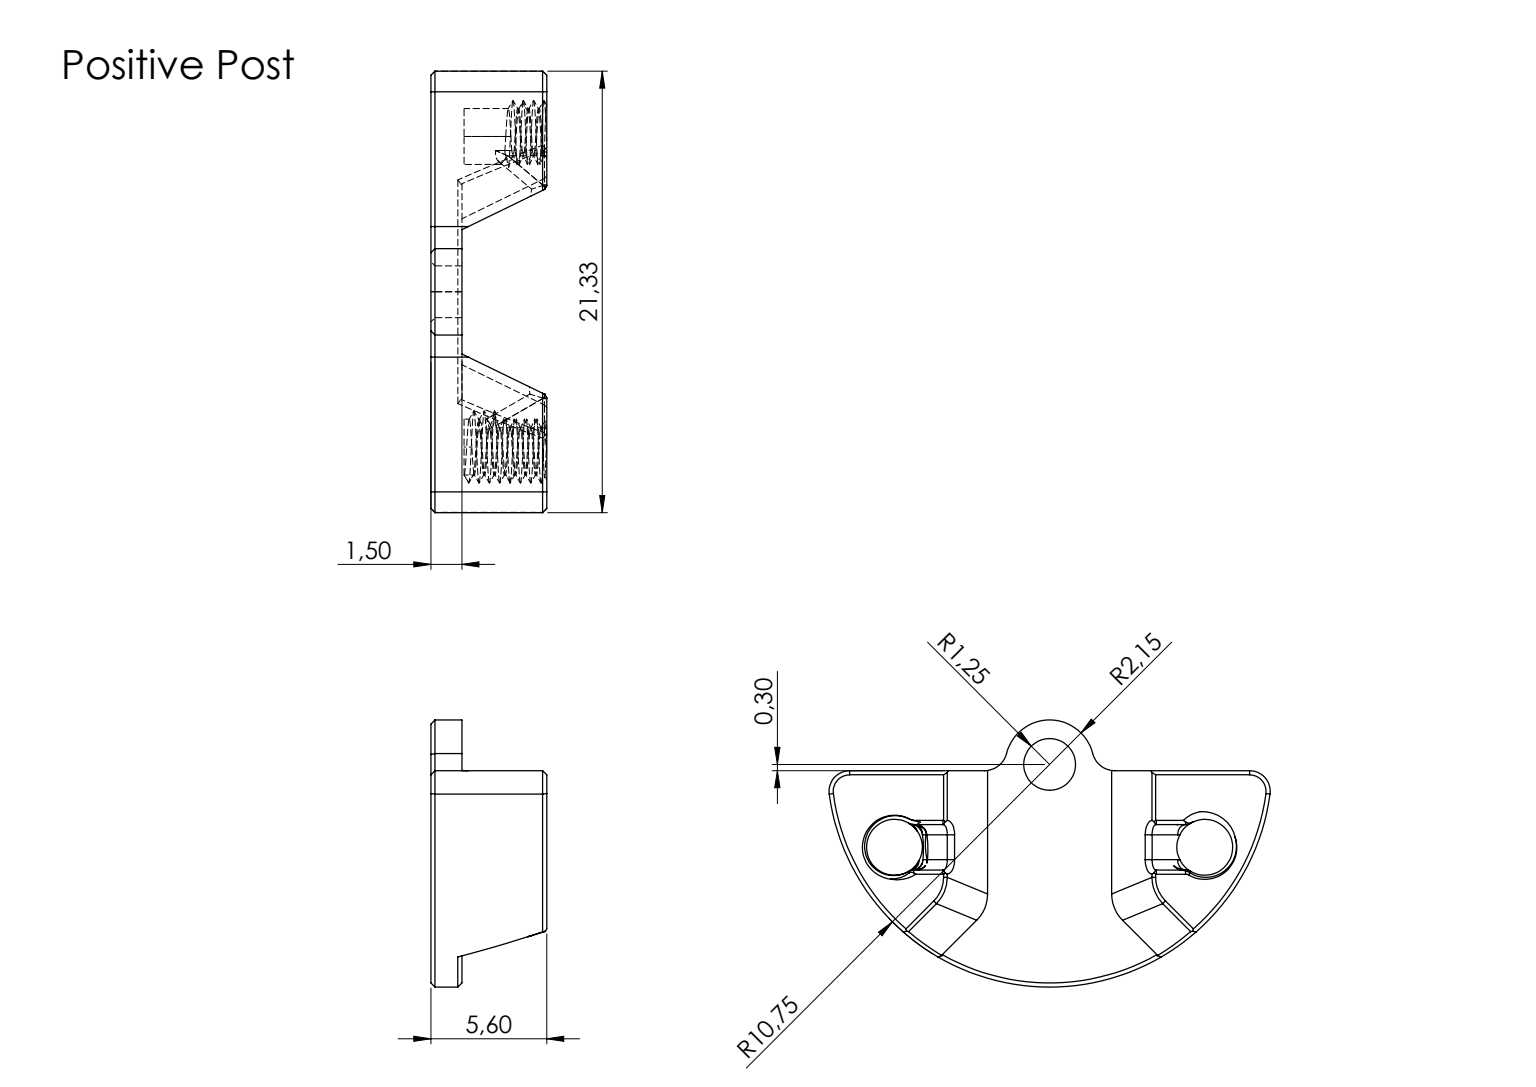
ISO-10303-21;
HEADER;
FILE_DESCRIPTION (('STEP AP214'),
    '1' );
FILE_NAME ('Positive Post.step',
    '2026-10-05T22:38:29',
    ( '' ),
    ( '' ),
    'SwSTEP 2.0',
    'SolidWorks 2020',
    '' );
FILE_SCHEMA (( 'AUTOMOTIVE_DESIGN' ));
ENDSEC;

DATA;
#3=DIRECTION ( 'NONE',  ( 1.000000000000000000, 0.000000000000000000, 0.000000000000000000 ) ) ;
#10=CARTESIAN_POINT ( 'NONE',  ( 9.778462793022999477, -5.743713977826000239, 7.748300060190000060 ) ) ;
#24=B_SPLINE_CURVE_WITH_KNOTS ( 'NONE', 3,
 ( #18393, #12452, #50546, #13155, #61715, #44967, #55102, #35164, #34485, #56132, #66271, #55449, #55796, #8240, #40068, #29927 ),
 .UNSPECIFIED., .F., .F.,
 ( 4, 2, 2, 1, 1, 2, 2, 2, 4 ),
 ( 0.000000000000000000, 0.2499999999999854561, 0.3749999999999792943, 0.4374999999999752420, 0.4687499999999756861, 0.4843749999999741873, 0.4999999999999726885, 0.7499999999999863443, 1.000000000000000000 ),
 .UNSPECIFIED. ) ;
#26=CARTESIAN_POINT ( 'NONE',  ( 9.239023565813489824, -2.669687318136871212, 7.269906695626100479 ) ) ;
#28=ORIENTED_EDGE ( 'NONE', *, *, #52791, .T. ) ;
#57=CARTESIAN_POINT ( 'NONE',  ( 8.674830025576039105, -2.649890579813208191, 7.499988935010342139 ) ) ;
#61=CARTESIAN_POINT ( 'NONE',  ( 9.794101180193951706, -2.685368189354502721, -7.853409369710684373 ) ) ;
#62=CYLINDRICAL_SURFACE ( 'NONE', #7615, 1.350000000000000089 ) ;
#73=EDGE_CURVE ( 'NONE', #54965, #29508, #17176, .T. ) ;
#82=ORIENTED_EDGE ( 'NONE', *, *, #59738, .T. ) ;
#88=CARTESIAN_POINT ( 'NONE',  ( 10.01835931248959888, -5.126777126172243015, -6.752018918849381102 ) ) ;
#100=EDGE_CURVE ( 'NONE', #6210, #57286, #54708, .T. ) ;
#109=CARTESIAN_POINT ( 'NONE',  ( 8.383148997457999130, -5.167567567567999731, 6.822293592207000934 ) ) ;
#113=CARTESIAN_POINT ( 'NONE',  ( 10.36950884864999978, -2.719121019997000399, -7.031782724641000293 ) ) ;
#114=ORIENTED_EDGE ( 'NONE', *, *, #34124, .T. ) ;
#117=CARTESIAN_POINT ( 'NONE',  ( 10.17905590578999941, -2.899999999999999911, 6.571291218949999902 ) ) ;
#118=LINE ( 'NONE', #6737, #27722 ) ;
#119=CARTESIAN_POINT ( 'NONE',  ( 8.635274708161395196, -3.045105040003566632, -6.545565613752198253 ) ) ;
#132=CARTESIAN_POINT ( 'NONE',  ( 7.905017292225999803, -2.916160783733999562, 6.437838678341997856 ) ) ;
#137=CARTESIAN_POINT ( 'NONE',  ( 9.215289122285998502, -4.861979632688999686, 8.938813901364000003 ) ) ;
#150=DIRECTION ( 'NONE',  ( -1.000000000000000000, 0.000000000000000000, 0.000000000000000000 ) ) ;
#157=DIRECTION ( 'NONE',  ( 0.000000000000000000, -0.1333333333333049930, -0.9910712498212376209 ) ) ;
#163=CARTESIAN_POINT ( 'NONE',  ( 10.00122642709000154, -2.274091010763000131, 7.851325450887000734 ) ) ;
#167=CARTESIAN_POINT ( 'NONE',  ( 9.085769353209000698, -2.821866379289000193, 6.127148604720000336 ) ) ;
#168=CARTESIAN_POINT ( 'NONE',  ( 10.32322128467999889, -3.399999874579999748, -4.621083553505000552 ) ) ;
#171=CIRCLE ( 'NONE', #66048, 0.5000000000000000000 ) ;
#176=CARTESIAN_POINT ( 'NONE',  ( 10.84168850528999961, -2.681008214828000114, 6.554752254946000889 ) ) ;
#181=CARTESIAN_POINT ( 'NONE',  ( 10.65229194037999960, -4.944342461481999962, -8.478476072358999360 ) ) ;
#183=CARTESIAN_POINT ( 'NONE',  ( 10.90000000536000080, -2.899999999941999640, -5.157071284930999866 ) ) ;
#191=CARTESIAN_POINT ( 'NONE',  ( 10.98768521492000083, -5.299565686336999981, -4.945211137252000455 ) ) ;
#200=CARTESIAN_POINT ( 'NONE',  ( 8.767881343006999728, -4.605543323398999966, -6.293427432547999523 ) ) ;
#202=CARTESIAN_POINT ( 'NONE',  ( 9.492702081557240490, -3.384517283567192170, -9.168413593352800817 ) ) ;
#208=CARTESIAN_POINT ( 'NONE',  ( 8.464254440379999522, -2.029110377978999846, 7.726994002375999315 ) ) ;
#212=VECTOR ( 'NONE', #46961, 1000.000000000000000 ) ;
#220=CARTESIAN_POINT ( 'NONE',  ( 11.09999999999999964, -6.593648099371000271, -5.598803483715999896 ) ) ;
#222=CARTESIAN_POINT ( 'NONE',  ( 8.764831853209999579, -5.808258301303999893, 7.446016267012000256 ) ) ;
#223=CARTESIAN_POINT ( 'NONE',  ( 8.898558059623999483, -5.146736128384000075, 6.597417125647000447 ) ) ;
#224=EDGE_CURVE ( 'NONE', #15130, #33857, #51488, .T. ) ;
#243=CARTESIAN_POINT ( 'NONE',  ( 8.449835681852293945, -2.260412657429408334, 7.498936987450196767 ) ) ;
#254=CARTESIAN_POINT ( 'NONE',  ( 9.865041550948088656, -2.650034642413194419, -7.500002425457253707 ) ) ;
#276=ORIENTED_EDGE ( 'NONE', *, *, #50855, .T. ) ;
#282=CARTESIAN_POINT ( 'NONE',  ( 10.98768521492000083, -5.299565686336999981, -4.945211137252000455 ) ) ;
#288=LINE ( 'NONE', #16362, #21275 ) ;
#296=ADVANCED_FACE ( 'NONE', ( #16756 ), #38788, .T. ) ;
#299=ORIENTED_EDGE ( 'NONE', *, *, #35075, .F. ) ;
#302=ADVANCED_FACE ( 'NONE', ( #33547 ), #22385, .T. ) ;
#309=AXIS2_PLACEMENT_3D ( 'NONE', #43572, #37285, #64184 ) ;
#320=CARTESIAN_POINT ( 'NONE',  ( 10.64872180584000105, -2.614778238704999591, 6.717279975758000177 ) ) ;
#321=CARTESIAN_POINT ( 'NONE',  ( 7.127706853208000126, -4.698358408974000255, 8.789434435623999065 ) ) ;
#326=CARTESIAN_POINT ( 'NONE',  ( 10.41025564679000048, -4.690690303276999984, -6.142863315966000215 ) ) ;
#327=CARTESIAN_POINT ( 'NONE',  ( 7.869532996850215234, -3.050177706499410668, 8.968124616582409558 ) ) ;
#329=CARTESIAN_POINT ( 'NONE',  ( 10.09196524370999981, -3.841385669346000231, 5.536421174581999338 ) ) ;
#350=CARTESIAN_POINT ( 'NONE',  ( 10.92717634842000152, -5.023656093247000243, 8.718039182945998888 ) ) ;
#357=ORIENTED_EDGE ( 'NONE', *, *, #14220, .T. ) ;
#374=CARTESIAN_POINT ( 'NONE',  ( 10.06844525594999951, -4.148609764890999863, 8.941457795715999524 ) ) ;
#414=CARTESIAN_POINT ( 'NONE',  ( 10.10735564678999943, -4.293585439421999439, -8.994200998147999115 ) ) ;
#436=CARTESIAN_POINT ( 'NONE',  ( 10.52663358771999924, -4.933730002636999679, -6.506004698255999585 ) ) ;
#438=VERTEX_POINT ( 'NONE', #64909 ) ;
#440=ORIENTED_EDGE ( 'NONE', *, *, #23269, .T. ) ;
#448=CARTESIAN_POINT ( 'NONE',  ( 10.29378083128999855, -3.483628580733000302, 6.176326635498999629 ) ) ;
#458=CARTESIAN_POINT ( 'NONE',  ( 10.36629943602999937, -5.852732332139999549, -7.568014220767000033 ) ) ;
#460=ORIENTED_EDGE ( 'NONE', *, *, #48777, .T. ) ;
#473=FACE_OUTER_BOUND ( 'NONE', #7500, .T. ) ;
#478=CARTESIAN_POINT ( 'NONE',  ( 9.318721994369999706, -2.755032632138999737, 8.795122807847999269 ) ) ;
#482=CARTESIAN_POINT ( 'NONE',  ( 9.504901164121001500, -3.934733502342999678, 5.704835336325999151 ) ) ;
#484=CARTESIAN_POINT ( 'NONE',  ( 9.780103651350286142, -2.899999999999999911, -6.453331515098025051 ) ) ;
#485=EDGE_CURVE ( 'NONE', #31101, #42061, #40421, .T. ) ;
#497=DIRECTION ( 'NONE',  ( 0.000000000000000000, -1.000000000000000000, 0.000000000000000000 ) ) ;
#505=ORIENTED_EDGE ( 'NONE', *, *, #36321, .F. ) ;
#507=CARTESIAN_POINT ( 'NONE',  ( 10.18909467608999897, -5.907859813488999912, 7.801539220053999912 ) ) ;
#518=VERTEX_POINT ( 'NONE', #61745 ) ;
#519=CARTESIAN_POINT ( 'NONE',  ( 9.104016254283999743, -5.045864843302999780, 8.527867871227000407 ) ) ;
#525=DIRECTION ( 'NONE',  ( 0.8987684456439055669, 0.000000000000000000, -0.4384236320214022764 ) ) ;
#532=VECTOR ( 'NONE', #65504, 1000.000000000000114 ) ;
#550=CARTESIAN_POINT ( 'NONE',  ( 10.90000000016000037, -2.832432432627000285, -6.822293591557000880 ) ) ;
#553=ORIENTED_EDGE ( 'NONE', *, *, #2355, .F. ) ;
#560=CARTESIAN_POINT ( 'NONE',  ( 7.705394353206999725, -3.245532552444000185, 8.949627348471000943 ) ) ;
#562=CARTESIAN_POINT ( 'NONE',  ( 7.851684996376999237, -4.710033951126000318, 6.351751497389999557 ) ) ;
#564=EDGE_CURVE ( 'NONE', #28902, #67173, #57226, .T. ) ;
#569=CARTESIAN_POINT ( 'NONE',  ( 11.09999999999999787, -5.533462193136272411, 7.009885406647008210 ) ) ;
#572=CARTESIAN_POINT ( 'NONE',  ( 9.406706853206999952, -3.705847642455000202, 9.096432253453999195 ) ) ;
#577=EDGE_CURVE ( 'NONE', #1541, #49491, #24675, .T. ) ;
#578=AXIS2_PLACEMENT_3D ( 'NONE', #48457, #16634, #59282 ) ;
#583=CARTESIAN_POINT ( 'NONE',  ( 9.470944094206000585, -5.100000000000000533, 6.571291218949999902 ) ) ;
#590=CARTESIAN_POINT ( 'NONE',  ( 8.432199894032919474, -2.299073235464944798, 7.876362923782135539 ) ) ;
#597=CARTESIAN_POINT ( 'NONE',  ( 7.732053840042254045, -3.067861470021875814, 6.507875357840980257 ) ) ;
#600=CARTESIAN_POINT ( 'NONE',  ( 10.28566371494471632, -5.375939593780930892, -6.377587382198379728 ) ) ;
#603=CARTESIAN_POINT ( 'NONE',  ( 9.004094043040858253, -2.621318921512024946, 6.376249635427098994 ) ) ;
#606=VERTEX_POINT ( 'NONE', #23655 ) ;
#611=CARTESIAN_POINT ( 'NONE',  ( 9.056630296855326279, -5.100000000000000533, 6.328714934328742103 ) ) ;
#612=ORIENTED_EDGE ( 'NONE', *, *, #21132, .T. ) ;
#616=LINE ( 'NONE', #53412, #60037 ) ;
#633=CARTESIAN_POINT ( 'NONE',  ( 10.25166529434999951, -3.418639857622999934, -8.733652610425998830 ) ) ;
#634=AXIS2_PLACEMENT_3D ( 'NONE', #59823, #28367, #23107 ) ;
#639=CARTESIAN_POINT ( 'NONE',  ( 10.85646369190719973, -5.100000000000000533, 6.665341197380437066 ) ) ;
#649=ORIENTED_EDGE ( 'NONE', *, *, #42532, .T. ) ;
#650=DIRECTION ( 'NONE',  ( 1.000000000000000000, 0.000000000000000000, -1.736057635220000058E-14 ) ) ;
#659=EDGE_CURVE ( 'NONE', #35912, #16031, #57879, .T. ) ;
#660=VECTOR ( 'NONE', #36324, 1000.000000000000000 ) ;
#664=VERTEX_POINT ( 'NONE', #9284 ) ;
#668=CARTESIAN_POINT ( 'NONE',  ( 10.98286725694000054, -3.998514182530999772, 9.091066422484001208 ) ) ;
#669=CARTESIAN_POINT ( 'NONE',  ( 7.833769353207999941, -2.583664704444999849, 6.684748541034000624 ) ) ;
#671=CARTESIAN_POINT ( 'NONE',  ( 8.205992358809998777, -3.399999999999999911, 6.138278517058000538 ) ) ;
#673=CARTESIAN_POINT ( 'NONE',  ( 10.29666814679000097, -2.755511079787000384, -6.622434938646999392 ) ) ;
#674=CARTESIAN_POINT ( 'NONE',  ( 7.771548168530000744, -5.066493862386956870, 8.873801325387214334 ) ) ;
#675=CARTESIAN_POINT ( 'NONE',  ( 10.58844302970999962, -3.754658547780000521, 5.545362468768000319 ) ) ;
#683=VERTEX_POINT ( 'NONE', #46710 ) ;
#691=CARTESIAN_POINT ( 'NONE',  ( 8.946004440379999423, -5.458705123429999695, 7.456451825584000659 ) ) ;
#701=EDGE_CURVE ( 'NONE', #59694, #61758, #40523, .T. ) ;
#705=ADVANCED_FACE ( 'NONE', ( #26415 ), #52981, .T. ) ;
#706=EDGE_CURVE ( 'NONE', #1057, #51230, #41392, .T. ) ;
#723=CARTESIAN_POINT ( 'NONE',  ( 10.31668414895000119, -3.819528725844000494, 6.062183754159999438 ) ) ;
#744=EDGE_CURVE ( 'NONE', #12348, #53120, #12170, .T. ) ;
#751=VECTOR ( 'NONE', #15220, 1000.000000000000000 ) ;
#760=CARTESIAN_POINT ( 'NONE',  ( 10.09249435321000021, -2.841617206345000035, -8.724656239052000828 ) ) ;
#765=DIRECTION ( 'NONE',  ( -0.7660444431190119863, -5.852582307674940185E-12, -0.6427876096864989508 ) ) ;
#766=ORIENTED_EDGE ( 'NONE', *, *, #53572, .F. ) ;
#782=CARTESIAN_POINT ( 'NONE',  ( 10.43283788151999936, -3.279327064383000145, -9.029275888523999427 ) ) ;
#795=CARTESIAN_POINT ( 'NONE',  ( 9.423521818475000700, -4.993993578306000103, 8.578110568283999982 ) ) ;
#808=CARTESIAN_POINT ( 'NONE',  ( 10.19715077290999972, -4.982624057277000418, -6.124316828241999744 ) ) ;
#825=CARTESIAN_POINT ( 'NONE',  ( 10.02990552045999983, -2.506467134554999809, 6.215414506835998942 ) ) ;
#829=CARTESIAN_POINT ( 'NONE',  ( 9.442841440870999747, -2.691258483914000355, 6.269525829285999663 ) ) ;
#844=CARTESIAN_POINT ( 'NONE',  ( 7.610826510211253115, -3.823093646280199653, 8.848653938445639966 ) ) ;
#847=CARTESIAN_POINT ( 'NONE',  ( 5.699999999836000697, -1.433333331105999919, -10.65401593570999950 ) ) ;
#849=CARTESIAN_POINT ( 'NONE',  ( 10.84920446231350155, -2.899999999999999911, -6.662590550579920112 ) ) ;
#852=VERTEX_POINT ( 'NONE', #14552 ) ;
#859=EDGE_LOOP ( 'NONE', ( #2403, #13429, #58338, #59065 ) ) ;
#864=CARTESIAN_POINT ( 'NONE',  ( 9.911640687501567015, -2.873222873816665413, -6.752018918868491149 ) ) ;
#867=CARTESIAN_POINT ( 'NONE',  ( 10.68904248846000016, -2.568964727443000307, 7.728094434513999467 ) ) ;
#870=EDGE_CURVE ( 'NONE', #57810, #22321, #17292, .T. ) ;
#873=VERTEX_POINT ( 'NONE', #6798 ) ;
#886=CARTESIAN_POINT ( 'NONE',  ( 9.327383005933997495, -3.946161398296482048, 9.238824392371451921 ) ) ;
#895=CARTESIAN_POINT ( 'NONE',  ( 9.305875415870998424, -4.945293979885000191, 9.077881967919999795 ) ) ;
#897=CARTESIAN_POINT ( 'NONE',  ( 7.717206996518667594, -2.839603352907888123, 6.809939372030577864 ) ) ;
#899=EDGE_LOOP ( 'NONE', ( #66916, #36286, #32294, #9509 ) ) ;
#900=ORIENTED_EDGE ( 'NONE', *, *, #41275, .F. ) ;
#904=CARTESIAN_POINT ( 'NONE',  ( 9.199609130449999839, -2.551382302226000487, 7.536606162076999738 ) ) ;
#906=CARTESIAN_POINT ( 'NONE',  ( 8.347269353210000631, -2.741638482234999952, 6.457327039244000311 ) ) ;
#915=CARTESIAN_POINT ( 'NONE',  ( 11.07925595036916633, -5.279255950369167394, 6.503434303641999925 ) ) ;
#920=CARTESIAN_POINT ( 'NONE',  ( 8.834370559623998531, -4.141908960411000429, 6.047561724438000219 ) ) ;
#938=CARTESIAN_POINT ( 'NONE',  ( 8.447423826815846581, -2.260942181570626541, 7.552185937853629127 ) ) ;
#948=CARTESIAN_POINT ( 'NONE',  ( 10.77164068750950143, -2.873222873834234914, 6.752018918838221140 ) ) ;
#949=CARTESIAN_POINT ( 'NONE',  ( 11.04783424078000031, -2.764605797469000148, 5.041477660832000218 ) ) ;
#953=EDGE_LOOP ( 'NONE', ( #20511, #17436, #26609 ) ) ;
#956=EDGE_CURVE ( 'NONE', #9091, #38701, #48076, .T. ) ;
#980=CARTESIAN_POINT ( 'NONE',  ( 10.77434462036999818, -4.612888200890999713, -8.898797372219998891 ) ) ;
#985=ORIENTED_EDGE ( 'NONE', *, *, #39002, .F. ) ;
#996=DIRECTION ( 'NONE',  ( -0.7071067811865474617, -0.7071067811865474617, 1.013775886743067205E-08 ) ) ;
#998=FACE_OUTER_BOUND ( 'NONE', #6504, .T. ) ;
#1004=CARTESIAN_POINT ( 'NONE',  ( 10.63789391302397647, -4.829717262113836895, -8.579596796881972409 ) ) ;
#1017=CARTESIAN_POINT ( 'NONE',  ( 10.18239901426000138, -2.607725299334000102, 7.783410967795999724 ) ) ;
#1018=CARTESIAN_POINT ( 'NONE',  ( 8.770183059623999355, -3.049610585291000042, 6.392533570808999421 ) ) ;
#1022=CARTESIAN_POINT ( 'NONE',  ( 11.01605564679000082, -5.482859940357000639, -7.846409404949000077 ) ) ;
#1023=CARTESIAN_POINT ( 'NONE',  ( 7.767789809242127141, -5.129599579532937881, 8.822844411293367273 ) ) ;
#1026=ORIENTED_EDGE ( 'NONE', *, *, #43279, .F. ) ;
#1040=DIRECTION ( 'NONE',  ( -0.7660444431190069903, 0.000000000000000000, -0.6427876096865049460 ) ) ;
#1043=CARTESIAN_POINT ( 'NONE',  ( 9.395316940379000670, -5.146736128384000075, 6.597417125647000447 ) ) ;
#1046=CARTESIAN_POINT ( 'NONE',  ( 10.00068357938802954, -3.239576832587917732, -9.078134629932138822 ) ) ;
#1057=VERTEX_POINT ( 'NONE', #21414 ) ;
#1064=LINE ( 'NONE', #22718, #65137 ) ;
#1072=CARTESIAN_POINT ( 'NONE',  ( 10.13050497920000126, -3.092053006542000215, 8.629388195475000245 ) ) ;
#1083=PLANE ( 'NONE',  #43091 ) ;
#1110=CARTESIAN_POINT ( 'NONE',  ( 10.16821935321000048, -2.330398934821000356, -7.267462182607999921 ) ) ;
#1111=CARTESIAN_POINT ( 'NONE',  ( 11.00000000000000000, -0.4000000000000000222, -7.331472342878999626 ) ) ;
#1114=DIRECTION ( 'NONE',  ( 0.4384236320214023319, 0.000000000000000000, -0.8987684456439056779 ) ) ;
#1117=ORIENTED_EDGE ( 'NONE', *, *, #15075, .T. ) ;
#1128=CARTESIAN_POINT ( 'NONE',  ( 10.98277446826000059, -2.518728855032000169, -8.314788219120000434 ) ) ;
#1132=B_SPLINE_CURVE_WITH_KNOTS ( 'NONE', 3,
 ( #7572, #7229, #2671, #65944 ),
 .UNSPECIFIED., .F., .F.,
 ( 4, 4 ),
 ( 0.000000000000000000, 1.000000000000000000 ),
 .UNSPECIFIED. ) ;
#1133=ORIENTED_EDGE ( 'NONE', *, *, #68920, .T. ) ;
#1136=ORIENTED_EDGE ( 'NONE', *, *, #47046, .F. ) ;
#1138=CARTESIAN_POINT ( 'NONE',  ( 10.85067755245999876, -5.068636324353000155, 5.153848641568999689 ) ) ;
#1150=DIRECTION ( 'NONE',  ( 1.000000000000000000, 0.000000000000000000, 0.000000000000000000 ) ) ;
#1155=CARTESIAN_POINT ( 'NONE',  ( 9.973487588364999823, -4.344961837988999598, -9.321582626371998970 ) ) ;
#1156=ORIENTED_EDGE ( 'NONE', *, *, #49731, .F. ) ;
#1158=CARTESIAN_POINT ( 'NONE',  ( 8.218666589540001510, -2.895314275791000203, 6.639800878566000542 ) ) ;
#1167=ORIENTED_EDGE ( 'NONE', *, *, #53745, .T. ) ;
#1170=CARTESIAN_POINT ( 'NONE',  ( 9.967845797207999681, -2.034786297409000078, 7.636877353231999344 ) ) ;
#1174=CARTESIAN_POINT ( 'NONE',  ( 11.02786767503999954, -5.596230239120999705, 7.209501483790000442 ) ) ;
#1185=CARTESIAN_POINT ( 'NONE',  ( 8.629721738021999045, -2.812225201737000635, -6.860033716225003353 ) ) ;
#1193=DIRECTION ( 'NONE',  ( 1.000000000000000000, 0.000000000000000000, 0.000000000000000000 ) ) ;
#1198=CARTESIAN_POINT ( 'NONE',  ( 7.961731591766580074, -5.351349901897480166, 7.263035046629693348 ) ) ;
#1205=CARTESIAN_POINT ( 'NONE',  ( 9.884624721933931824, -2.899999999999999911, 6.445686799102332110 ) ) ;
#1206=CARTESIAN_POINT ( 'NONE',  ( 8.545870559624999530, -3.856773448568000084, 5.521258396339000285 ) ) ;
#1213=ORIENTED_EDGE ( 'NONE', *, *, #58230, .F. ) ;
#1218=CARTESIAN_POINT ( 'NONE',  ( 11.35905860703999970, -2.719090443614000208, -7.157642341559000698 ) ) ;
#1237=CARTESIAN_POINT ( 'NONE',  ( 9.409308287954999628, -2.634700736117999931, 8.920302460802998823 ) ) ;
#1247=CARTESIAN_POINT ( 'NONE',  ( 8.796581853210000190, -2.368260286481999710, 7.410200011629000549 ) ) ;
#1251=PLANE ( 'NONE',  #9581 ) ;
#1257=ORIENTED_EDGE ( 'NONE', *, *, #60141, .F. ) ;
#1258=CARTESIAN_POINT ( 'NONE',  ( 8.353308059623998361, -2.800111029801999774, 9.079936276749000612 ) ) ;
#1261=EDGE_CURVE ( 'NONE', #64636, #25798, #1264, .T. ) ;
#1264=B_SPLINE_CURVE_WITH_KNOTS ( 'NONE', 3,
 ( #28756, #50411, #13017, #2177, #23492 ),
 .UNSPECIFIED., .F., .F.,
 ( 4, 1, 4 ),
 ( 0.000000000000000000, 0.5000000000000000000, 1.000000000000000000 ),
 .UNSPECIFIED. ) ;
#1278=EDGE_CURVE ( 'NONE', #11696, #53746, #2872, .T. ) ;
#1279=CARTESIAN_POINT ( 'NONE',  ( 8.377276386243467599, -2.937594683383006888, 8.878994193280906444 ) ) ;
#1282=VERTEX_POINT ( 'NONE', #24530 ) ;
#1283=LINE ( 'NONE', #33448, #6506 ) ;
#1284=CARTESIAN_POINT ( 'NONE',  ( 9.532671748231999587, -4.663050389319001177, 8.669823109968998409 ) ) ;
#1286=ADVANCED_FACE ( 'NONE', ( #29799 ), #3878, .T. ) ;
#1292=FILL_AREA_STYLE ('',( #64556 ) ) ;
#1296=ORIENTED_EDGE ( 'NONE', *, *, #59364, .F. ) ;
#1316=CARTESIAN_POINT ( 'NONE',  ( 10.65650106607000147, -5.448187878199999723, -7.015213573792999036 ) ) ;
#1322=DIRECTION ( 'NONE',  ( 0.4682208595142289265, -0.4682208595142289265, -0.7493586947727458591 ) ) ;
#1325=CARTESIAN_POINT ( 'NONE',  ( 9.615066448851507630, -5.349942704376990044, -7.499996115248991124 ) ) ;
#1332=CARTESIAN_POINT ( 'NONE',  ( 10.90000000000000036, -8.091320520030999219, -7.077643127633000297 ) ) ;
#1334=CARTESIAN_POINT ( 'NONE',  ( 8.207504440379000954, -5.944572422272999646, 7.106845737860000511 ) ) ;
#1336=ADVANCED_FACE ( 'NONE', ( #69147 ), #52485, .F. ) ;
#1346=CARTESIAN_POINT ( 'NONE',  ( 10.67905590578999941, -2.899999999999999911, 6.571291218949999902 ) ) ;
#1353=CARTESIAN_POINT ( 'NONE',  ( 9.534903635507999908, -3.030945724184999968, 8.761987396837000119 ) ) ;
#1354=CARTESIAN_POINT ( 'NONE',  ( 8.641808059624999316, -2.933824946949000090, 8.496487880080000110 ) ) ;
#1356=CARTESIAN_POINT ( 'NONE',  ( 8.191498616105999275, -3.399962740672999750, 6.146646623957999545 ) ) ;
#1359=CARTESIAN_POINT ( 'NONE',  ( 10.62256935321000029, -2.471463903746000224, -8.210787855397999380 ) ) ;
#1360=CARTESIAN_POINT ( 'NONE',  ( 7.755402176232501610, -5.324011115352642598, 8.627901512810892015 ) ) ;
#1361=CARTESIAN_POINT ( 'NONE',  ( 9.967845797207999681, -2.034786297409000078, 7.636877353231999344 ) ) ;
#1363=ORIENTED_EDGE ( 'NONE', *, *, #20264, .F. ) ;
#1364=VECTOR ( 'NONE', #19089, 1000.000000000000114 ) ;
#1382=ORIENTED_EDGE ( 'NONE', *, *, #4865, .F. ) ;
#1417=B_SPLINE_CURVE_WITH_KNOTS ( 'NONE', 3,
 ( #33485, #17394, #59349, #2010 ),
 .UNSPECIFIED., .F., .F.,
 ( 4, 4 ),
 ( 0.8745775486650082531, 1.000000000000000000 ),
 .UNSPECIFIED. ) ;
#1449=ADVANCED_FACE ( 'NONE', ( #9991 ), #58479, .F. ) ;
#1454=CARTESIAN_POINT ( 'NONE',  ( 11.16750564679000135, -3.188702545307000147, -8.788667016604001958 ) ) ;
#1472=CARTESIAN_POINT ( 'NONE',  ( 11.15192313136999935, -2.359310578948000003, -6.636692315558000210 ) ) ;
#1479=ORIENTED_EDGE ( 'NONE', *, *, #21563, .T. ) ;
#1482=CARTESIAN_POINT ( 'NONE',  ( 10.32769335537625111, -3.168316061382061566, 4.960153499376385611 ) ) ;
#1487=CARTESIAN_POINT ( 'NONE',  ( 9.569799020577001158, -4.064052785562999759, 8.919253808370999792 ) ) ;
#1499=CARTESIAN_POINT ( 'NONE',  ( 10.43283788151999936, -3.279327064383000145, -9.029275888523999427 ) ) ;
#1503=CARTESIAN_POINT ( 'NONE',  ( 5.000000000000000000, -0.2999999999999999889, -6.709430130811999682 ) ) ;
#1509=CARTESIAN_POINT ( 'NONE',  ( 10.32941944301999904, -3.080527974829000204, 4.567383801607999949 ) ) ;
#1514=CARTESIAN_POINT ( 'NONE',  ( 9.442841440870999747, -2.691258483914000355, 6.269525829285999663 ) ) ;
#1517=CARTESIAN_POINT ( 'NONE',  ( 10.15903154954000165, -4.166415630773999901, 9.114167874391000623 ) ) ;
#1518=CARTESIAN_POINT ( 'NONE',  ( 10.90453766415000025, -2.900310535872000273, -5.130381900875999435 ) ) ;
#1525=CARTESIAN_POINT ( 'NONE',  ( 8.666062080003996471, -2.822439486461001401, -6.845494810064998603 ) ) ;
#1534=CARTESIAN_POINT ( 'NONE',  ( 7.548482128266483571, -4.828745666966125505, 8.579002673691162428 ) ) ;
#1541=VERTEX_POINT ( 'NONE', #16267 ) ;
#1546=CARTESIAN_POINT ( 'NONE',  ( 8.866808059624998961, -2.550589632307000088, 8.854674225901000284 ) ) ;
#1552=ORIENTED_EDGE ( 'NONE', *, *, #16777, .F. ) ;
#1566=EDGE_CURVE ( 'NONE', #852, #67663, #47083, .T. ) ;
#1567=ADVANCED_FACE ( 'NONE', ( #23930 ), #45266, .F. ) ;
#1570=ADVANCED_FACE ( 'NONE', ( #39324 ), #59792, .F. ) ;
#1588=CARTESIAN_POINT ( 'NONE',  ( 10.75110221171000013, -2.822135527917999820, 6.655890318096999714 ) ) ;
#1595=CARTESIAN_POINT ( 'NONE',  ( 8.851049249631991245, -5.136676904523000076, -6.770570396461005558 ) ) ;
#1600=CARTESIAN_POINT ( 'NONE',  ( 10.31498017945871126, -2.650031506806249659, -7.499998780888571304 ) ) ;
#1631=CARTESIAN_POINT ( 'NONE',  ( 9.769471092180999960, -5.100000000000000533, -6.152188490330000370 ) ) ;
#1639=DIRECTION ( 'NONE',  ( -0.9999999999999997780, 1.340566441529999910E-09, -2.196397022486999685E-08 ) ) ;
#1640=LINE ( 'NONE', #12475, #26186 ) ;
#1647=ORIENTED_EDGE ( 'NONE', *, *, #46056, .F. ) ;
#1664=CARTESIAN_POINT ( 'NONE',  ( 10.85290698989999925, -3.170384785323999921, -8.782188229854000383 ) ) ;
#1683=VERTEX_POINT ( 'NONE', #31586 ) ;
#1684=CARTESIAN_POINT ( 'NONE',  ( 7.886566940378000545, -3.084082018960999871, 9.259837032825000591 ) ) ;
#1685=CARTESIAN_POINT ( 'NONE',  ( 9.754318513071000396, -2.462132291381999849, -7.373611177161000008 ) ) ;
#1690=CARTESIAN_POINT ( 'NONE',  ( 10.58580560302255336, -5.314991280552569641, -7.853445763305400007 ) ) ;
#1700=CARTESIAN_POINT ( 'NONE',  ( 11.09424907396999949, -2.431867116603999790, 7.769513708858000633 ) ) ;
#1705=CARTESIAN_POINT ( 'NONE',  ( 10.09249435321000021, -2.841617206345000035, -8.724656239052000828 ) ) ;
#1706=CARTESIAN_POINT ( 'NONE',  ( 8.093175425641877752, -4.412936408959972745, 5.810561453377049546 ) ) ;
#1724=CARTESIAN_POINT ( 'NONE',  ( 27.64127793187000037, -2.399999999999999911, -6.571291218949999902 ) ) ;
#1730=CARTESIAN_POINT ( 'NONE',  ( 11.06205805961999999, -2.154403720901000518, -7.605897512385999981 ) ) ;
#1736=PLANE ( 'NONE',  #51995 ) ;
#1744=DIRECTION ( 'NONE',  ( -1.000000000000000000, 7.105427357347999651E-14, -1.243449787536000124E-13 ) ) ;
#1788=EDGE_LOOP ( 'NONE', ( #20717, #67196, #12483, #48430, #46677, #49089, #64017, #27105, #14391, #50804, #27207, #17189, #26426, #33045, #29344, #30815, #67646, #42917, #24260, #20176, #39518, #17278, #7910, #28187, #35313, #8859 ) ) ;
#1794=ORIENTED_EDGE ( 'NONE', *, *, #42391, .F. ) ;
#1796=DIRECTION ( 'NONE',  ( 0.8987684456439055669, 0.000000000000000000, 0.4384236320214022764 ) ) ;
#1802=CARTESIAN_POINT ( 'NONE',  ( 11.01605564679000082, -5.482859940357000639, -7.846409404949000077 ) ) ;
#1820=CARTESIAN_POINT ( 'NONE',  ( 10.58996262057999971, -2.876743158681999812, -6.236533224899999617 ) ) ;
#1825=B_SPLINE_CURVE_WITH_KNOTS ( 'NONE', 3,
 ( #51317, #24748, #46073, #67379 ),
 .UNSPECIFIED., .F., .F.,
 ( 4, 4 ),
 ( 0.000000000000000000, 1.000000000000000000 ),
 .UNSPECIFIED. ) ;
#1830=CARTESIAN_POINT ( 'NONE',  ( 10.42019978113000001, -4.954695572289999461, 4.899689062414000595 ) ) ;
#1834=CARTESIAN_POINT ( 'NONE',  ( 10.25888544622000076, -4.512389816463000081, 5.993697694029000544 ) ) ;
#1848=CARTESIAN_POINT ( 'NONE',  ( 10.90421209872000041, -3.863781031729999871, -9.185081053980001187 ) ) ;
#1852=CARTESIAN_POINT ( 'NONE',  ( 9.614739029020999084, -5.020908168068000776, -6.342951604057000203 ) ) ;
#1861=VECTOR ( 'NONE', #37919, 1000.000000000000000 ) ;
#1864=CARTESIAN_POINT ( 'NONE',  ( 10.15402496696000156, -5.267980706381999667, 5.992344456606999437 ) ) ;
#1867=CARTESIAN_POINT ( 'NONE',  ( 9.447848023450999833, -5.447470167531999863, 7.431328114251999573 ) ) ;
#1868=CIRCLE ( 'NONE', #42088, 1.549999999999999156 ) ;
#1883=CARTESIAN_POINT ( 'NONE',  ( 5.700000000000000178, 0.000000000000000000, 0.000000000000000000 ) ) ;
#1904=FACE_OUTER_BOUND ( 'NONE', #31398, .T. ) ;
#1907=CARTESIAN_POINT ( 'NONE',  ( 9.820206362952999868, -3.883324525498000224, 6.055606607331999847 ) ) ;
#1923=CARTESIAN_POINT ( 'NONE',  ( 9.456118062523774626, -2.255366135290077345, 7.362790452840693334 ) ) ;
#1937=CIRCLE ( 'NONE', #20890, 10.75000000000000533 ) ;
#1941=CARTESIAN_POINT ( 'NONE',  ( 10.06844525594999951, -4.148609764890999863, 8.941457795715999524 ) ) ;
#1943=CARTESIAN_POINT ( 'NONE',  ( 8.192495559623999668, -2.550228841911000188, 7.666975032000999946 ) ) ;
#1947=CARTESIAN_POINT ( 'NONE',  ( 9.264867054676999558, -5.097279491198996482, -6.598518734304002820 ) ) ;
#1951=CARTESIAN_POINT ( 'NONE',  ( 11.09999999999999964, -5.489445176276809057, 6.853104147731436946 ) ) ;
#1964=ADVANCED_FACE ( 'NONE', ( #22378 ), #22582, .T. ) ;
#1969=VECTOR ( 'NONE', #19314, 1000.000000000000114 ) ;
#1971=VERTEX_POINT ( 'NONE', #17131 ) ;
#1976=CARTESIAN_POINT ( 'NONE',  ( 11.09999999999999964, -4.000000000000000000, 7.500000000000000000 ) ) ;
#1982=CARTESIAN_POINT ( 'NONE',  ( 9.487500104632182740, -4.950335429809691767, 8.458601829922910653 ) ) ;
#1988=LINE ( 'NONE', #3350, #1364 ) ;
#1989=CARTESIAN_POINT ( 'NONE',  ( 8.769549439917666334, -5.100000000000000533, 6.459823844766666490 ) ) ;
#1997=CARTESIAN_POINT ( 'NONE',  ( 10.67500447327561908, -2.650284540010996004, 7.500001951671615430 ) ) ;
#2003=AXIS2_PLACEMENT_3D ( 'NONE', #35024, #19268, #45510 ) ;
#2008=EDGE_LOOP ( 'NONE', ( #58991, #6494, #23721, #13922 ) ) ;
#2010=CARTESIAN_POINT ( 'NONE',  ( 8.766851002546001581, -2.832432432432000269, 6.822293592207000934 ) ) ;
#2012=CARTESIAN_POINT ( 'NONE',  ( 9.870877370727999534, -2.904359058094999835, -8.563874348197000330 ) ) ;
#2014=AXIS2_PLACEMENT_3D ( 'NONE', #36960, #10377, #32406 ) ;
#2024=CARTESIAN_POINT ( 'NONE',  ( 10.82336322479176083, -2.820284244472506252, -8.179952785015981220 ) ) ;
#2025=DIRECTION ( 'NONE',  ( 0.8660254001570034665, -4.588230081904017516E-12, -0.5000000062829018654 ) ) ;
#2031=B_SPLINE_CURVE_WITH_KNOTS ( 'NONE', 3,
 ( #28093, #50111, #59898, #43487, #23532, #22837, #23188, #12006, #49067, #44183, #44534, #7107, #66178, #11310, #28444, #32647, #53959, #22488, #43831, #60595, #6062, #65482, #17606, #65130 ),
 .UNSPECIFIED., .F., .F.,
 ( 4, 2, 2, 2, 2, 2, 2, 2, 2, 2, 2, 4 ),
 ( 0.000000000000000000, 0.06250000000000027756, 0.1250000000000005551, 0.1875000000000008327, 0.2500000000000011102, 0.3750000000000009992, 0.5000000000000008882, 0.6250000000000007772, 0.7500000000000006661, 0.8750000000000005551, 0.9375000000000002220, 1.000000000000000000 ),
 .UNSPECIFIED. ) ;
#2036=CARTESIAN_POINT ( 'NONE',  ( 7.346668146792000087, -2.374041291348000016, 8.293390875797999939 ) ) ;
#2037=CARTESIAN_POINT ( 'NONE',  ( 10.09166489801000033, -4.565692099013000771, -8.879633571423999783 ) ) ;
#2041=VERTEX_POINT ( 'NONE', #60140 ) ;
#2052=CARTESIAN_POINT ( 'NONE',  ( 9.555699158955999195, -2.440755924888999839, 6.680881588809999272 ) ) ;
#2058=CARTESIAN_POINT ( 'NONE',  ( 10.22094314679000071, -2.563075248996000255, -8.004105227364998854 ) ) ;
#2059=CARTESIAN_POINT ( 'NONE',  ( 8.059803797423384708, -3.670685108766681193, 5.791771361350072311 ) ) ;
#2060=CARTESIAN_POINT ( 'NONE',  ( 10.77962878203999963, -2.397503436487000261, 7.755423856053000442 ) ) ;
#2068=VERTEX_POINT ( 'NONE', #44069 ) ;
#2070=AXIS2_PLACEMENT_3D ( 'NONE', #15851, #52921, #10265 ) ;
#2071=CARTESIAN_POINT ( 'NONE',  ( 8.188938565157450000, -2.652235273545322070, 7.263344527950025942 ) ) ;
#2080=VERTEX_POINT ( 'NONE', #23072 ) ;
#2081=CARTESIAN_POINT ( 'NONE',  ( 7.464688980125999684, -4.351670788182000038, 8.977200644264000218 ) ) ;
#2086=CARTESIAN_POINT ( 'NONE',  ( 10.56984555961999916, -2.152868447761999704, -7.425101130468999777 ) ) ;
#2097=B_SPLINE_CURVE_WITH_KNOTS ( 'NONE', 3,
 ( #6932, #61798, #61458, #19147 ),
 .UNSPECIFIED., .F., .F.,
 ( 4, 4 ),
 ( 0.000000000000000000, 1.000000000000000000 ),
 .UNSPECIFIED. ) ;
#2123=CARTESIAN_POINT ( 'NONE',  ( 8.753441940380000119, -2.876278577719999952, 6.568889245344999850 ) ) ;
#2127=ORIENTED_EDGE ( 'NONE', *, *, #18147, .T. ) ;
#2151=B_SPLINE_CURVE_WITH_KNOTS ( 'NONE', 3,
 ( #29955, #3013, #8264, #35529 ),
 .UNSPECIFIED., .F., .F.,
 ( 4, 4 ),
 ( 0.000000000000000000, 1.000000000000000000 ),
 .UNSPECIFIED. ) ;
#2152=CARTESIAN_POINT ( 'NONE',  ( 9.662398456552571346, -2.649938674317672049, 7.712117850346626113 ) ) ;
#2153=CARTESIAN_POINT ( 'NONE',  ( 10.17270027370999941, -4.650151116117000605, -8.655526539784000661 ) ) ;
#2154=CARTESIAN_POINT ( 'NONE',  ( 10.99385884816407888, -6.138431480138868856, 5.072166845528967016 ) ) ;
#2168=CARTESIAN_POINT ( 'NONE',  ( 10.98768491210000064, -8.067891622241001315, 6.818837029638999958 ) ) ;
#2169=CARTESIAN_POINT ( 'NONE',  ( 11.09999999999999964, -4.000000000000000000, -7.500000000000000000 ) ) ;
#2173=CARTESIAN_POINT ( 'NONE',  ( 11.11264194660999927, -2.146089039267000231, -7.517188649391000510 ) ) ;
#2174=DIRECTION ( 'NONE',  ( -0.7071067811865474617, 0.7071067811865474617, 1.196435574830078999E-09 ) ) ;
#2175=CARTESIAN_POINT ( 'NONE',  ( 10.69836233406524606, -2.942435227297377498, -5.063088263990971782 ) ) ;
#2177=CARTESIAN_POINT ( 'NONE',  ( 10.99828335019000214, -2.710349843344999954, -4.962170859942000689 ) ) ;
#2179=CARTESIAN_POINT ( 'NONE',  ( 10.27122572358000063, -4.578406546873999616, 4.846540991051999647 ) ) ;
#2180=DIRECTION ( 'NONE',  ( 0.000000000000000000, -0.8648648648648720183, -0.5020047465136826537 ) ) ;
#2184=CARTESIAN_POINT ( 'NONE',  ( 10.64872180584000105, -2.614778238704999591, 6.717279975758000177 ) ) ;
#2185=ORIENTED_EDGE ( 'NONE', *, *, #42796, .F. ) ;
#2191=AXIS2_PLACEMENT_3D ( 'NONE', #67985, #150, #5047 ) ;
#2194=B_SPLINE_CURVE_WITH_KNOTS ( 'NONE', 3,
 ( #31715, #22243, #53035, #49160, #15629, #43581, #54060, #26468, #27157, #21214 ),
 .UNSPECIFIED., .F., .F.,
 ( 4, 2, 2, 2, 4 ),
 ( 0.000000000000000000, 0.08334174874897928853, 0.1666834974979585771, 0.2500252462469378933, 0.3333669949959171541 ),
 .UNSPECIFIED. ) ;
#2201=CARTESIAN_POINT ( 'NONE',  ( 0.000000000000000000, -2.899999999999999911, 7.500000000000000000 ) ) ;
#2203=CARTESIAN_POINT ( 'NONE',  ( 9.658740731405000446, -5.476443305113000370, -7.051545409824000465 ) ) ;
#2205=LINE ( 'NONE', #59883, #62835 ) ;
#2213=CARTESIAN_POINT ( 'NONE',  ( 11.15982711745999900, -5.578228817597000955, 8.067792329320999656 ) ) ;
#2216=CARTESIAN_POINT ( 'NONE',  ( 9.124702828701000357, -4.778665285493000070, 8.799745834808000211 ) ) ;
#2226=DIRECTION ( 'NONE',  ( -1.000000000000000000, 0.000000000000000000, 0.000000000000000000 ) ) ;
#2229=CARTESIAN_POINT ( 'NONE',  ( 9.568154437819998748, -5.318469253323000245, -7.099528416287999910 ) ) ;
#2230=CARTESIAN_POINT ( 'NONE',  ( 10.15293113568789352, -5.100000000000000533, -6.444141223401128826 ) ) ;
#2231=VERTEX_POINT ( 'NONE', #10343 ) ;
#2234=CARTESIAN_POINT ( 'NONE',  ( 9.179055905797000037, -2.899999999999999911, 6.571291218949999902 ) ) ;
#2241=DIRECTION ( 'NONE',  ( 0.000000000000000000, 0.000000000000000000, -1.000000000000000000 ) ) ;
#2265=CARTESIAN_POINT ( 'NONE',  ( 7.642630378808000557, -9.064121401021999702, -5.575735562471000328 ) ) ;
#2267=CARTESIAN_POINT ( 'NONE',  ( 8.237893718522188991, -4.937145962667132792, 6.269524514844754037 ) ) ;
#2277=ORIENTED_EDGE ( 'NONE', *, *, #19880, .F. ) ;
#2283=CARTESIAN_POINT ( 'NONE',  ( 7.743183059623000020, -2.735207418315000361, 6.771977475428999860 ) ) ;
#2284=CARTESIAN_POINT ( 'NONE',  ( 8.470944094208999076, -5.100000000000000533, 6.571291218949999902 ) ) ;
#2289=LINE ( 'NONE', #29911, #35859 ) ;
#2294=EDGE_LOOP ( 'NONE', ( #17746, #39052 ) ) ;
#2295=CARTESIAN_POINT ( 'NONE',  ( 8.160745559622998968, -5.944572422272999646, 7.106845737860000511 ) ) ;
#2324=VERTEX_POINT ( 'NONE', #20838 ) ;
#2342=CARTESIAN_POINT ( 'NONE',  ( 10.02052890782000105, -2.899999999999999911, 6.152188490330000370 ) ) ;
#2346=ORIENTED_EDGE ( 'NONE', *, *, #26547, .T. ) ;
#2352=CARTESIAN_POINT ( 'NONE',  ( 10.98277446826000059, -2.518728855032000169, -8.314788219120000434 ) ) ;
#2355=EDGE_CURVE ( 'NONE', #20484, #34155, #69072, .T. ) ;
#2363=DIRECTION ( 'NONE',  ( -1.000000000000000000, 0.000000000000000000, 0.000000000000000000 ) ) ;
#2375=CARTESIAN_POINT ( 'NONE',  ( 8.335879440378999305, -4.310353212080000773, 9.459493062793997709 ) ) ;
#2388=CARTESIAN_POINT ( 'NONE',  ( 10.78089914631999946, -5.735295708369000600, 7.801561210335000496 ) ) ;
#2393=CARTESIAN_POINT ( 'NONE',  ( 7.911796541810308447, -2.452069608993371119, 8.293693421916961128 ) ) ;
#2394=CARTESIAN_POINT ( 'NONE',  ( 9.910792656537999790, -3.869344906782000049, 5.882544796414999944 ) ) ;
#2401=EDGE_CURVE ( 'NONE', #25841, #51664, #33749, .T. ) ;
#2403=ORIENTED_EDGE ( 'NONE', *, *, #65572, .T. ) ;
#2404=CARTESIAN_POINT ( 'NONE',  ( 9.751735624253999646, -3.361793157411000266, -5.915550373431999631 ) ) ;
#2407=CARTESIAN_POINT ( 'NONE',  ( 9.406851002546000373, -2.832432432432000269, -6.822293592207000934 ) ) ;
#2415=CARTESIAN_POINT ( 'NONE',  ( 9.240543146793999796, -4.158911960977000000, 5.873536005760000123 ) ) ;
#2420=CARTESIAN_POINT ( 'NONE',  ( 10.19122055961999962, -3.990707710465999813, -5.651373900265999950 ) ) ;
#2423=CARTESIAN_POINT ( 'NONE',  ( 7.474316494907240482, -3.999963201012326053, 8.979508826873761507 ) ) ;
#2435=AXIS2_PLACEMENT_3D ( 'NONE', #58659, #5519, #26859 ) ;
#2439=CARTESIAN_POINT ( 'NONE',  ( 5.500000000000000000, 0.000000000000000000, 0.000000000000000000 ) ) ;
#2459=CARTESIAN_POINT ( 'NONE',  ( 9.587879440377001572, -3.762710033898000184, 8.787827024292999667 ) ) ;
#2479=CARTESIAN_POINT ( 'NONE',  ( 7.800894438721999613, -3.218815632501999868, 6.398977300879999497 ) ) ;
#2483=CARTESIAN_POINT ( 'NONE',  ( 10.79325778752896525, -5.089851028638672226, 5.099140771708407627 ) ) ;
#2488=CARTESIAN_POINT ( 'NONE',  ( 10.87946694038000039, -2.817416132545000007, -6.828662897514999663 ) ) ;
#2489=EDGE_CURVE ( 'NONE', #62373, #67945, #62785, .T. ) ;
#2498=VERTEX_POINT ( 'NONE', #6564 ) ;
#2508=CARTESIAN_POINT ( 'NONE',  ( 10.09133114265999964, -2.216726401468000152, -8.007130485478999304 ) ) ;
#2515=FACE_OUTER_BOUND ( 'NONE', #56149, .T. ) ;
#2519=CARTESIAN_POINT ( 'NONE',  ( 10.98286725694000054, -3.998514182530999772, 9.091066422484001208 ) ) ;
#2520=VERTEX_POINT ( 'NONE', #59359 ) ;
#2529=CARTESIAN_POINT ( 'NONE',  ( 8.383148997457999130, -5.167567567567999731, 6.822293592207000934 ) ) ;
#2534=CARTESIAN_POINT ( 'NONE',  ( 9.881332132140999036, -4.333399685216000385, -9.088699530815999239 ) ) ;
#2541=CARTESIAN_POINT ( 'NONE',  ( 10.25832334068999963, -3.359820126011999974, 4.530776491823000462 ) ) ;
#2546=CARTESIAN_POINT ( 'NONE',  ( 11.11845396862999991, -5.767021056207999763, 7.178419201465000121 ) ) ;
#2562=CARTESIAN_POINT ( 'NONE',  ( 9.612156140204000110, -5.332339947063000629, -7.851654145788001138 ) ) ;
#2584=CARTESIAN_POINT ( 'NONE',  ( 10.91666666666863073, -5.385217356302812952, 7.523132604489776831 ) ) ;
#2586=CARTESIAN_POINT ( 'NONE',  ( 8.642077642326000841, -2.899999999999999911, 6.463854830420999953 ) ) ;
#2587=CARTESIAN_POINT ( 'NONE',  ( 5.600000001140999828, 0.000000000000000000, 0.000000000000000000 ) ) ;
#2589=ORIENTED_EDGE ( 'NONE', *, *, #20575, .F. ) ;
#2600=CARTESIAN_POINT ( 'NONE',  ( 9.407593387382531702, -2.496308800233906222, 8.374379778997440127 ) ) ;
#2606=CARTESIAN_POINT ( 'NONE',  ( 10.95262606961999907, -5.154900359228999918, -5.178689578204999755 ) ) ;
#2610=CARTESIAN_POINT ( 'NONE',  ( 9.629020610622001541, -5.794331084664000819, 7.414872097535999629 ) ) ;
#2613=EDGE_LOOP ( 'NONE', ( #63715, #59921, #49367 ) ) ;
#2623=CARTESIAN_POINT ( 'NONE',  ( 10.96256856629999987, -6.761408932091000246, 5.456131228213999762 ) ) ;
#2628=CARTESIAN_POINT ( 'NONE',  ( 10.89610713867999969, -2.705901429593000174, 4.900545273262999935 ) ) ;
#2636=CARTESIAN_POINT ( 'NONE',  ( 10.95375739185000086, -5.155102718910000270, 5.173734077849999835 ) ) ;
#2644=ORIENTED_EDGE ( 'NONE', *, *, #42100, .T. ) ;
#2647=CARTESIAN_POINT ( 'NONE',  ( 11.04968150330033438, -2.750318496699665438, -6.534572094925334085 ) ) ;
#2653=CARTESIAN_POINT ( 'NONE',  ( 8.574101921698924045, -3.981802517092035476, 5.760066862916072949 ) ) ;
#2662=CARTESIAN_POINT ( 'NONE',  ( 7.464688980125999684, -4.351670788182000038, 8.977200644264000218 ) ) ;
#2668=CARTESIAN_POINT ( 'NONE',  ( 11.09999999999999964, -5.299999999999999822, 6.469505845987999493 ) ) ;
#2671=CARTESIAN_POINT ( 'NONE',  ( 8.609967445932001695, -4.707159105298062585, 5.915074581558068978 ) ) ;
#2678=CARTESIAN_POINT ( 'NONE',  ( 9.817462135711998883, -5.100000000000000533, 6.571291218949999902 ) ) ;
#2680=CARTESIAN_POINT ( 'NONE',  ( 10.07314899745999881, -5.167567567567999731, -6.822293592207000934 ) ) ;
#2692=EDGE_CURVE ( 'NONE', #1683, #16661, #7828, .T. ) ;
#2696=ADVANCED_FACE ( 'NONE', ( #56190 ), #62753, .T. ) ;
#2698=CARTESIAN_POINT ( 'NONE',  ( 10.43283788151999936, -3.279327064383000145, -9.029275888523999427 ) ) ;
#2700=CARTESIAN_POINT ( 'NONE',  ( 9.061840010887420860, -4.635352338266921279, 8.712813424890676117 ) ) ;
#2704=CARTESIAN_POINT ( 'NONE',  ( 10.68797807636034847, -4.829546767829381970, -8.579382731881592505 ) ) ;
#2705=DIRECTION ( 'NONE',  ( -1.000000000000000000, 0.000000000000000000, 0.000000000000000000 ) ) ;
#2718=CARTESIAN_POINT ( 'NONE',  ( 7.373066940378000034, -3.394845988290999816, 9.388942682504000103 ) ) ;
#2722=ORIENTED_EDGE ( 'NONE', *, *, #61872, .T. ) ;
#2723=AXIS2_PLACEMENT_3D ( 'NONE', #2810, #24140, #45471 ) ;
#2732=CARTESIAN_POINT ( 'NONE',  ( 10.66951732929000052, -4.592671928130000580, 5.841406818427000047 ) ) ;
#2737=CARTESIAN_POINT ( 'NONE',  ( 7.967003474473192348, -2.304381480019767725, 7.113056951929115357 ) ) ;
#2738=CARTESIAN_POINT ( 'NONE',  ( 10.62197618263000010, -5.779779175739000685, 7.256573549370999743 ) ) ;
#2742=CARTESIAN_POINT ( 'NONE',  ( 10.34612086457000046, -4.749262201179999643, -4.718566242310000547 ) ) ;
#2759=ORIENTED_EDGE ( 'NONE', *, *, #62223, .F. ) ;
#2760=CARTESIAN_POINT ( 'NONE',  ( 8.534480646793999981, -3.011617647609999615, 8.801438026873999121 ) ) ;
#2761=CARTESIAN_POINT ( 'NONE',  ( 7.474999999999999645, -5.349999999999999645, 7.500000000000000000 ) ) ;
#2766=CARTESIAN_POINT ( 'NONE',  ( 10.69829435321000055, -2.534030585780999711, -6.667788699001999220 ) ) ;
#2780=AXIS2_PLACEMENT_3D ( 'NONE', #15144, #3275, #8180 ) ;
#2782=DIRECTION ( 'NONE',  ( 1.000000000000000000, 0.000000000000000000, 0.000000000000000000 ) ) ;
#2785=ORIENTED_EDGE ( 'NONE', *, *, #25253, .T. ) ;
#2801=CARTESIAN_POINT ( 'NONE',  ( 7.443293146792999693, -4.698358408974000255, 8.789434435623999065 ) ) ;
#2802=PLANE ( 'NONE',  #40727 ) ;
#2810=CARTESIAN_POINT ( 'NONE',  ( 7.000000000000000000, 0.000000000000000000, 0.000000000000000000 ) ) ;
#2814=CARTESIAN_POINT ( 'NONE',  ( 7.822379440378000481, -4.636725880537000855, 9.378965771357000492 ) ) ;
#2818=CARTESIAN_POINT ( 'NONE',  ( 7.449893704810870432, -2.260907433923616150, 7.482160321753426935 ) ) ;
#2822=DIRECTION ( 'NONE',  ( 0.8660254038003750710, -1.114487574551968024E-07, -0.4999999999723849786 ) ) ;
#2823=CARTESIAN_POINT ( 'NONE',  ( 11.08613868670750335, -2.236165381191161039, -7.580675004253683902 ) ) ;
#2830=CARTESIAN_POINT ( 'NONE',  ( 10.38725444037999956, -2.888666857901000196, -6.716331201355000502 ) ) ;
#2833=EDGE_CURVE ( 'NONE', #17467, #8257, #41138, .T. ) ;
#2839=CARTESIAN_POINT ( 'NONE',  ( 10.31746213571000048, -5.100000000000000533, 6.571291218949999902 ) ) ;
#2848=CARTESIAN_POINT ( 'NONE',  ( 10.76010362286999822, -4.535387425205000156, 6.001717576299999024 ) ) ;
#2854=VERTEX_POINT ( 'NONE', #18794 ) ;
#2855=EDGE_CURVE ( 'NONE', #16623, #2498, #14513, .T. ) ;
#2861=CARTESIAN_POINT ( 'NONE',  ( 10.53733998880999856, -2.992814141720000265, 8.731692578598000409 ) ) ;
#2867=B_SPLINE_CURVE_WITH_KNOTS ( 'NONE', 3,
 ( #254, #27516, #31732, #58987, #63532, #53052, #16327, #11088 ),
 .UNSPECIFIED., .F., .F.,
 ( 4, 1, 1, 1, 1, 4 ),
 ( 0.2125974459517032678, 0.3245965717578418452, 0.5241428039294082630, 0.7236890361001979688, 0.9232352682709885627, 1.000000000000000000 ),
 .UNSPECIFIED. ) ;
#2868=CARTESIAN_POINT ( 'NONE',  ( 10.52052890781999928, -2.899999999999999911, 6.152188490330000370 ) ) ;
#2872=B_SPLINE_CURVE_WITH_KNOTS ( 'NONE', 3,
 ( #23840, #13365, #37335, #48172, #25211 ),
 .UNSPECIFIED., .F., .F.,
 ( 4, 1, 4 ),
 ( 0.000000000000000000, 0.3670466485305822757, 1.000000000000000000 ),
 .UNSPECIFIED. ) ;
#2880=CARTESIAN_POINT ( 'NONE',  ( 9.086718600414000591, -4.531444417037000072, -6.133284059228000018 ) ) ;
#2890=CARTESIAN_POINT ( 'NONE',  ( 10.80815535238000002, -2.937528991339000140, 8.948455587554001056 ) ) ;
#2900=CARTESIAN_POINT ( 'NONE',  ( 10.96459579918999871, -2.848437942114999899, 5.071485159340999971 ) ) ;
#2904=CARTESIAN_POINT ( 'NONE',  ( 9.883915020958999875, -5.811247906278000031, -7.978055797018001272 ) ) ;
#2916=ORIENTED_EDGE ( 'NONE', *, *, #57098, .T. ) ;
#2927=CARTESIAN_POINT ( 'NONE',  ( 11.07928131834999874, -7.977359646417001571, 6.935621157201000031 ) ) ;
#2941=CARTESIAN_POINT ( 'NONE',  ( 5.500000000000000000, 0.000000000000000000, 0.000000000000000000 ) ) ;
#2942=CARTESIAN_POINT ( 'NONE',  ( 9.382165295667087790, -2.854056800879049671, 8.808963309177558543 ) ) ;
#2946=CARTESIAN_POINT ( 'NONE',  ( 9.947724669985010593, -5.285954009497336514, 7.027653896126389022 ) ) ;
#2950=CARTESIAN_POINT ( 'NONE',  ( 10.62197618263000010, -5.779779175739000685, 7.256573549370999743 ) ) ;
#2953=CARTESIAN_POINT ( 'NONE',  ( 7.100000000000000533, 0.000000000000000000, 0.000000000000000000 ) ) ;
#2955=ORIENTED_EDGE ( 'NONE', *, *, #65162, .F. ) ;
#2966=CARTESIAN_POINT ( 'NONE',  ( 11.07074860546000039, -5.433615603927000492, 5.078288009826000149 ) ) ;
#2971=CARTESIAN_POINT ( 'NONE',  ( 10.73883163666999963, -2.873420258502000113, -5.007713218437999991 ) ) ;
#2975=ORIENTED_EDGE ( 'NONE', *, *, #16779, .T. ) ;
#2976=CARTESIAN_POINT ( 'NONE',  ( 10.95899882946999959, -5.155721817611999214, 5.124270346052999692 ) ) ;
#2977=LINE ( 'NONE', #7889, #44094 ) ;
#2979=CARTESIAN_POINT ( 'NONE',  ( 7.750036073563001615, -5.085252754069001568, 6.546627699621002883 ) ) ;
#2999=CARTESIAN_POINT ( 'NONE',  ( 9.611390067472999732, -3.334847606888000193, 5.869121315726000709 ) ) ;
#3002=CARTESIAN_POINT ( 'NONE',  ( 8.534480646793999981, -3.011617647609999615, 8.801438026873999121 ) ) ;
#3006=CARTESIAN_POINT ( 'NONE',  ( 6.831155956914999550, -9.270367636368000319, 5.219306890235999141 ) ) ;
#3013=CARTESIAN_POINT ( 'NONE',  ( 8.721802827889566956, -2.874603711571219744, 6.749639981086952290 ) ) ;
#3015=CARTESIAN_POINT ( 'NONE',  ( 11.09999999999999964, -6.075667615221999718, -5.238593909383999048 ) ) ;
#3026=CARTESIAN_POINT ( 'NONE',  ( 11.09999999999999964, -1.300000000000000044, -9.662944685757000940 ) ) ;
#3036=CARTESIAN_POINT ( 'NONE',  ( 9.922182479546000522, -3.489927462211000364, -9.111803974470001677 ) ) ;
#3047=CIRCLE ( 'NONE', #46627, 0.5000000000000004441 ) ;
#3056=CARTESIAN_POINT ( 'NONE',  ( 7.550620559621999739, -4.468370631666999770, 8.882152684713000568 ) ) ;
#3070=CARTESIAN_POINT ( 'NONE',  ( 9.743567407955000093, -5.287392049455999832, 8.939957179821000466 ) ) ;
#3075=ADVANCED_FACE ( 'NONE', ( #34106 ), #50517, .T. ) ;
#3076=CARTESIAN_POINT ( 'NONE',  ( 11.10664194037999941, -5.324199331986000594, -7.809344861333999965 ) ) ;
#3077=CARTESIAN_POINT ( 'NONE',  ( 7.966914046381088355, -2.303960697091592014, 7.114913321231458809 ) ) ;
#3078=CARTESIAN_POINT ( 'NONE',  ( 9.848732933287999813, -2.769734897491000325, 6.441850735262000249 ) ) ;
#3082=CARTESIAN_POINT ( 'NONE',  ( 10.35353477906000030, -4.571505382416000351, -4.862086577461999681 ) ) ;
#3084=EDGE_LOOP ( 'NONE', ( #18436, #5800, #47000, #44840, #64223 ) ) ;
#3087=CARTESIAN_POINT ( 'NONE',  ( 9.397139116365000433, -4.993413662858000812, -9.088148847710000311 ) ) ;
#3099=CARTESIAN_POINT ( 'NONE',  ( 9.176355646795000709, -2.935738482289000029, 6.259841087764999479 ) ) ;
#3106=CARTESIAN_POINT ( 'NONE',  ( 11.09178064679000109, -4.578543110806999827, -8.908602356389000221 ) ) ;
#3115=CARTESIAN_POINT ( 'NONE',  ( 8.560832189570803052, -5.056892070296432173, 6.275968648838331276 ) ) ;
#3118=VECTOR ( 'NONE', #55368, 1000.000000000000227 ) ;
#3131=B_SPLINE_CURVE_WITH_KNOTS ( 'NONE', 3,
 ( #49086, #43849, #1198, #27080 ),
 .UNSPECIFIED., .F., .F.,
 ( 4, 4 ),
 ( 0.000000000000000000, 0.1255288163819863745 ),
 .UNSPECIFIED. ) ;
#3146=CARTESIAN_POINT ( 'NONE',  ( 7.764230646791999924, -4.628942671846000501, 5.991663889842000046 ) ) ;
#3147=DIRECTION ( 'NONE',  ( 0.000000000000000000, -0.7071067811865475727, -0.7071067811865475727 ) ) ;
#3153=CARTESIAN_POINT ( 'NONE',  ( 11.07213888212999997, -2.731532893235999904, -5.080375744811999716 ) ) ;
#3155=PLANE ( 'NONE',  #42507 ) ;
#3157=B_SPLINE_CURVE_WITH_KNOTS ( 'NONE', 3,
 ( #38807, #33913, #39846, #50334 ),
 .UNSPECIFIED., .F., .F.,
 ( 4, 4 ),
 ( 0.8719585443747394082, 1.000000000000000000 ),
 .UNSPECIFIED. ) ;
#3158=CARTESIAN_POINT ( 'NONE',  ( 5.699999999554000496, -0.3000000004460000036, 9.662944681662999358 ) ) ;
#3162=CARTESIAN_POINT ( 'NONE',  ( 9.298691940377999288, -5.159251056493999954, 9.109488373271000583 ) ) ;
#3165=EDGE_CURVE ( 'NONE', #21223, #852, #54504, .T. ) ;
#3167=CARTESIAN_POINT ( 'NONE',  ( 7.446475209053147637, -2.261386354369964824, 7.556112484256551909 ) ) ;
#3171=VERTEX_POINT ( 'NONE', #23950 ) ;
#3175=CYLINDRICAL_SURFACE ( 'NONE', #64330, 0.5000000000000000000 ) ;
#3179=CARTESIAN_POINT ( 'NONE',  ( 9.612308556531111492, -3.034755127823582921, 8.468084591988906951 ) ) ;
#3180=DIRECTION ( 'NONE',  ( 0.000000000000000000, -0.2461538461537955691, -0.9692307692307821076 ) ) ;
#3181=CARTESIAN_POINT ( 'NONE',  ( 7.816481737960005560, -3.426408505174418195, 6.252170097456407838 ) ) ;
#3197=CARTESIAN_POINT ( 'NONE',  ( 9.479212726990999371, -4.071727350623000063, 9.089303488377000306 ) ) ;
#3199=CARTESIAN_POINT ( 'NONE',  ( 10.68054891417000007, -2.768175152062000155, -6.114413274984999980 ) ) ;
#3203=CARTESIAN_POINT ( 'NONE',  ( 11.12486991174999851, -5.426792458777999428, -5.164830891052999640 ) ) ;
#3210=CARTESIAN_POINT ( 'NONE',  ( 9.687876499438001332, -5.912252057206999645, 7.772299417761000306 ) ) ;
#3216=ORIENTED_EDGE ( 'NONE', *, *, #19477, .F. ) ;
#3227=CARTESIAN_POINT ( 'NONE',  ( 9.174722005181999762, -5.536248950452999473, -7.355084988757000453 ) ) ;
#3235=DIRECTION ( 'NONE',  ( 0.000000000000000000, -1.000000000000000000, 0.000000000000000000 ) ) ;
#3239=CARTESIAN_POINT ( 'NONE',  ( 9.166075977534999808, -4.023333687735000552, 9.122281080215000060 ) ) ;
#3242=CARTESIAN_POINT ( 'NONE',  ( 9.615066448851507630, -5.349942704376990044, -7.499996115248991124 ) ) ;
#3247=CARTESIAN_POINT ( 'NONE',  ( 10.68287132187968602, -5.051222535738905783, -5.058047779293387336 ) ) ;
#3253=CARTESIAN_POINT ( 'NONE',  ( 8.996132306828998892, -4.474581801608000120, -6.279517683005999551 ) ) ;
#3259=CARTESIAN_POINT ( 'NONE',  ( 10.03695705046682818, -5.286467410629250629, -7.027033154920563796 ) ) ;
#3274=EDGE_CURVE ( 'NONE', #12955, #37266, #55075, .T. ) ;
#3275=DIRECTION ( 'NONE',  ( 1.000000000000000000, 0.000000000000000000, 0.000000000000000000 ) ) ;
#3276=ORIENTED_EDGE ( 'NONE', *, *, #54353, .F. ) ;
#3299=ORIENTED_EDGE ( 'NONE', *, *, #45108, .T. ) ;
#3304=CARTESIAN_POINT ( 'NONE',  ( 7.465326089856205272, -5.349750919053078313, 7.322903698185732502 ) ) ;
#3314=CARTESIAN_POINT ( 'NONE',  ( 9.888906509039999904, -2.890602650755999647, -6.682694598879999504 ) ) ;
#3333=ORIENTED_EDGE ( 'NONE', *, *, #20575, .T. ) ;
#3340=ORIENTED_EDGE ( 'NONE', *, *, #61926, .T. ) ;
#3341=CARTESIAN_POINT ( 'NONE',  ( 9.534903635507999908, -3.030945724184999968, 8.761987396837000119 ) ) ;
#3344=CARTESIAN_POINT ( 'NONE',  ( 8.304129440378000382, -3.650411072918999800, 6.083135626079000602 ) ) ;
#3347=ORIENTED_EDGE ( 'NONE', *, *, #56436, .F. ) ;
#3350=CARTESIAN_POINT ( 'NONE',  ( 11.09999422944000003, -1.406550927767000081, 10.45582307705999980 ) ) ;
#3351=EDGE_CURVE ( 'NONE', #51171, #61050, #53944, .T. ) ;
#3355=CARTESIAN_POINT ( 'NONE',  ( 10.89874164595999950, -2.834836218627000193, 9.088455567997000273 ) ) ;
#3357=CARTESIAN_POINT ( 'NONE',  ( 11.09999999999999964, -5.556657014908000569, -5.124965748850000224 ) ) ;
#3362=CARTESIAN_POINT ( 'NONE',  ( 11.02452225494999993, -2.775477745048999800, -6.571291218949999902 ) ) ;
#3369=EDGE_LOOP ( 'NONE', ( #61943, #44800, #6576, #9043 ) ) ;
#3375=CARTESIAN_POINT ( 'NONE',  ( 9.973487588364999823, -4.344961837988999598, -9.321582626371998970 ) ) ;
#3378=ORIENTED_EDGE ( 'NONE', *, *, #63757, .T. ) ;
#3395=CARTESIAN_POINT ( 'NONE',  ( 7.897956853208000005, -3.608524635952000459, 5.913372239166000632 ) ) ;
#3399=DIRECTION ( 'NONE',  ( -1.000000000000000000, 0.000000000000000000, 0.000000000000000000 ) ) ;
#3407=ORIENTED_EDGE ( 'NONE', *, *, #61529, .T. ) ;
#3417=CARTESIAN_POINT ( 'NONE',  ( 8.227919288421315258, -5.628404604175369030, 8.112053306693633559 ) ) ;
#3421=CARTESIAN_POINT ( 'NONE',  ( 10.38053123589000037, -4.707947451838999875, -5.013008711266000006 ) ) ;
#3426=FACE_OUTER_BOUND ( 'NONE', #12221, .T. ) ;
#3435=CARTESIAN_POINT ( 'NONE',  ( 8.855418146794999501, -5.633481712366999794, 7.451234046297000368 ) ) ;
#3440=CARTESIAN_POINT ( 'NONE',  ( 10.56170564679000101, -5.057490041178001050, -8.595713413570999606 ) ) ;
#3441=CARTESIAN_POINT ( 'NONE',  ( 8.475341021510246264, -5.350570349241358770, 7.499981640446112152 ) ) ;
#3448=CARTESIAN_POINT ( 'NONE',  ( 8.614144221484336228, -4.937690759611556679, 6.045737820659460304 ) ) ;
#3450=ORIENTED_EDGE ( 'NONE', *, *, #39707, .T. ) ;
#3451=CARTESIAN_POINT ( 'NONE',  ( 10.27669459503999860, -4.581840238100999940, 5.003918118598999598 ) ) ;
#3456=AXIS2_PLACEMENT_3D ( 'NONE', #4224, #16435, #15067 ) ;
#3474=CLOSED_SHELL ( 'NONE', ( #28195, #17438, #68773, #19112, #26004, #23320, #22416, #45394, #47214, #46509, #33819, #65301, #62948, #8663, #61282, #19216, #21792, #7686, #34104, #11873, #31846, #60807, #30869, #19196, #40315, #7528, #66177, #45704, #37950, #7274, #37336, #51691, #68046, #42924, #46259, #37998, #4392, #62477, #41735, #1286, #10192, #3075, #8153, #26939, #60158, #32528, #16986, #51991, #5002, #31962, #62475, #32851, #4389, #705, #29629, #2696, #5033, #19055, #47007, #9517, #44482, #37639, #5438, #49841, #34185, #14878, #37872, #1964, #42276, #4958, #41741, #6971, #47662, #1449, #56238, #64684, #68248, #25729, #39874, #20513, #22999, #66381, #12726, #35288, #36862, #48965, #22577, #67823, #61981, #58308, #36891, #10721, #13970, #32198, #22521, #56187, #66404, #61200, #56518, #61839, #16108, #13933, #66134, #48631, #30784, #1567, #17259, #48352, #302, #31888, #8607, #62503, #56292, #61239, #20149, #51905, #50451, #14528, #51147, #43049, #15659, #31407, #32284, #18974, #65905, #19736, #16479, #44457, #29627, #48218, #29286, #46735, #62228, #32526, #12533, #50756, #1570, #60692, #38053, #1336, #35669, #13339, #11957, #39272, #30332, #59835, #4556, #35587, #17858, #34417, #33337, #46180, #16356, #51270, #61749, #58614, #10519, #7575, #22722, #21936, #10866, #296, #28976, #38746, #69003, #67771, #18932, #16390, #62369, #65956, #6713, #50272, #19277, #66566, #12394, #61108, #16525, #50130, #52221, #55966 ) ) ;
#3478=VERTEX_POINT ( 'NONE', #58504 ) ;
#3481=CARTESIAN_POINT ( 'NONE',  ( 10.64079374716282800, -5.301110017552429277, 6.316741276523229587 ) ) ;
#3482=CARTESIAN_POINT ( 'NONE',  ( 7.464688980125999684, -4.351670788182000038, 8.977200644264000218 ) ) ;
#3486=ORIENTED_EDGE ( 'NONE', *, *, #16665, .T. ) ;
#3488=EDGE_CURVE ( 'NONE', #23313, #22584, #53266, .T. ) ;
#3497=CARTESIAN_POINT ( 'NONE',  ( 8.592629440379999650, -3.856773448568000084, 5.521258396339000285 ) ) ;
#3498=EDGE_LOOP ( 'NONE', ( #1257, #5484, #49726, #46063, #29954 ) ) ;
#3501=CARTESIAN_POINT ( 'NONE',  ( 7.441574459899483962, -2.267067028809165219, 7.663462709907783221 ) ) ;
#3513=CARTESIAN_POINT ( 'NONE',  ( 8.576923877145999242, -3.399999999999999911, 5.924121105096999962 ) ) ;
#3530=CARTESIAN_POINT ( 'NONE',  ( 10.12670810574000058, -3.117521507207000386, 8.613544937223998943 ) ) ;
#3535=ORIENTED_EDGE ( 'NONE', *, *, #485, .F. ) ;
#3536=CARTESIAN_POINT ( 'NONE',  ( 10.96504121510999852, -6.670435863508999752, -5.365570440722000178 ) ) ;
#3542=CARTESIAN_POINT ( 'NONE',  ( 11.09999999999999964, -4.000000000000000000, 7.500000000000000000 ) ) ;
#3551=CARTESIAN_POINT ( 'NONE',  ( 10.98768472625999948, -5.449702614167000192, -4.945212061590999575 ) ) ;
#3566=CARTESIAN_POINT ( 'NONE',  ( 10.97807333593999957, -5.235090452703000885, -6.783100406990000053 ) ) ;
#3582=CARTESIAN_POINT ( 'NONE',  ( 8.887782330080007398, -3.105205165878999196, -6.157731156825001051 ) ) ;
#3585=CARTESIAN_POINT ( 'NONE',  ( 9.353311703536000721, -4.905858243509999106, -8.948175900338000588 ) ) ;
#3587=DIRECTION ( 'NONE',  ( 1.000000000000000000, 0.000000000000000000, 0.000000000000000000 ) ) ;
#3589=CARTESIAN_POINT ( 'NONE',  ( 10.26195629121000152, -4.600000265269999389, 4.591198190832999515 ) ) ;
#3597=CARTESIAN_POINT ( 'NONE',  ( 9.156713723001384864, -5.179807657556271927, -8.179981299039964071 ) ) ;
#3601=FACE_OUTER_BOUND ( 'NONE', #56676, .T. ) ;
#3602=DIRECTION ( 'NONE',  ( 0.000000000000000000, 1.000000000000000000, 0.000000000000000000 ) ) ;
#3608=EDGE_CURVE ( 'NONE', #46752, #65197, #2205, .T. ) ;
#3622=DIRECTION ( 'NONE',  ( 0.000000000000000000, 0.8648648648648720183, 0.5020047465136825426 ) ) ;
#3631=DIRECTION ( 'NONE',  ( 1.000000000000000000, -2.025400574418000070E-14, -2.893429392025000534E-14 ) ) ;
#3632=CARTESIAN_POINT ( 'NONE',  ( 10.64447714202000128, -5.073836261934999925, -8.340686666652999293 ) ) ;
#3637=CARTESIAN_POINT ( 'NONE',  ( 7.434063311431996723, -5.180700782550064609, 6.820069141833377202 ) ) ;
#3643=CARTESIAN_POINT ( 'NONE',  ( 8.344928245395999866, -4.790498497136999489, -6.523246444533000954 ) ) ;
#3648=CARTESIAN_POINT ( 'NONE',  ( 10.61390167354000091, -2.793204138329999697, -4.716480657362000173 ) ) ;
#3649=CARTESIAN_POINT ( 'NONE',  ( 10.01832872737000102, -5.491975933468000726, -7.893788029530999673 ) ) ;
#3651=CARTESIAN_POINT ( 'NONE',  ( 9.884778143176074394, -2.675332436538061742, -7.165830604257146241 ) ) ;
#3655=AXIS2_PLACEMENT_3D ( 'NONE', #56151, #12128, #54772 ) ;
#3665=ORIENTED_EDGE ( 'NONE', *, *, #53282, .T. ) ;
#3672=EDGE_LOOP ( 'NONE', ( #15756, #21183, #46185, #55962 ) ) ;
#3673=CARTESIAN_POINT ( 'NONE',  ( 10.64872180584000105, -2.614778238704999591, 6.717279975758000177 ) ) ;
#3675=CARTESIAN_POINT ( 'NONE',  ( -15.86200481174999943, -2.399999999999999911, 6.571291218949999902 ) ) ;
#3688=CARTESIAN_POINT ( 'NONE',  ( 11.20904026220999938, -5.937811873294999820, 7.147336919140999001 ) ) ;
#3692=CARTESIAN_POINT ( 'NONE',  ( 10.17310292480999934, -4.709171320598000143, -8.664883863910000983 ) ) ;
#3699=CARTESIAN_POINT ( 'NONE',  ( 10.46166951222632591, -5.351570712698000776, 7.263306442112493322 ) ) ;
#3700=DIRECTION ( 'NONE',  ( 0.000000000000000000, 1.000000000000000000, 0.000000000000000000 ) ) ;
#3704=CARTESIAN_POINT ( 'NONE',  ( 8.185765847591000011, -4.942196905450001232, 6.196983455206997782 ) ) ;
#3712=CARTESIAN_POINT ( 'NONE',  ( 10.51140025105000042, -2.326718149302000160, -7.741209600718000239 ) ) ;
#3715=CARTESIAN_POINT ( 'NONE',  ( 9.001479836347179742, -5.278236052291213731, 7.933966972496419245 ) ) ;
#3721=CARTESIAN_POINT ( 'NONE',  ( 7.565629440376999248, -3.206365290996999740, 5.681739161071000410 ) ) ;
#3735=CARTESIAN_POINT ( 'NONE',  ( 7.320269353207000229, -2.466384407480000096, 6.935560677555000275 ) ) ;
#3740=CIRCLE ( 'NONE', #62925, 10.75000000000000533 ) ;
#3753=CARTESIAN_POINT ( 'NONE',  ( 8.119297623376104056, -4.926355840723960711, 6.024311677146462429 ) ) ;
#3757=CARTESIAN_POINT ( 'NONE',  ( 10.42469759965999998, -4.813117804065999650, -5.025876989183999832 ) ) ;
#3774=B_SPLINE_CURVE_WITH_KNOTS ( 'NONE', 3,
 ( #41596, #67463, #15373, #30766 ),
 .UNSPECIFIED., .F., .F.,
 ( 4, 4 ),
 ( 0.000000000000000000, 1.000000000000000000 ),
 .UNSPECIFIED. ) ;
#3775=CARTESIAN_POINT ( 'NONE',  ( 7.968183059622999664, -2.280579276705999803, 6.510290672242000198 ) ) ;
#3780=CARTESIAN_POINT ( 'NONE',  ( 10.33453064679000200, -3.295701412239999684, -6.149875347297999895 ) ) ;
#3789=EDGE_LOOP ( 'NONE', ( #67150, #61530, #29888, #3276 ) ) ;
#3800=CARTESIAN_POINT ( 'NONE',  ( 10.13586576648898330, -5.314625264832349316, -7.853278872971151792 ) ) ;
#3833=CARTESIAN_POINT ( 'NONE',  ( 7.694004440376999376, -5.850279024084999335, 6.784181137144999596 ) ) ;
#3837=CARTESIAN_POINT ( 'NONE',  ( 10.45625805961999966, -3.661873208228000109, -9.317463915629002003 ) ) ;
#3838=CARTESIAN_POINT ( 'NONE',  ( 7.458084730951140884, -2.267780973363890062, 7.308742852188579775 ) ) ;
#3839=AXIS2_PLACEMENT_3D ( 'NONE', #61094, #50949, #67017 ) ;
#3845=CARTESIAN_POINT ( 'NONE',  ( 11.07236672166249924, -2.278048615010975553, -7.888876361990175390 ) ) ;
#3860=CARTESIAN_POINT ( 'NONE',  ( 8.941938785621264429, -5.237454815711724443, 6.943328879398332099 ) ) ;
#3863=ORIENTED_EDGE ( 'NONE', *, *, #13383, .F. ) ;
#3864=CARTESIAN_POINT ( 'NONE',  ( 10.56690934386000080, -5.170965040585000061, 4.739956486541999858 ) ) ;
#3870=CARTESIAN_POINT ( 'NONE',  ( 10.73930809942999964, -2.762991917822000154, 6.801028165221000066 ) ) ;
#3878=CYLINDRICAL_SURFACE ( 'NONE', #2435, 1.000000000000000000 ) ;
#3884=CARTESIAN_POINT ( 'NONE',  ( 10.52324012719000024, -3.325647021086999722, 5.689999163383999026 ) ) ;
#3894=CARTESIAN_POINT ( 'NONE',  ( 27.64127793187000037, -2.399999999999999911, -6.571291218949999902 ) ) ;
#3899=CARTESIAN_POINT ( 'NONE',  ( 9.957251191599000961, -4.686746084135999801, -9.174865097765998456 ) ) ;
#3910=DIRECTION ( 'NONE',  ( 1.000000000000000000, 0.000000000000000000, 0.000000000000000000 ) ) ;
#3923=CARTESIAN_POINT ( 'NONE',  ( 10.86169145887000020, -2.934707142245000178, 5.180212859994000496 ) ) ;
#3926=CARTESIAN_POINT ( 'NONE',  ( 10.96990540416000037, -2.852123108999999879, -5.029685703292000376 ) ) ;
#3927=CARTESIAN_POINT ( 'NONE',  ( 10.64557055961999943, -2.988935764546999607, -5.952339209104000162 ) ) ;
#3940=CARTESIAN_POINT ( 'NONE',  ( 9.135881449927612863, -5.314639390875580460, -7.853423517146890909 ) ) ;
#3949=CARTESIAN_POINT ( 'NONE',  ( 9.716851002543000604, -2.832432432432000269, 6.822293592207000934 ) ) ;
#3950=EDGE_LOOP ( 'NONE', ( #15795, #10678, #37059, #68015, #13253, #23913, #23584, #30978, #63029, #47219, #26395, #50303, #62739, #26387, #67509 ) ) ;
#3956=ORIENTED_EDGE ( 'NONE', *, *, #56717, .F. ) ;
#3962=FACE_OUTER_BOUND ( 'NONE', #7902, .T. ) ;
#3964=VERTEX_POINT ( 'NONE', #38127 ) ;
#3967=CARTESIAN_POINT ( 'NONE',  ( 8.433148997460000018, -5.167567567567999731, 6.822293592207000934 ) ) ;
#3971=CARTESIAN_POINT ( 'NONE',  ( 9.831596185961002377, -3.539228349258999984, -8.956015611440999891 ) ) ;
#3986=AXIS2_PLACEMENT_3D ( 'NONE', #21445, #47689, #31268 ) ;
#3987=CARTESIAN_POINT ( 'NONE',  ( 7.722414202460995192, -2.834216095980001349, 6.826613447391997269 ) ) ;
#3989=EDGE_CURVE ( 'NONE', #42529, #68830, #33579, .T. ) ;
#3990=CARTESIAN_POINT ( 'NONE',  ( 9.756901401888999459, -3.283392111224999965, -8.676955243274001361 ) ) ;
#3992=CARTESIAN_POINT ( 'NONE',  ( 9.906851002540999929, -2.832432432432000269, -6.822293592207000934 ) ) ;
#3993=CARTESIAN_POINT ( 'NONE',  ( 11.04626556088000022, -5.245434002695000153, 5.120146859325999777 ) ) ;
#4012=CARTESIAN_POINT ( 'NONE',  ( 9.610944094206999466, -5.100000000000000533, -6.571291218949999902 ) ) ;
#4017=CARTESIAN_POINT ( 'NONE',  ( 10.70441271436000008, -3.444516450945999786, 6.009051312948000323 ) ) ;
#4018=ORIENTED_EDGE ( 'NONE', *, *, #20354, .T. ) ;
#4019=CARTESIAN_POINT ( 'NONE',  ( 9.432978986056474113, -5.350301812018463110, 7.637514618902952357 ) ) ;
#4020=CARTESIAN_POINT ( 'NONE',  ( 8.085168146793000332, -2.431397064767999439, 7.958394431095000776 ) ) ;
#4032=ORIENTED_EDGE ( 'NONE', *, *, #5456, .T. ) ;
#4033=CARTESIAN_POINT ( 'NONE',  ( 10.21238410957999854, -4.072568653311000375, -8.861841462475000597 ) ) ;
#4055=CARTESIAN_POINT ( 'NONE',  ( 10.19715077290999972, -4.982624057277000418, -6.124316828241999744 ) ) ;
#4057=CARTESIAN_POINT ( 'NONE',  ( 9.039803704978325527, -4.929474118734117560, 8.478877421443728579 ) ) ;
#4058=ORIENTED_EDGE ( 'NONE', *, *, #39003, .T. ) ;
#4061=B_SPLINE_CURVE_WITH_KNOTS ( 'NONE', 3,
 ( #22470, #49388, #49741, #1158, #17234 ),
 .UNSPECIFIED., .F., .F.,
 ( 4, 1, 4 ),
 ( 0.000000000000000000, 0.5000000000000000000, 1.000000000000000000 ),
 .UNSPECIFIED. ) ;
#4068=CARTESIAN_POINT ( 'NONE',  ( 10.76947109217999810, -5.100000000000000533, -6.152188490330000370 ) ) ;
#4070=EDGE_CURVE ( 'NONE', #44229, #51258, #40720, .T. ) ;
#4077=CARTESIAN_POINT ( 'NONE',  ( 7.871558059623000148, -4.780993534312999671, 6.267212032957000467 ) ) ;
#4090=CARTESIAN_POINT ( 'NONE',  ( 9.210982939512550871, -5.015527360726283135, -6.211259001266990154 ) ) ;
#4092=CARTESIAN_POINT ( 'NONE',  ( 7.954503319898948988, -5.004866943022359571, 6.489198313767416515 ) ) ;
#4094=CARTESIAN_POINT ( 'NONE',  ( 10.90000000042000039, -0.3000000004212000082, -9.662944680462999258 ) ) ;
#4095=ORIENTED_EDGE ( 'NONE', *, *, #40021, .T. ) ;
#4098=CARTESIAN_POINT ( 'NONE',  ( 8.218406721992218777, -5.687944966856361972, 7.919044992995649679 ) ) ;
#4102=CARTESIAN_POINT ( 'NONE',  ( 9.225602416349406809, -4.497379437544680947, 9.030677449726647765 ) ) ;
#4114=ORIENTED_EDGE ( 'NONE', *, *, #706, .T. ) ;
#4117=DIRECTION ( 'NONE',  ( 0.000000000000000000, 1.000000000000000000, 1.181194577550999990E-14 ) ) ;
#4122=CARTESIAN_POINT ( 'NONE',  ( 10.82674314678999927, -3.167157901876000103, -6.225148200207000215 ) ) ;
#4123=CARTESIAN_POINT ( 'NONE',  ( 9.365000000002998704, -2.649999999999999911, -7.500000000000000000 ) ) ;
#4129=CARTESIAN_POINT ( 'NONE',  ( 11.09999999999999964, -0.5000000000000000000, -5.124965750789000296 ) ) ;
#4130=CARTESIAN_POINT ( 'NONE',  ( 8.542969685731069518, -5.075224516770981076, 6.339907061512210618 ) ) ;
#4143=ORIENTED_EDGE ( 'NONE', *, *, #11505, .T. ) ;
#4159=CARTESIAN_POINT ( 'NONE',  ( 9.225036374688860619, -2.649952446100997339, 7.500002253091946791 ) ) ;
#4162=CARTESIAN_POINT ( 'NONE',  ( 10.98768491210000064, -8.067891622241001315, 6.818837029638999958 ) ) ;
#4169=ORIENTED_EDGE ( 'NONE', *, *, #52791, .F. ) ;
#4181=CARTESIAN_POINT ( 'NONE',  ( 7.565629440376999248, -3.206365290996999740, 5.681739161071000410 ) ) ;
#4188=CARTESIAN_POINT ( 'NONE',  ( 7.526976851188666551, -3.029433660751889690, 6.048151158366446900 ) ) ;
#4199=AXIS2_PLACEMENT_3D ( 'NONE', #14506, #41415, #14844 ) ;
#4206=ORIENTED_EDGE ( 'NONE', *, *, #24704, .T. ) ;
#4209=EDGE_LOOP ( 'NONE', ( #39408, #68302, #28412, #30210 ) ) ;
#4215=CARTESIAN_POINT ( 'NONE',  ( 9.532671748231999587, -4.663050389319001177, 8.669823109968998409 ) ) ;
#4224=CARTESIAN_POINT ( 'NONE',  ( 11.09999999999999964, -4.000000000000000000, -7.500000000000000000 ) ) ;
#4229=CARTESIAN_POINT ( 'NONE',  ( 11.00366278039000001, -2.264082614160999984, 7.798350693290999835 ) ) ;
#4231=CARTESIAN_POINT ( 'NONE',  ( 9.266851002542999538, -2.832432432432000269, 6.822293592207000934 ) ) ;
#4236=CARTESIAN_POINT ( 'NONE',  ( 9.910792656537999790, -3.869344906782000049, 5.882544796414999944 ) ) ;
#4255=AXIS2_PLACEMENT_3D ( 'NONE', #46942, #3587, #4279 ) ;
#4270=CARTESIAN_POINT ( 'NONE',  ( 10.55878694030978338, -4.980312522622296179, -5.017513730241772052 ) ) ;
#4278=CARTESIAN_POINT ( 'NONE',  ( 10.45625805961999966, -3.661873208228000109, -9.317463915629002003 ) ) ;
#4279=DIRECTION ( 'NONE',  ( 0.000000000000000000, 1.000000000000000000, 0.000000000000000000 ) ) ;
#4283=CARTESIAN_POINT ( 'NONE',  ( 7.800894438721999613, -3.218815632501999868, 6.398977300879999497 ) ) ;
#4288=FACE_OUTER_BOUND ( 'NONE', #49751, .T. ) ;
#4297=LINE ( 'NONE', #19353, #52711 ) ;
#4298=VECTOR ( 'NONE', #50442, 999.9999999999998863 ) ;
#4303=ORIENTED_EDGE ( 'NONE', *, *, #42774, .F. ) ;
#4314=CARTESIAN_POINT ( 'NONE',  ( 9.879728264518837122, -5.547209490050214242, -8.349578818441225181 ) ) ;
#4316=CARTESIAN_POINT ( 'NONE',  ( 7.966460921982604582, -5.180256874905444064, 8.180071673469297977 ) ) ;
#4320=CARTESIAN_POINT ( 'NONE',  ( 10.97075054419999951, -2.648517896406999750, -6.788869136079999755 ) ) ;
#4335=CARTESIAN_POINT ( 'NONE',  ( 11.07245484343000008, -2.731907627704000419, 5.080881421444000345 ) ) ;
#4337=CARTESIAN_POINT ( 'NONE',  ( 10.38593211929999960, -3.066808974315999858, -4.600377780681998985 ) ) ;
#4341=PLANE ( 'NONE',  #4199 ) ;
#4342=LINE ( 'NONE', #26720, #38599 ) ;
#4365=CARTESIAN_POINT ( 'NONE',  ( 9.351499161061999743, -4.821938821912000073, 8.950150764319998231 ) ) ;
#4368=CARTESIAN_POINT ( 'NONE',  ( 8.251331853209000755, -5.773185758034999893, 7.141496747382000798 ) ) ;
#4374=LINE ( 'NONE', #64132, #751 ) ;
#4377=CARTESIAN_POINT ( 'NONE',  ( 9.305875415870998424, -4.945293979885000191, 9.077881967919999795 ) ) ;
#4381=CARTESIAN_POINT ( 'NONE',  ( 10.77434462036999818, -4.612888200890999713, -8.898797372219998891 ) ) ;
#4382=B_SPLINE_CURVE_WITH_KNOTS ( 'NONE', 3,
 ( #22265, #27874, #22609, #43952 ),
 .UNSPECIFIED., .F., .F.,
 ( 4, 4 ),
 ( 0.000000000000000000, 1.000000000000000000 ),
 .UNSPECIFIED. ) ;
#4384=ORIENTED_EDGE ( 'NONE', *, *, #8853, .T. ) ;
#4387=LINE ( 'NONE', #68705, #43834 ) ;
#4389=ADVANCED_FACE ( 'NONE', ( #32309 ), #33609, .T. ) ;
#4392=ADVANCED_FACE ( 'NONE', ( #31612 ), #4587, .F. ) ;
#4411=CARTESIAN_POINT ( 'NONE',  ( 7.308879440377999970, -4.847802017252000439, 9.065364004483999594 ) ) ;
#4412=VECTOR ( 'NONE', #32580, 1000.000000000000000 ) ;
#4424=CARTESIAN_POINT ( 'NONE',  ( 7.512831853207000421, -5.524126964933000927, 6.910359834012999691 ) ) ;
#4427=EDGE_LOOP ( 'NONE', ( #55944, #27432, #8692, #55742, #47714 ) ) ;
#4434=DIRECTION ( 'NONE',  ( 0.7071067811865475727, 0.7071067811865475727, 0.000000000000000000 ) ) ;
#4441=CARTESIAN_POINT ( 'NONE',  ( 8.283766169413352642, -4.844672635244611669, 9.020389543242568919 ) ) ;
#4443=VERTEX_POINT ( 'NONE', #21450 ) ;
#4444=LINE ( 'NONE', #36621, #57812 ) ;
#4451=DIRECTION ( 'NONE',  ( 0.000000000000000000, -1.000000000000000000, 0.000000000000000000 ) ) ;
#4454=CYLINDRICAL_SURFACE ( 'NONE', #8545, 1.250000000000000000 ) ;
#4460=CARTESIAN_POINT ( 'NONE',  ( 7.711433059622000208, -5.797088532631000213, 8.340479314546998424 ) ) ;
#4476=FILL_AREA_STYLE_COLOUR ( '', #41883 ) ;
#4485=ORIENTED_EDGE ( 'NONE', *, *, #67630, .T. ) ;
#4486=CARTESIAN_POINT ( 'NONE',  ( 8.625477980836398828, -4.987582323328632938, -6.571819886621350193 ) ) ;
#4499=CARTESIAN_POINT ( 'NONE',  ( 9.208690252286228173, -2.678874286390015680, 7.777716411846479438 ) ) ;
#4519=EDGE_CURVE ( 'NONE', #51180, #39230, #15117, .T. ) ;
#4522=CARTESIAN_POINT ( 'NONE',  ( 11.01895424672924584, -5.424779607849700369, 7.028465765784092767 ) ) ;
#4523=CARTESIAN_POINT ( 'NONE',  ( 7.448644353207000357, -4.628942671846000501, 5.991663889842000046 ) ) ;
#4526=CARTESIAN_POINT ( 'NONE',  ( 10.12125395348325441, -3.646954034496651786, 8.849054885471268506 ) ) ;
#4527=CARTESIAN_POINT ( 'NONE',  ( 10.64557055961999943, -2.988935764546999607, -5.952339209104000162 ) ) ;
#4528=CARTESIAN_POINT ( 'NONE',  ( 7.594155103570124687, -4.422461687346440407, 5.812547095734072577 ) ) ;
#4532=CARTESIAN_POINT ( 'NONE',  ( 10.27427156480999848, -4.600000212792999754, 4.944156960788000710 ) ) ;
#4537=VERTEX_POINT ( 'NONE', #51139 ) ;
#4540=CARTESIAN_POINT ( 'NONE',  ( 10.98041052569057285, -5.205274417407212084, 6.713913193645853816 ) ) ;
#4555=CARTESIAN_POINT ( 'NONE',  ( 10.13340376756999994, -5.653635692335999607, 6.501829690795999817 ) ) ;
#4556=ADVANCED_FACE ( 'NONE', ( #24568 ), #14640, .F. ) ;
#4568=DIRECTION ( 'NONE',  ( 0.8843050095428930391, 0.1786786001429985227, 0.4313682973379965868 ) ) ;
#4571=CARTESIAN_POINT ( 'NONE',  ( 10.80169466977000070, -3.998196228428999355, 9.431543037543999475 ) ) ;
#4579=CARTESIAN_POINT ( 'NONE',  ( 10.15903154954000165, -4.166415630773999901, 9.114167874391000623 ) ) ;
#4586=CARTESIAN_POINT ( 'NONE',  ( 9.795911616191999016, -5.239375073306999475, -6.095351682555999240 ) ) ;
#4587=CONICAL_SURFACE ( 'NONE', #20220, 1.199999999294000030, 0.7853981633972997312 ) ;
#4590=B_SPLINE_CURVE_WITH_KNOTS ( 'NONE', 3,
 ( #9352, #8683, #24762, #46776, #68081, #4797, #26140, #46088, #19517, #40837 ),
 .UNSPECIFIED., .F., .F.,
 ( 4, 1, 1, 1, 1, 1, 1, 4 ),
 ( 0.000000000000000000, 0.03621323782862000129, 0.1968444277449999946, 0.3574756176613000380, 0.5181068075775999704, 0.6787379974939999894, 0.8393691874102999773, 1.000000000000000000 ),
 .UNSPECIFIED. ) ;
#4595=CARTESIAN_POINT ( 'NONE',  ( 11.04782425406999913, -5.235403588978999601, 5.041461677707999911 ) ) ;
#4601=CARTESIAN_POINT ( 'NONE',  ( 9.385788300200999856, -4.980873770300999759, 6.433336655958999728 ) ) ;
#4612=CARTESIAN_POINT ( 'NONE',  ( 9.804518107930274340, -2.650217341019555306, -7.676659142575331884 ) ) ;
#4619=CARTESIAN_POINT ( 'NONE',  ( 9.282558421712998609, -4.950980172046000050, -5.959730545597000884 ) ) ;
#4620=CARTESIAN_POINT ( 'NONE',  ( 11.11478185320999934, -2.548220588762000194, -8.356740464335999263 ) ) ;
#4646=VERTEX_POINT ( 'NONE', #282 ) ;
#4657=CARTESIAN_POINT ( 'NONE',  ( 8.008165174986327628, -4.679062738103563213, 8.679582621499569939 ) ) ;
#4661=CARTESIAN_POINT ( 'NONE',  ( 10.42081395746000005, -2.488448635474999726, -7.717895569088000229 ) ) ;
#4665=CARTESIAN_POINT ( 'NONE',  ( 10.94076550314999885, -5.140765503144999471, -6.571291218949999902 ) ) ;
#4666=CARTESIAN_POINT ( 'NONE',  ( 10.36409408021999923, -4.600000090830000943, -4.954046131267999087 ) ) ;
#4672=CARTESIAN_POINT ( 'NONE',  ( 7.861945368778997079, -2.855203060631998024, 6.787771340568003353 ) ) ;
#4678=CARTESIAN_POINT ( 'NONE',  ( 10.55991645936999923, -5.094263939633999705, 6.075409946530999861 ) ) ;
#4685=CIRCLE ( 'NONE', #43789, 0.8000000000000000444 ) ;
#4694=CARTESIAN_POINT ( 'NONE',  ( 10.90000000000000036, -5.283926297003000094, 7.082827057608000132 ) ) ;
#4696=ORIENTED_EDGE ( 'NONE', *, *, #39099, .T. ) ;
#4701=CARTESIAN_POINT ( 'NONE',  ( 5.699999999579000054, -0.3000000004212000082, -9.662944680462999258 ) ) ;
#4705=CARTESIAN_POINT ( 'NONE',  ( 11.02445830383999947, -3.404091099119999519, 5.822494319281999786 ) ) ;
#4708=CARTESIAN_POINT ( 'NONE',  ( 7.518870559622000016, -3.206365290996999740, 5.681739161071000410 ) ) ;
#4717=CARTESIAN_POINT ( 'NONE',  ( 10.62197618263000010, -5.779779175739000685, 7.256573549370999743 ) ) ;
#4718=EDGE_CURVE ( 'NONE', #11189, #64219, #42799, .T. ) ;
#4721=B_SPLINE_CURVE_WITH_KNOTS ( 'NONE', 3,
 ( #36185, #57159, #9957, #25691 ),
 .UNSPECIFIED., .F., .F.,
 ( 4, 4 ),
 ( 0.000000000000000000, 1.000000000000000000 ),
 .UNSPECIFIED. ) ;
#4739=DIRECTION ( 'NONE',  ( 1.000000000000000000, 0.000000000000000000, 0.000000000000000000 ) ) ;
#4746=CARTESIAN_POINT ( 'NONE',  ( 9.350151960951233576, -5.734349002094055514, -7.726429600794550545 ) ) ;
#4754=CARTESIAN_POINT ( 'NONE',  ( 7.475043146792000215, -3.276313010012999793, 5.841993238691999935 ) ) ;
#4765=CARTESIAN_POINT ( 'NONE',  ( 7.454683059621999952, -2.138201851198999748, 6.814774777484000623 ) ) ;
#4769=EDGE_LOOP ( 'NONE', ( #21350, #13848, #33094, #56494, #30396 ) ) ;
#4770=B_SPLINE_CURVE_WITH_KNOTS ( 'NONE', 3,
 ( #65749, #50028, #44792, #61546, #23455, #12977, #45474, #34299, #40562, #29062 ),
 .UNSPECIFIED., .F., .F.,
 ( 4, 2, 2, 2, 4 ),
 ( 0.7033810150431129005, 0.7404583881627235797, 0.7775357612823343700, 0.8516905075215559506, 1.000000000000000000 ),
 .UNSPECIFIED. ) ;
#4780=CARTESIAN_POINT ( 'NONE',  ( 10.69031285273999821, -5.903020122789000013, 7.830708506196000229 ) ) ;
#4781=DIRECTION ( 'NONE',  ( -0.7071067811866525998, 0.000000000000000000, -0.7071067811864425456 ) ) ;
#4785=CARTESIAN_POINT ( 'NONE',  ( 8.254586106814789659, -5.344701609173532653, 8.603696000269675181 ) ) ;
#4797=CARTESIAN_POINT ( 'NONE',  ( 10.48419913891000022, -2.939341339380999507, -4.699609182310999778 ) ) ;
#4809=CARTESIAN_POINT ( 'NONE',  ( 9.123558059623999128, -5.558929022707999046, 6.272984818914999927 ) ) ;
#4833=CARTESIAN_POINT ( 'NONE',  ( 10.32322128467999889, -4.600000125420001140, -4.621083553505000552 ) ) ;
#4837=VECTOR ( 'NONE', #30973, 1000.000000000000000 ) ;
#4847=CARTESIAN_POINT ( 'NONE',  ( 9.167130263679302615, -2.992093955605813260, 8.398819266328139577 ) ) ;
#4859=AXIS2_PLACEMENT_3D ( 'NONE', #9053, #2782, #36313 ) ;
#4865=EDGE_CURVE ( 'NONE', #67307, #56244, #22790, .T. ) ;
#4870=CARTESIAN_POINT ( 'NONE',  ( 8.989144353209001181, -5.284133759825000887, 6.489273023403000273 ) ) ;
#4874=CARTESIAN_POINT ( 'NONE',  ( 10.56984555961999916, -2.152868447761999704, -7.425101130468999777 ) ) ;
#4875=CARTESIAN_POINT ( 'NONE',  ( 7.570875225191677771, -3.932046780718525980, 5.759964130382589254 ) ) ;
#4885=B_SPLINE_SURFACE_WITH_KNOTS ( 'NONE', 3, 3, ( 
 ( #38024, #31417, #58666, #68450, #25820, #64242, #36661, #27203, #15333, #57982, #16357, #52733, #11118, #5180, #10767, #5525, #32451, #48524, #633, #21942, #28945, #43977, #60047, #28591, #12500, #13204, #61084, #65627, #43632, #60735, #6900, #38374, #33833, #22292, #64926 ),
 ( #18097, #28236, #17396, #44329, #39416, #1664, #27900, #980, #17042, #6557, #1316, #44675, #49209, #38725, #22633, #59698, #49552, #65283, #34178, #7250, #12157, #33488, #49903, #54801, #45013, #22981, #66318, #17752, #55496, #18441, #2012, #7596, #50250, #39072, #55147 ),
 ( #60395, #23334, #27545, #39766, #2352, #23675, #12849, #11800, #65969, #34532, #6203, #48872, #33139, #54455, #34864, #45356, #3712, #66665, #2698, #41477, #19809, #45698, #61429, #25049, #4055, #14907, #67007, #61765, #56871, #56180, #25390, #3036, #35213, #62786, #9304 ),
 ( #46036, #24022, #41139, #56525, #18784, #62108, #40115, #13545, #13883, #24367, #46728, #30645, #51280, #14227, #8630, #8291, #51616, #40438, #68034, #40783, #29636, #20150, #7945, #55841, #51954, #24712, #35554, #29978, #29282, #50596, #50939, #19116, #3375, #67341, #19463 ) ),
 .UNSPECIFIED., .F., .F., .F.,
 ( 4, 4 ),
 ( 4, 1, 1, 1, 1, 1, 1, 1, 1, 1, 1, 1, 1, 1, 1, 1, 1, 1, 1, 1, 1, 1, 1, 1, 1, 1, 1, 1, 1, 1, 1, 1, 4 ),
 ( -0.1039086239011999951, 1.103908623900999864 ),
 ( 0.1942321073450000157, 0.2199060843169000079, 0.2455800612886999967, 0.2712540382605999612, 0.2969280152323999777, 0.3226019922043000254, 0.3482759691761000420, 0.3739499461479999787, 0.3996239231197999953, 0.4252979000916999874, 0.4509718770635000040, 0.4766458540353999962, 0.5023198310072000128, 0.5279938079791000050, 0.5536677849509000771, 0.5793417619227999582, 0.6050157388945999193, 0.6306897158665000225, 0.6563636928382999836, 0.6820376698101999757, 0.7077116467820000478, 0.7333856237539000400, 0.7590596007256998901, 0.7847335776975999933, 0.8104075546693999543, 0.8360815316413000575, 0.8617555086131000186, 0.8874294855850000108, 0.9131034625568000829, 0.9387774395286999640, 0.9644514165004999251, 0.9901253934722999972, 1.015799370444000038 ),
 .UNSPECIFIED. ) ;
#4898=ORIENTED_EDGE ( 'NONE', *, *, #51983, .F. ) ;
#4904=CARTESIAN_POINT ( 'NONE',  ( 9.834153701540001791, -5.173926576843999925, 8.813045240277000758 ) ) ;
#4929=CARTESIAN_POINT ( 'NONE',  ( 9.848732933287999813, -2.769734897491000325, 6.441850735262000249 ) ) ;
#4952=EDGE_CURVE ( 'NONE', #46692, #51958, #28455, .T. ) ;
#4958=ADVANCED_FACE ( 'NONE', ( #17258 ), #37892, .T. ) ;
#4961=AXIS2_PLACEMENT_3D ( 'NONE', #2587, #11691, #23917 ) ;
#4971=CARTESIAN_POINT ( 'NONE',  ( 11.06205805961999999, -2.154403720901000518, -7.605897512385999981 ) ) ;
#4972=CARTESIAN_POINT ( 'NONE',  ( 9.132625033077360399, -2.794592352501091170, 8.206332652464567445 ) ) ;
#4975=CARTESIAN_POINT ( 'NONE',  ( 8.316694573732000606, -2.898380360490000029, 6.611503418275999522 ) ) ;
#4977=EDGE_LOOP ( 'NONE', ( #460, #10966, #17291, #3407, #55069 ) ) ;
#5002=ADVANCED_FACE ( 'NONE', ( #50119 ), #39982, .F. ) ;
#5003=CARTESIAN_POINT ( 'NONE',  ( 8.461732853997688153, -5.351516129092861895, 7.263730654262129605 ) ) ;
#5009=CARTESIAN_POINT ( 'NONE',  ( 7.000000000000000000, -1.250000000000000000, 0.000000000000000000 ) ) ;
#5013=CARTESIAN_POINT ( 'NONE',  ( 10.99693800072000016, -2.980603239157999962, -6.418614998350999912 ) ) ;
#5023=CARTESIAN_POINT ( 'NONE',  ( 10.27668195243999882, -3.417616861023999864, 5.003889090935000006 ) ) ;
#5024=CARTESIAN_POINT ( 'NONE',  ( 7.684934563448005740, -2.928065616737000720, 6.508603912219004251 ) ) ;
#5025=ORIENTED_EDGE ( 'NONE', *, *, #34586, .F. ) ;
#5027=CARTESIAN_POINT ( 'NONE',  ( 10.41114191524999910, -3.147777059971999414, -4.883851472541000049 ) ) ;
#5028=CARTESIAN_POINT ( 'NONE',  ( 9.492891187585001944, -4.474581801608000120, -6.279517683005999551 ) ) ;
#5030=CARTESIAN_POINT ( 'NONE',  ( 10.89874164595999950, -2.834836218627000193, 9.088455567997000273 ) ) ;
#5033=ADVANCED_FACE ( 'NONE', ( #50809 ), #67213, .T. ) ;
#5042=PLANE ( 'NONE',  #29236 ) ;
#5045=CARTESIAN_POINT ( 'NONE',  ( 10.16052890781999984, -2.899999999999999911, -6.152188490330000370 ) ) ;
#5046=CARTESIAN_POINT ( 'NONE',  ( 9.461621083092298434, -5.351423275947231772, 7.263649724570567123 ) ) ;
#5047=DIRECTION ( 'NONE',  ( 0.000000000000000000, -0.1333333333333049375, -0.9910712498212376209 ) ) ;
#5048=CARTESIAN_POINT ( 'NONE',  ( 8.616332382228000242, -2.832433105983000132, -6.822293595522999077 ) ) ;
#5050=CARTESIAN_POINT ( 'NONE',  ( 5.700000000000000178, 0.5292307692307999245, 2.083846153846000249 ) ) ;
#5059=CARTESIAN_POINT ( 'NONE',  ( 9.465112865370999273, -2.290047720994000002, 6.601709978349000529 ) ) ;
#5061=EDGE_LOOP ( 'NONE', ( #28240, #68949, #46639 ) ) ;
#5063=CARTESIAN_POINT ( 'NONE',  ( 9.149956853208999874, -4.175914961544999748, 5.699510287082000026 ) ) ;
#5072=CARTESIAN_POINT ( 'NONE',  ( 9.318721994369999706, -2.755032632138999737, 8.795122807847999269 ) ) ;
#5080=CARTESIAN_POINT ( 'NONE',  ( 9.814967517147769271, -2.649990781018497721, -7.499998108648967765 ) ) ;
#5090=EDGE_LOOP ( 'NONE', ( #26341, #45735, #52205, #23000 ) ) ;
#5106=CARTESIAN_POINT ( 'NONE',  ( 7.795980646793000624, -3.164807285701999984, 9.104732190648000767 ) ) ;
#5117=CARTESIAN_POINT ( 'NONE',  ( 7.802019353206999241, -5.638700495537999124, 8.266402903491000487 ) ) ;
#5134=CARTESIAN_POINT ( 'NONE',  ( 7.835154761361642350, -4.943139372678011512, 6.476578150245067000 ) ) ;
#5137=CARTESIAN_POINT ( 'NONE',  ( 8.420824285387190855, -2.370222298025555840, 8.108356380490343795 ) ) ;
#5149=FACE_OUTER_BOUND ( 'NONE', #66349, .T. ) ;
#5162=CARTESIAN_POINT ( 'NONE',  ( 8.096558059622999792, -5.061720701958000390, 5.824087910811999613 ) ) ;
#5164=VERTEX_POINT ( 'NONE', #23888 ) ;
#5180=CARTESIAN_POINT ( 'NONE',  ( 10.44807121817999906, -3.684978196963999864, -6.173109031625999776 ) ) ;
#5213=LINE ( 'NONE', #1346, #44356 ) ;
#5220=CARTESIAN_POINT ( 'NONE',  ( 10.37026726325999881, -5.571557883540000589, 7.748386351620999868 ) ) ;
#5221=CARTESIAN_POINT ( 'NONE',  ( 8.822980646795000936, -2.678334737187000325, 8.735278777293000729 ) ) ;
#5222=ORIENTED_EDGE ( 'NONE', *, *, #4952, .F. ) ;
#5224=CARTESIAN_POINT ( 'NONE',  ( 10.07963755961356611, -4.353097593134603649, 8.851823023821729919 ) ) ;
#5225=CARTESIAN_POINT ( 'NONE',  ( 11.09992055961999924, -2.373397911211000189, -6.776606350776999577 ) ) ;
#5226=CARTESIAN_POINT ( 'NONE',  ( 7.615409857907971869, -4.849756550714564796, 5.981625193514809702 ) ) ;
#5227=CARTESIAN_POINT ( 'NONE',  ( 7.933148997457998952, -5.167567567567999731, 6.822293592207000934 ) ) ;
#5254=CARTESIAN_POINT ( 'NONE',  ( 10.78089914631999946, -5.735295708369000600, 7.801561210335000496 ) ) ;
#5273=DIRECTION ( 'NONE',  ( 1.000000000000000000, 0.000000000000000000, 0.000000000000000000 ) ) ;
#5301=VERTEX_POINT ( 'NONE', #64025 ) ;
#5304=CYLINDRICAL_SURFACE ( 'NONE', #19821, 0.5000000000000002220 ) ;
#5312=CARTESIAN_POINT ( 'NONE',  ( 10.07763305961999833, -2.169024213715999849, -7.244986319234999250 ) ) ;
#5313=DIRECTION ( 'NONE',  ( 0.000000000000000000, 0.000000000000000000, -1.000000000000000000 ) ) ;
#5317=DIRECTION ( 'NONE',  ( -0.1570822244628920505, -0.9696804098390484628, 0.1872033053451904461 ) ) ;
#5332=DIRECTION ( 'NONE',  ( -1.000000000000000000, 0.000000000000000000, 0.000000000000000000 ) ) ;
#5334=AXIS2_PLACEMENT_3D ( 'NONE', #68706, #15583, #14211 ) ;
#5347=AXIS2_PLACEMENT_3D ( 'NONE', #53609, #25662, #46995 ) ;
#5355=VECTOR ( 'NONE', #66704, 1000.000000000000000 ) ;
#5359=CARTESIAN_POINT ( 'NONE',  ( 9.662447522843001124, -4.824180051339999942, -8.517611033492999084 ) ) ;
#5363=VECTOR ( 'NONE', #2822, 1000.000000000000227 ) ;
#5364=CARTESIAN_POINT ( 'NONE',  ( 10.20920446230533507, -2.899999999999999911, 6.662590550568703307 ) ) ;
#5366=DIRECTION ( 'NONE',  ( 0.000000000000000000, 0.000000000000000000, -1.000000000000000000 ) ) ;
#5372=CARTESIAN_POINT ( 'NONE',  ( 10.26574321149000113, -3.424277613364000050, 4.689150231930001134 ) ) ;
#5373=CARTESIAN_POINT ( 'NONE',  ( 8.335542453529990681, -2.897657451248000893, 6.653312621732999865 ) ) ;
#5375=VECTOR ( 'NONE', #6048, 1000.000000000000000 ) ;
#5377=CARTESIAN_POINT ( 'NONE',  ( 8.212419626809003503, -3.104180672527999896, 6.104185052591001082 ) ) ;
#5380=CARTESIAN_POINT ( 'NONE',  ( 10.77462219945999955, -5.575466189878000911, 8.682669263022999573 ) ) ;
#5390=ORIENTED_EDGE ( 'NONE', *, *, #57521, .F. ) ;
#5395=AXIS2_PLACEMENT_3D ( 'NONE', #48369, #5713, #57920 ) ;
#5408=CARTESIAN_POINT ( 'NONE',  ( 9.260912867475999732, -4.901383038209000453, 9.090314591495999963 ) ) ;
#5412=CARTESIAN_POINT ( 'NONE',  ( 8.727043146794999373, -3.882020254083999866, 5.870054788755000530 ) ) ;
#5421=CARTESIAN_POINT ( 'NONE',  ( 10.24961784311999935, -4.184221496660999406, 9.286877953065999947 ) ) ;
#5427=CARTESIAN_POINT ( 'NONE',  ( 11.03091694037999915, -5.020463882420000523, -6.601194361798000010 ) ) ;
#5434=DIRECTION ( 'NONE',  ( 0.000000000000000000, 0.000000000000000000, -1.000000000000000000 ) ) ;
#5438=ADVANCED_FACE ( 'NONE', ( #63081 ), #27081, .F. ) ;
#5456=EDGE_CURVE ( 'NONE', #23313, #40162, #37557, .T. ) ;
#5457=CARTESIAN_POINT ( 'NONE',  ( 9.079730646793999327, -5.421531391267000011, 6.381128921159999301 ) ) ;
#5468=CARTESIAN_POINT ( 'NONE',  ( 8.406105646793999853, -5.342173944271999986, 8.432314172168000610 ) ) ;
#5469=CARTESIAN_POINT ( 'NONE',  ( 9.209204462306566086, -2.899999999999999911, 6.662590550605525408 ) ) ;
#5479=CARTESIAN_POINT ( 'NONE',  ( 10.90000000000000036, 0.000000000000000000, 0.000000000000000000 ) ) ;
#5484=ORIENTED_EDGE ( 'NONE', *, *, #21431, .F. ) ;
#5485=LINE ( 'NONE', #15291, #54467 ) ;
#5487=CARTESIAN_POINT ( 'NONE',  ( 8.542538633423246708, -3.328189143799264560, 5.895772191526457817 ) ) ;
#5492=ORIENTED_EDGE ( 'NONE', *, *, #68210, .T. ) ;
#5495=CARTESIAN_POINT ( 'NONE',  ( 11.02452225494999993, -2.775477745048999800, -6.571291218949999902 ) ) ;
#5497=CARTESIAN_POINT ( 'NONE',  ( 10.49751479358649320, -3.288413547421944916, -9.126840212398633412 ) ) ;
#5504=ORIENTED_EDGE ( 'NONE', *, *, #22746, .F. ) ;
#5519=DIRECTION ( 'NONE',  ( 1.000000000000000000, 0.000000000000000000, 0.000000000000000000 ) ) ;
#5522=CARTESIAN_POINT ( 'NONE',  ( 10.43314899746000002, -5.167567567567999731, 6.822293592207000934 ) ) ;
#5525=CARTESIAN_POINT ( 'NONE',  ( 10.36950884864999978, -2.719121019997000399, -7.031782724641000293 ) ) ;
#5544=CARTESIAN_POINT ( 'NONE',  ( 9.910492310842998975, -4.686746084135999801, -9.174865097765998456 ) ) ;
#5551=CARTESIAN_POINT ( 'NONE',  ( 10.12947109217999930, -5.100000000000000533, 6.152188490330000370 ) ) ;
#5559=CARTESIAN_POINT ( 'NONE',  ( 10.03612181215999932, -3.011786236723999810, 8.746965724352000038 ) ) ;
#5560=CARTESIAN_POINT ( 'NONE',  ( 7.256081853207000165, -2.531197775378000170, 8.216705951490000714 ) ) ;
#5561=ORIENTED_EDGE ( 'NONE', *, *, #62115, .F. ) ;
#5564=CARTESIAN_POINT ( 'NONE',  ( 11.16750564679000135, -3.188702545307000147, -8.788667016604001958 ) ) ;
#5566=CARTESIAN_POINT ( 'NONE',  ( 7.806944751142499861, -4.387688527371611968, 9.195859951489477879 ) ) ;
#5567=CARTESIAN_POINT ( 'NONE',  ( 10.31167756636999933, -2.874479384703000129, 8.900026329558999194 ) ) ;
#5579=ORIENTED_EDGE ( 'NONE', *, *, #9211, .T. ) ;
#5580=CARTESIAN_POINT ( 'NONE',  ( 8.897673733342999824, -5.117431802241999783, -6.704256657961999544 ) ) ;
#5588=CARTESIAN_POINT ( 'NONE',  ( 11.09648096125000016, -3.099777420064000033, 6.097103007060000301 ) ) ;
#5595=EDGE_LOOP ( 'NONE', ( #31424, #2185, #56487, #65731, #52234, #3665 ) ) ;
#5598=DIRECTION ( 'NONE',  ( 0.000000000000000000, 1.000000000000000000, 0.000000000000000000 ) ) ;
#5618=B_SPLINE_CURVE_WITH_KNOTS ( 'NONE', 3,
 ( #51782, #9129, #50497, #65876 ),
 .UNSPECIFIED., .F., .F.,
 ( 4, 4 ),
 ( 0.000000000000000000, 1.000000000000000000 ),
 .UNSPECIFIED. ) ;
#5634=CYLINDRICAL_SURFACE ( 'NONE', #68139, 1.350000000000000089 ) ;
#5650=CARTESIAN_POINT ( 'NONE',  ( 10.97819314679000158, -5.476828481365000556, -7.128717489481000591 ) ) ;
#5661=DIRECTION ( 'NONE',  ( 0.000000000000000000, 1.000000000000000000, 0.000000000000000000 ) ) ;
#5671=FACE_OUTER_BOUND ( 'NONE', #53490, .T. ) ;
#5686=CARTESIAN_POINT ( 'NONE',  ( 11.12914445903999905, -3.083861519183999977, 8.586004431109000024 ) ) ;
#5689=ORIENTED_EDGE ( 'NONE', *, *, #29167, .T. ) ;
#5698=CARTESIAN_POINT ( 'NONE',  ( 10.64126772939999910, -2.258710642251000156, -6.863482599505999815 ) ) ;
#5712=ORIENTED_EDGE ( 'NONE', *, *, #17839, .T. ) ;
#5713=DIRECTION ( 'NONE',  ( 1.000000000000000000, 0.000000000000000000, 0.000000000000000000 ) ) ;
#5714=CARTESIAN_POINT ( 'NONE',  ( 9.471368011205999693, -2.030678448189000118, 7.549764202121000523 ) ) ;
#5717=CARTESIAN_POINT ( 'NONE',  ( 10.02990552045999983, -2.506467134554999809, 6.215414506835998942 ) ) ;
#5730=CARTESIAN_POINT ( 'NONE',  ( 9.475279990687656806, -5.350441389720279162, 7.499985493516659218 ) ) ;
#5742=CARTESIAN_POINT ( 'NONE',  ( 10.72520823780999955, -5.521647200017000934, 6.612992938078999572 ) ) ;
#5746=CARTESIAN_POINT ( 'NONE',  ( 7.416894353206999746, -3.448181789123000218, 9.222458996124998976 ) ) ;
#5749=DIRECTION ( 'NONE',  ( 0.000000000000000000, 0.8648648648648720183, 0.5020047465136825426 ) ) ;
#5750=VECTOR ( 'NONE', #54885, 1000.000000000000000 ) ;
#5756=CARTESIAN_POINT ( 'NONE',  ( 9.691080333872001518, -5.335644368206000188, 8.701217921043999937 ) ) ;
#5762=EDGE_CURVE ( 'NONE', #58951, #32339, #48176, .T. ) ;
#5774=EDGE_LOOP ( 'NONE', ( #62241, #18788, #62914, #11173, #11266, #8511, #43070, #55165 ) ) ;
#5780=CARTESIAN_POINT ( 'NONE',  ( 8.938754677014808081, -4.205681946487742628, -6.150054534049018251 ) ) ;
#5781=EDGE_CURVE ( 'NONE', #21446, #46265, #19822, .T. ) ;
#5783=CARTESIAN_POINT ( 'NONE',  ( 9.425619671860273385, -4.846212772418011738, -9.064231341663099073 ) ) ;
#5789=CARTESIAN_POINT ( 'NONE',  ( 8.630418146794999856, -5.808258301303999893, 7.446016267012000256 ) ) ;
#5800=ORIENTED_EDGE ( 'NONE', *, *, #15501, .T. ) ;
#5801=CARTESIAN_POINT ( 'NONE',  ( 9.385311019873999072, -4.135077143711000325, 9.175520401071999288 ) ) ;
#5803=B_SPLINE_CURVE_WITH_KNOTS ( 'NONE', 3,
 ( #19029, #40356, #61678, #4314, #13794, #35125, #32288, #42074, #57803, #31589 ),
 .UNSPECIFIED., .F., .F.,
 ( 4, 2, 2, 2, 4 ),
 ( 0.000000000000000000, 0.2500000000000000000, 0.5000000000000000000, 0.7500000000000000000, 1.000000000000000000 ),
 .UNSPECIFIED. ) ;
#5804=B_SPLINE_CURVE_WITH_KNOTS ( 'NONE', 3,
 ( #53262, #44169, #33326, #59881, #17236, #119, #48357, #32298, #64767, #6046, #21437, #54287 ),
 .UNSPECIFIED., .F., .F.,
 ( 4, 2, 2, 2, 2, 4 ),
 ( 0.000000000000000000, 0.2499999999999962252, 0.3749999999999931721, 0.4374999999999933942, 0.4999999999999935607, 1.000000000000000000 ),
 .UNSPECIFIED. ) ;
#5816=LINE ( 'NONE', #54058, #24182 ) ;
#5825=CARTESIAN_POINT ( 'NONE',  ( 8.409821582311559851, -2.468534350186054382, 8.326276327825025803 ) ) ;
#5830=ORIENTED_EDGE ( 'NONE', *, *, #50623, .F. ) ;
#5832=DIRECTION ( 'NONE',  ( -1.000000000000000000, 0.000000000000000000, 0.000000000000000000 ) ) ;
#5838=DIRECTION ( 'NONE',  ( -1.000000000000000000, 0.000000000000000000, 0.000000000000000000 ) ) ;
#5840=VERTEX_POINT ( 'NONE', #52097 ) ;
#5843=ORIENTED_EDGE ( 'NONE', *, *, #44982, .T. ) ;
#5846=CARTESIAN_POINT ( 'NONE',  ( 8.970944094206998898, -5.100000000000000533, 6.571291218949999902 ) ) ;
#5851=FACE_OUTER_BOUND ( 'NONE', #58259, .T. ) ;
#5882=CARTESIAN_POINT ( 'NONE',  ( 6.900000172107000118, -1.065814103639999922E-14, 1.505462421391999793E-13 ) ) ;
#5898=CARTESIAN_POINT ( 'NONE',  ( 10.85068991645999859, -4.478102922274999287, 6.162028334171000488 ) ) ;
#5899=CARTESIAN_POINT ( 'NONE',  ( 7.512831853207000421, -5.524126964933000927, 6.910359834012999691 ) ) ;
#5900=VERTEX_POINT ( 'NONE', #25191 ) ;
#5901=CARTESIAN_POINT ( 'NONE',  ( 8.203567189027999973, -3.399999998438999693, 6.139678690022999596 ) ) ;
#5905=CARTESIAN_POINT ( 'NONE',  ( 10.88760685321000032, -5.634843745609000365, -7.088991614236999972 ) ) ;
#5906=CARTESIAN_POINT ( 'NONE',  ( 7.876919724916979781, -2.918260083478235067, 8.873651148443707726 ) ) ;
#5908=CARTESIAN_POINT ( 'NONE',  ( 10.02990552045999983, -2.506467134554999809, 6.215414506835998942 ) ) ;
#5924=CARTESIAN_POINT ( 'NONE',  ( 8.689254440380000943, -2.550228841911000188, 7.666975032000999946 ) ) ;
#5927=DIRECTION ( 'NONE',  ( 0.000000000000000000, 0.000000000000000000, -1.000000000000000000 ) ) ;
#5932=CARTESIAN_POINT ( 'NONE',  ( 10.50244460374000077, -2.268915328469999881, 7.824865002012999504 ) ) ;
#5956=CARTESIAN_POINT ( 'NONE',  ( 10.87522165821000009, -4.831071966430999787, 6.312786525516999703 ) ) ;
#5986=VECTOR ( 'NONE', #56872, 1000.000000000000000 ) ;
#5987=CARTESIAN_POINT ( 'NONE',  ( 9.669098047358048120, -4.353250594943018470, -8.814528502301756774 ) ) ;
#5993=CARTESIAN_POINT ( 'NONE',  ( 11.09178064679000109, -4.578543110806999827, -8.908602356389000221 ) ) ;
#6003=VERTEX_POINT ( 'NONE', #33545 ) ;
#6015=CARTESIAN_POINT ( 'NONE',  ( 10.11858840337999865, -3.393395892949000014, -5.921999462319999630 ) ) ;
#6025=CARTESIAN_POINT ( 'NONE',  ( 10.48744998751060997, -3.030310408214976992, 5.007827882781265671 ) ) ;
#6029=CARTESIAN_POINT ( 'NONE',  ( 10.96207173348999930, -5.399846879528999999, 7.743266618618998898 ) ) ;
#6041=CARTESIAN_POINT ( 'NONE',  ( 10.09133114265999964, -2.216726401468000152, -8.007130485478999304 ) ) ;
#6042=EDGE_CURVE ( 'NONE', #7868, #15904, #51391, .T. ) ;
#6045=LINE ( 'NONE', #59190, #25463 ) ;
#6046=CARTESIAN_POINT ( 'NONE',  ( 8.672328646360149662, -3.200842352561755533, -6.403885667220094113 ) ) ;
#6048=DIRECTION ( 'NONE',  ( 0.000000000000000000, -1.000000000000000000, 0.000000000000000000 ) ) ;
#6058=CARTESIAN_POINT ( 'NONE',  ( 9.595487457706001422, -3.928425191288000384, 5.531324308465000783 ) ) ;
#6061=CARTESIAN_POINT ( 'NONE',  ( 10.71256247620999957, -5.951803124515000043, 7.233045248871000865 ) ) ;
#6062=CARTESIAN_POINT ( 'NONE',  ( 9.987419771736607998, -2.445504403440184937, 6.696380856873024534 ) ) ;
#6065=B_SPLINE_CURVE_WITH_KNOTS ( 'NONE', 3,
 ( #31153, #37072, #41285, #52455, #3864, #15052, #58384, #9804, #25548, #47220 ),
 .UNSPECIFIED., .F., .F.,
 ( 4, 1, 1, 1, 1, 1, 1, 4 ),
 ( 0.000000000000000000, 0.02409300149743000274, 0.1867443091173000003, 0.3493956167372000432, 0.5120469243570999751, 0.6746982319770000736, 0.8373495395968999500, 1.000000000000000000 ),
 .UNSPECIFIED. ) ;
#6075=DIRECTION ( 'NONE',  ( 0.000000000000000000, 0.3146293386371170064, -0.9492146118074512584 ) ) ;
#6085=ORIENTED_EDGE ( 'NONE', *, *, #11505, .F. ) ;
#6089=EDGE_LOOP ( 'NONE', ( #41646, #5579, #10126, #53743 ) ) ;
#6091=CARTESIAN_POINT ( 'NONE',  ( 9.832537864288001472, -2.899999999999999911, 6.571291218949999902 ) ) ;
#6098=CARTESIAN_POINT ( 'NONE',  ( 8.191498616105999275, -3.399962740672999750, 6.146646623957999545 ) ) ;
#6100=CARTESIAN_POINT ( 'NONE',  ( 10.31668414895000119, -3.819528725844000494, 6.062183754159999438 ) ) ;
#6103=AXIS2_PLACEMENT_3D ( 'NONE', #34008, #1150, #27727 ) ;
#6105=CARTESIAN_POINT ( 'NONE',  ( 10.06949314679000018, -4.910373174915999783, -8.649593977693999847 ) ) ;
#6122=CARTESIAN_POINT ( 'NONE',  ( 10.46432358320999967, -2.042767395367000027, 7.723698102088000006 ) ) ;
#6131=CARTESIAN_POINT ( 'NONE',  ( 9.625409048293999348, -2.899999999999999911, -6.226580113766999602 ) ) ;
#6133=CARTESIAN_POINT ( 'NONE',  ( 8.181105646794000208, -5.485781663882000281, 8.532068390166999805 ) ) ;
#6143=ORIENTED_EDGE ( 'NONE', *, *, #34995, .T. ) ;
#6144=CARTESIAN_POINT ( 'NONE',  ( 7.673644353206999114, -4.696237245142999228, 5.830277424166999900 ) ) ;
#6155=CARTESIAN_POINT ( 'NONE',  ( 10.90000000000000036, 0.000000000000000000, 0.000000000000000000 ) ) ;
#6157=CARTESIAN_POINT ( 'NONE',  ( 7.955265382045282330, -4.958437936411385749, 6.436898865497720834 ) ) ;
#6162=CARTESIAN_POINT ( 'NONE',  ( 8.414809249528957480, -2.419867401190203715, 8.226612844550492909 ) ) ;
#6165=DIRECTION ( 'NONE',  ( -1.000000000000000000, -5.329070518371000199E-14, 3.552713678914000343E-14 ) ) ;
#6174=CARTESIAN_POINT ( 'NONE',  ( 8.871554213457001126, -3.399999843100999897, -6.206435837692999336 ) ) ;
#6178=AXIS2_PLACEMENT_3D ( 'NONE', #8543, #66576, #24627 ) ;
#6187=B_SPLINE_SURFACE_WITH_KNOTS ( 'NONE', 3, 3, ( 
 ( #56156, #4377, #14204, #25028, #45334, #8948, #40094, #57520, #46012, #66982, #66644, #14882, #30621, #51933, #19785, #61740, #25368, #46705, #56501, #30289, #36204, #18764, #13525, #45677, #50914, #19094, #13860, #3355, #35188, #67320, #51592, #19438, #3688, #41112, #62425 ),
 ( #14546, #32348, #42148, #5072, #64135, #31312, #63098, #47044, #15224, #5756, #58907, #15573, #10660, #26410, #48072, #68697, #52624, #36549, #5421, #68347, #26061, #9976, #32007, #42827, #4717, #20465, #47390, #16597, #42486, #41794, #20811, #21159, #37572, #48413, #58216 ),
 ( #519, #57875, #16249, #63451, #53663, #15905, #11011, #63796, #36901, #10320, #31653, #52975, #47737, #21836, #27098, #53998, #43167, #37237, #21493, #37922, #32685, #64473, #58554, #69051, #59241, #53321, #11347, #25712, #26759, #176, #38265, #65518, #7145, #34073, #28482 ),
 ( #43865, #11690, #33030, #65866, #60631, #16932, #44908, #49800, #12743, #6793, #66210, #60979, #59589, #28130, #1907, #39656, #17288, #13091, #54342, #60288, #18332, #34426, #6100, #38615, #27439, #6445, #59935, #48761, #867, #39308, #23228, #22183, #12046, #54694, #43523 ) ),
 .UNSPECIFIED., .F., .F., .F.,
 ( 4, 4 ),
 ( 4, 1, 1, 1, 1, 1, 1, 1, 1, 1, 1, 1, 1, 1, 1, 1, 1, 1, 1, 1, 1, 1, 1, 1, 1, 1, 1, 1, 1, 1, 1, 1, 4 ),
 ( -0.1039086239011999951, 1.103908623900999864 ),
 ( -0.01933701211302999920, 0.01208563257065999909, 0.04350827725433999843, 0.07493092193802000645, 0.1063535666217000075, 0.1377762113054000204, 0.1691988559891000055, 0.2006215006727000150, 0.2320441453564000001, 0.2634667900400999851, 0.2948894347238000258, 0.3263120794074999553, 0.3577347240911999959, 0.3891573687748000054, 0.4205800134584999905, 0.4520026581421999756, 0.4834253028259000162, 0.5148479475096000568, 0.5462705921932000663, 0.5776932368768999959, 0.6091158815606000365, 0.6405385262443000771, 0.6719611709280000067, 0.7033838156117000473, 0.7348064602953000568, 0.7662291049789999864, 0.7976517496627000270, 0.8290743943464000676, 0.8604970390300999972, 0.8919196837138000378, 0.9233423283974000473, 0.9547649730810999769, 0.9861876177648000175 ),
 .UNSPECIFIED. ) ;
#6196=EDGE_LOOP ( 'NONE', ( #34226, #35721, #40011 ) ) ;
#6198=ORIENTED_EDGE ( 'NONE', *, *, #4070, .T. ) ;
#6203=CARTESIAN_POINT ( 'NONE',  ( 10.74708735964999917, -5.603138702306000418, -6.963343193308999979 ) ) ;
#6210=VERTEX_POINT ( 'NONE', #36287 ) ;
#6241=CARTESIAN_POINT ( 'NONE',  ( 10.46085355684000007, -5.403406918566000527, 7.721809917403000156 ) ) ;
#6242=CARTESIAN_POINT ( 'NONE',  ( 8.449245559625000013, -5.458705123429999695, 7.456451825584000659 ) ) ;
#6246=CARTESIAN_POINT ( 'NONE',  ( 11.00119435320999983, -4.640445114785999969, -9.059317673956000405 ) ) ;
#6247=CARTESIAN_POINT ( 'NONE',  ( 7.817505239956299867, -4.153452198738197154, 9.248890255915149794 ) ) ;
#6248=CARTESIAN_POINT ( 'NONE',  ( 10.46432358320999967, -2.042767395367000027, 7.723698102088000006 ) ) ;
#6258=ORIENTED_EDGE ( 'NONE', *, *, #33730, .T. ) ;
#6266=CARTESIAN_POINT ( 'NONE',  ( 8.625066940379999991, -3.117370956513999758, 8.662188901935000018 ) ) ;
#6269=CARTESIAN_POINT ( 'NONE',  ( 10.16052890781999984, -2.899999999999999911, -6.152188490330000370 ) ) ;
#6294=ORIENTED_EDGE ( 'NONE', *, *, #29067, .T. ) ;
#6298=CARTESIAN_POINT ( 'NONE',  ( 9.323728576950999880, -3.947350124452999598, 6.051857392047999440 ) ) ;
#6305=FACE_OUTER_BOUND ( 'NONE', #29626, .T. ) ;
#6325=VECTOR ( 'NONE', #15902, 1000.000000000000000 ) ;
#6335=CARTESIAN_POINT ( 'NONE',  ( 10.73615685320999980, -3.078046833211999900, -6.088743704655001032 ) ) ;
#6339=CARTESIAN_POINT ( 'NONE',  ( 8.679055905797000037, -2.899999999999999911, 6.571291218949999902 ) ) ;
#6359=CARTESIAN_POINT ( 'NONE',  ( 10.46009514222999925, -2.565650894080999667, -6.975682682930000489 ) ) ;
#6365=VERTEX_POINT ( 'NONE', #46441 ) ;
#6371=CARTESIAN_POINT ( 'NONE',  ( 9.625489929093001606, -3.134630999349000025, 8.626959345509000343 ) ) ;
#6384=CARTESIAN_POINT ( 'NONE',  ( 10.94349328348999961, -3.081618981425999770, -8.919377696680001577 ) ) ;
#6407=CARTESIAN_POINT ( 'NONE',  ( 11.15982711745999900, -5.578228817597000955, 8.067792329320999656 ) ) ;
#6413=CARTESIAN_POINT ( 'NONE',  ( 10.90453766415000025, -2.900310535872000273, -5.130381900875999435 ) ) ;
#6419=CARTESIAN_POINT ( 'NONE',  ( 8.225195096046189036, -2.649880853682571313, 7.500010424662522546 ) ) ;
#6421=CARTESIAN_POINT ( 'NONE',  ( 7.474999999999999645, -5.349999999999999645, 7.500000000000000000 ) ) ;
#6432=ORIENTED_EDGE ( 'NONE', *, *, #37865, .T. ) ;
#6445=CARTESIAN_POINT ( 'NONE',  ( 10.50286331871000023, -5.158900740613000302, 8.369962360110999811 ) ) ;
#6465=ORIENTED_EDGE ( 'NONE', *, *, #23404, .F. ) ;
#6471=CARTESIAN_POINT ( 'NONE',  ( 10.77462219945999955, -5.575466189878000911, 8.682669263022999573 ) ) ;
#6494=ORIENTED_EDGE ( 'NONE', *, *, #37135, .T. ) ;
#6495=CARTESIAN_POINT ( 'NONE',  ( 8.674245559624999657, -5.983034890242000081, 7.440798487724999966 ) ) ;
#6504=EDGE_LOOP ( 'NONE', ( #24749, #45634, #33512, #60016, #12943, #18412, #32841, #42428, #61785, #47821, #14978, #38719, #41181, #45076, #20857, #49528, #12153, #33659, #6667 ) ) ;
#6506=VECTOR ( 'NONE', #60355, 1000.000000000000000 ) ;
#6511=ORIENTED_EDGE ( 'NONE', *, *, #52700, .F. ) ;
#6514=CARTESIAN_POINT ( 'NONE',  ( 8.449745872479532238, -2.260409384866206128, 7.500964401359662581 ) ) ;
#6519=CARTESIAN_POINT ( 'NONE',  ( 9.569799020577001158, -4.064052785562999759, 8.919253808370999792 ) ) ;
#6527=CARTESIAN_POINT ( 'NONE',  ( 10.35084866221912137, -5.758574906236493263, -7.748452900945333788 ) ) ;
#6530=CARTESIAN_POINT ( 'NONE',  ( 8.961955453702401542, -2.270851131865847528, 7.235821414696904874 ) ) ;
#6535=APPLICATION_CONTEXT ( 'automotive_design' ) ;
#6540=VECTOR ( 'NONE', #54111, 1000.000000000000114 ) ;
#6557=CARTESIAN_POINT ( 'NONE',  ( 10.69578225082999978, -5.505007625740000243, -7.759264430206000540 ) ) ;
#6559=LINE ( 'NONE', #12159, #28336 ) ;
#6564=CARTESIAN_POINT ( 'NONE',  ( 11.09999999999999964, -2.274006712557999688, -7.281956340829000673 ) ) ;
#6576=ORIENTED_EDGE ( 'NONE', *, *, #28951, .T. ) ;
#6593=CARTESIAN_POINT ( 'NONE',  ( 10.14750362918999826, -2.602959084636999876, 6.738575912023000214 ) ) ;
#6598=CARTESIAN_POINT ( 'NONE',  ( 10.31966935320999923, -4.764591648058999596, -5.997654637741999473 ) ) ;
#6599=CARTESIAN_POINT ( 'NONE',  ( 7.744183139975749697, -5.475625709055735868, 8.421281122564774790 ) ) ;
#6600=CARTESIAN_POINT ( 'NONE',  ( 9.843726350706999639, -4.115123626494000320, 9.466607949400000166 ) ) ;
#6617=ORIENTED_EDGE ( 'NONE', *, *, #744, .F. ) ;
#6627=CARTESIAN_POINT ( 'NONE',  ( 10.72129555961999792, -4.673507771948999689, -5.778404201896999659 ) ) ;
#6636=ORIENTED_EDGE ( 'NONE', *, *, #14550, .T. ) ;
#6645=ORIENTED_EDGE ( 'NONE', *, *, #26350, .F. ) ;
#6648=DIRECTION ( 'NONE',  ( 0.8660254037831510709, 1.247809965406074354E-13, -0.5000000000022299940 ) ) ;
#6655=LINE ( 'NONE', #22733, #67368 ) ;
#6661=DIRECTION ( 'NONE',  ( 0.000000000000000000, 0.000000000000000000, 1.000000000000000000 ) ) ;
#6667=ORIENTED_EDGE ( 'NONE', *, *, #61977, .F. ) ;
#6672=CARTESIAN_POINT ( 'NONE',  ( 9.174642513462206495, -2.649442673322992103, 7.499981897072125925 ) ) ;
#6677=ORIENTED_EDGE ( 'NONE', *, *, #61176, .T. ) ;
#6679=CARTESIAN_POINT ( 'NONE',  ( 11.09999999999999964, -5.350000000000000533, 7.500000000000000000 ) ) ;
#6689=CARTESIAN_POINT ( 'NONE',  ( 10.58470685321000104, -2.966812129551000154, -8.831977776575000050 ) ) ;
#6709=CARTESIAN_POINT ( 'NONE',  ( 10.04002603384999937, -2.348908096685999869, -7.136751747961000092 ) ) ;
#6713=ADVANCED_FACE ( 'NONE', ( #5671 ), #27405, .F. ) ;
#6718=CARTESIAN_POINT ( 'NONE',  ( 10.54675686666999823, -5.053011711995999633, 4.944839641817000420 ) ) ;
#6722=CARTESIAN_POINT ( 'NONE',  ( 10.68361719090999884, -2.603550124652000086, 7.762065570229999878 ) ) ;
#6733=CARTESIAN_POINT ( 'NONE',  ( 10.23643195768000069, -5.517145045299000294, -6.754127937316000363 ) ) ;
#6737=CARTESIAN_POINT ( 'NONE',  ( 10.90000000000000036, -2.899999999999999911, 6.414037451299000381 ) ) ;
#6749=CARTESIAN_POINT ( 'NONE',  ( 8.228217774218997249, -3.441349337319001389, 6.127431371819001882 ) ) ;
#6752=CARTESIAN_POINT ( 'NONE',  ( 9.820206362952999868, -3.883324525498000224, 6.055606607331999847 ) ) ;
#6753=CARTESIAN_POINT ( 'NONE',  ( 10.90227331380999942, -2.900050252960999941, -5.143660774000999858 ) ) ;
#6767=FACE_OUTER_BOUND ( 'NONE', #68845, .T. ) ;
#6791=CARTESIAN_POINT ( 'NONE',  ( 10.96666666666865453, -4.766458981284529273, 8.714450223968791320 ) ) ;
#6793=CARTESIAN_POINT ( 'NONE',  ( 9.509907746701999898, -5.077451867123000007, 8.469011304701000498 ) ) ;
#6798=CARTESIAN_POINT ( 'NONE',  ( 10.61094409420999973, -5.100000000000000533, -6.571291218949999902 ) ) ;
#6807=VECTOR ( 'NONE', #42522, 1000.000000000000000 ) ;
#6829=CARTESIAN_POINT ( 'NONE',  ( 10.97865453029000093, -5.273142482194999481, 7.958032781726000593 ) ) ;
#6831=CARTESIAN_POINT ( 'NONE',  ( 8.026331853209001110, -5.601799093797000140, 7.176147756900999930 ) ) ;
#6834=CARTESIAN_POINT ( 'NONE',  ( 11.02143415462000142, -6.120828910132000367, 5.114867263064000191 ) ) ;
#6835=CARTESIAN_POINT ( 'NONE',  ( 9.105958040553998600, -5.104280076368001851, -6.665288755903000073 ) ) ;
#6839=CARTESIAN_POINT ( 'NONE',  ( 11.03776785110999903, -5.237767851104999650, 6.571291218949999902 ) ) ;
#6840=CARTESIAN_POINT ( 'NONE',  ( 10.81905590578999998, -2.899999999999999911, -6.571291218949999902 ) ) ;
#6846=CARTESIAN_POINT ( 'NONE',  ( 10.18576633586640767, -4.069734382926335492, -8.865705745738447163 ) ) ;
#6852=CARTESIAN_POINT ( 'NONE',  ( 9.565773468336619345, -5.100000000000000533, 6.304440313901286785 ) ) ;
#6857=EDGE_CURVE ( 'NONE', #23757, #51247, #41293, .T. ) ;
#6867=CARTESIAN_POINT ( 'NONE',  ( 9.498146308785210934, -4.816854805705224507, 8.576504408122966439 ) ) ;
#6871=ORIENTED_EDGE ( 'NONE', *, *, #56040, .F. ) ;
#6872=FACE_OUTER_BOUND ( 'NONE', #9623, .T. ) ;
#6884=CARTESIAN_POINT ( 'NONE',  ( 10.62947109217999930, -5.100000000000000533, 6.152188490330000370 ) ) ;
#6896=DIRECTION ( 'NONE',  ( 0.000000000000000000, 1.000000000000000000, 0.000000000000000000 ) ) ;
#6900=CARTESIAN_POINT ( 'NONE',  ( 9.780291077142999612, -3.021588645102999848, -8.450043670922001482 ) ) ;
#6910=CARTESIAN_POINT ( 'NONE',  ( 9.140753410162000492, -5.100000000000000533, 6.175944241622000064 ) ) ;
#6916=EDGE_CURVE ( 'NONE', #43113, #45838, #52813, .T. ) ;
#6921=ORIENTED_EDGE ( 'NONE', *, *, #15801, .F. ) ;
#6922=CARTESIAN_POINT ( 'NONE',  ( 8.528441940379998698, -2.472358291268000219, 6.234202627038999189 ) ) ;
#6923=CARTESIAN_POINT ( 'NONE',  ( 9.795737326637999232, -4.289037785427000316, -5.816478295321999781 ) ) ;
#6932=CARTESIAN_POINT ( 'NONE',  ( 6.799999999999999822, -9.295462635088998837, -5.399710584805999858 ) ) ;
#6937=CARTESIAN_POINT ( 'NONE',  ( 10.30047649312000146, -4.027768368024999823, 9.431342508940000258 ) ) ;
#6938=CARTESIAN_POINT ( 'NONE',  ( 8.256683059623998844, -2.876278577719999952, 6.568889245344999850 ) ) ;
#6945=CARTESIAN_POINT ( 'NONE',  ( 10.54684435321000002, -3.691674321452999674, -9.157280075569998345 ) ) ;
#6946=CARTESIAN_POINT ( 'NONE',  ( 8.079085852406842960, -4.100770249492976305, 5.760890686963834106 ) ) ;
#6947=CARTESIAN_POINT ( 'NONE',  ( 9.504901164121001500, -3.934733502342999678, 5.704835336325999151 ) ) ;
#6957=EDGE_LOOP ( 'NONE', ( #20963, #52770, #12328, #63020, #61505, #20280 ) ) ;
#6971=ADVANCED_FACE ( 'NONE', ( #38802 ), #1736, .T. ) ;
#6974=CARTESIAN_POINT ( 'NONE',  ( 10.07763305961999833, -2.169024213715999849, -7.244986319234999250 ) ) ;
#6979=B_SPLINE_CURVE_WITH_KNOTS ( 'NONE', 3,
 ( #55783, #27485, #17692, #7195 ),
 .UNSPECIFIED., .F., .F.,
 ( 4, 4 ),
 ( 0.000000000000000000, 0.1324350869623206473 ),
 .UNSPECIFIED. ) ;
#6985=CARTESIAN_POINT ( 'NONE',  ( -15.86200481174999943, -2.399999999999999911, 6.571291218949999902 ) ) ;
#6994=ORIENTED_EDGE ( 'NONE', *, *, #13551, .T. ) ;
#7008=ORIENTED_EDGE ( 'NONE', *, *, #42532, .F. ) ;
#7042=CARTESIAN_POINT ( 'NONE',  ( 10.20608185320999972, -2.622355301673999772, -6.528538675937999969 ) ) ;
#7056=CARTESIAN_POINT ( 'NONE',  ( 9.709204462304001026, -2.899999999999999911, 6.662590550603789019 ) ) ;
#7061=CARTESIAN_POINT ( 'NONE',  ( 11.02205565301999890, -2.309485172892000282, -7.515673712097999726 ) ) ;
#7067=CARTESIAN_POINT ( 'NONE',  ( 10.41599088719999955, -4.897727109276999613, 5.040303808578999956 ) ) ;
#7069=CARTESIAN_POINT ( 'NONE',  ( 10.27427173964635898, -3.287502775498966301, 4.944156915057607016 ) ) ;
#7072=CARTESIAN_POINT ( 'NONE',  ( 10.14750362918999826, -2.602959084636999876, 6.738575912023000214 ) ) ;
#7083=CARTESIAN_POINT ( 'NONE',  ( 10.68054891417000007, -2.768175152062000155, -6.114413274984999980 ) ) ;
#7088=DIRECTION ( 'NONE',  ( -0.000000000000000000, 1.000000000000000000, 0.000000000000000000 ) ) ;
#7102=CARTESIAN_POINT ( 'NONE',  ( 7.426677373658002956, -3.232655724474999381, 6.473459691208998557 ) ) ;
#7106=CARTESIAN_POINT ( 'NONE',  ( 10.96580795178999956, -4.930647899304999804, 6.170539049947000088 ) ) ;
#7107=CARTESIAN_POINT ( 'NONE',  ( 9.791887411239740047, -4.711645841719509953, 9.126404666217009520 ) ) ;
#7110=ORIENTED_EDGE ( 'NONE', *, *, #6916, .T. ) ;
#7115=CARTESIAN_POINT ( 'NONE',  ( 10.99798614923244600, -2.813325336768271345, -5.071883290842238878 ) ) ;
#7117=CARTESIAN_POINT ( 'NONE',  ( 7.000000000000000000, 0.5292307692307999245, -2.083846153846000249 ) ) ;
#7121=DIRECTION ( 'NONE',  ( 0.000000000000000000, 0.8648648648648720183, -0.5020047465136825426 ) ) ;
#7134=ORIENTED_EDGE ( 'NONE', *, *, #66607, .T. ) ;
#7136=CARTESIAN_POINT ( 'NONE',  ( 8.481683059623998489, -2.472358291268000219, 6.234202627038999189 ) ) ;
#7141=DIRECTION ( 'NONE',  ( -1.000000000000000000, 0.000000000000000000, 0.000000000000000000 ) ) ;
#7145=CARTESIAN_POINT ( 'NONE',  ( 11.02786767503999954, -5.596230239120999705, 7.209501483790000442 ) ) ;
#7159=CARTESIAN_POINT ( 'NONE',  ( 9.377480346882569151, -2.931296748430716193, 8.873990698568421820 ) ) ;
#7167=CARTESIAN_POINT ( 'NONE',  ( 9.504901164121001500, -3.934733502342999678, 5.704835336325999151 ) ) ;
#7179=EDGE_CURVE ( 'NONE', #55729, #17154, #13409, .T. ) ;
#7182=CARTESIAN_POINT ( 'NONE',  ( 8.539831853209999935, -5.633481712366999794, 7.451234046297000368 ) ) ;
#7185=CARTESIAN_POINT ( 'NONE',  ( 11.12373728587000166, -5.759484258661999867, 5.183808156345000029 ) ) ;
#7191=B_SPLINE_SURFACE_WITH_KNOTS ( 'NONE', 3, 3, ( 
 ( #30583, #40722, #34808, #67284 ),
 ( #29222, #56815, #19057, #46668 ),
 ( #51895, #3993, #2976, #50534 ),
 ( #8230, #51554, #2636, #23963 ),
 ( #66946, #24652, #57479, #52936 ) ),
 .UNSPECIFIED., .F., .F., .F.,
 ( 4, 1, 4 ),
 ( 4, 4 ),
 ( 0.9547086424368000923, 1.000000000000000000, 1.007144313228999888 ),
 ( -0.1721939420595999803, 1.172193941872999856 ),
 .UNSPECIFIED. ) ;
#7195=CARTESIAN_POINT ( 'NONE',  ( 11.08380555355832620, -3.999999927290649460, -9.033895164528411570 ) ) ;
#7201=CARTESIAN_POINT ( 'NONE',  ( 8.500365452454994752, -5.097361224984004124, 6.605627025648004746 ) ) ;
#7214=CARTESIAN_POINT ( 'NONE',  ( 8.577663641219146484, -4.062279398746261094, 5.761468528428593139 ) ) ;
#7220=CARTESIAN_POINT ( 'NONE',  ( 9.502127015675981170, -4.762560867020375177, 8.617745476188831688 ) ) ;
#7229=CARTESIAN_POINT ( 'NONE',  ( 8.613182395984926742, -4.653584300239352878, 5.903187239484563698 ) ) ;
#7238=LINE ( 'NONE', #44997, #35494 ) ;
#7250=CARTESIAN_POINT ( 'NONE',  ( 10.30297040315999979, -4.081263557776000361, -9.025012210052000938 ) ) ;
#7255=VERTEX_POINT ( 'NONE', #50742 ) ;
#7271=CARTESIAN_POINT ( 'NONE',  ( 8.721004440379999778, -5.983034890242000081, 7.440798487724999966 ) ) ;
#7272=CARTESIAN_POINT ( 'NONE',  ( 10.10891502095999961, -5.332339947063000629, -7.851654145788001138 ) ) ;
#7274=ADVANCED_FACE ( 'NONE', ( #40933 ), #68175, .T. ) ;
#7288=CARTESIAN_POINT ( 'NONE',  ( 9.260912867475999732, -4.901383038209000453, 9.090314591495999963 ) ) ;
#7289=CARTESIAN_POINT ( 'NONE',  ( 9.069724726289001282, -4.108965473266000146, 8.851626696081998702 ) ) ;
#7293=CARTESIAN_POINT ( 'NONE',  ( 10.23580444037999904, -3.621838308198000345, -8.806219190581000333 ) ) ;
#7294=CARTESIAN_POINT ( 'NONE',  ( 7.955723615552813044, -2.265131536788511646, 7.358139940862454154 ) ) ;
#7295=CARTESIAN_POINT ( 'NONE',  ( 9.124702828701000357, -4.778665285493000070, 8.799745834808000211 ) ) ;
#7302=CARTESIAN_POINT ( 'NONE',  ( 9.107059081473819262, -5.098368162008560134, -6.579893398394093929 ) ) ;
#7312=CARTESIAN_POINT ( 'NONE',  ( 9.433105646793000787, -4.954907757874000396, 8.825780921426000347 ) ) ;
#7318=CARTESIAN_POINT ( 'NONE',  ( 10.53198305961999992, -2.323723769066000422, -8.279488812962998878 ) ) ;
#7335=CARTESIAN_POINT ( 'NONE',  ( 10.98768503802999952, -8.067884818888000353, -6.818830313157000056 ) ) ;
#7342=DIRECTION ( 'NONE',  ( 0.000000000000000000, 1.000000000000000000, 0.000000000000000000 ) ) ;
#7399=DIRECTION ( 'NONE',  ( 1.000000000000000000, 0.000000000000000000, 0.000000000000000000 ) ) ;
#7400=EDGE_CURVE ( 'NONE', #42097, #51258, #49300, .T. ) ;
#7404=CARTESIAN_POINT ( 'NONE',  ( 10.19715077290999972, -4.982624057277000418, -6.124316828241999744 ) ) ;
#7411=CARTESIAN_POINT ( 'NONE',  ( 11.00643352828999966, -5.061761008800999662, 5.194533778134999835 ) ) ;
#7415=CARTESIAN_POINT ( 'NONE',  ( 10.78089914631999946, -5.735295708369000600, 7.801561210335000496 ) ) ;
#7426=EDGE_CURVE ( 'NONE', #21138, #438, #37067, .T. ) ;
#7432=CARTESIAN_POINT ( 'NONE',  ( 9.524152735436000938, -4.911674715448000050, -6.466751564808000730 ) ) ;
#7438=CARTESIAN_POINT ( 'NONE',  ( 11.04989271531000128, -2.849679502984999946, 5.124329486915000231 ) ) ;
#7439=CARTESIAN_POINT ( 'NONE',  ( 7.491953176340000908, -3.528027000165000704, 6.607934030033999484 ) ) ;
#7440=EDGE_LOOP ( 'NONE', ( #9883, #36078, #55500, #900, #34301, #45290, #29182, #20319, #31149 ) ) ;
#7444=CARTESIAN_POINT ( 'NONE',  ( 9.137549407199999862, -2.995696424181999884, 8.544763501938000161 ) ) ;
#7447=CARTESIAN_POINT ( 'NONE',  ( 9.662553763536999796, -4.094830574823999925, 9.119950378356000087 ) ) ;
#7459=CARTESIAN_POINT ( 'NONE',  ( 7.766851002543999627, -2.832432432432000269, 6.822293592207000934 ) ) ;
#7460=CARTESIAN_POINT ( 'NONE',  ( 9.262725409949998934, -4.818302824158000597, -8.808202952968999355 ) ) ;
#7470=EDGE_LOOP ( 'NONE', ( #31768, #67954, #52884, #4898 ) ) ;
#7478=CARTESIAN_POINT ( 'NONE',  ( 11.10000000000000142, -2.933222718292388898, -8.703884637941042612 ) ) ;
#7483=CARTESIAN_POINT ( 'NONE',  ( 10.95833333333531634, -4.952949899268980438, 8.562434272073259578 ) ) ;
#7500=EDGE_LOOP ( 'NONE', ( #61739, #42826, #29328, #25414, #6143 ) ) ;
#7501=CARTESIAN_POINT ( 'NONE',  ( 8.235184868407717573, -4.918172741149095195, 6.252519622020343171 ) ) ;
#7507=CARTESIAN_POINT ( 'NONE',  ( 9.471368011205999693, -2.030678448189000118, 7.549764202121000523 ) ) ;
#7510=ORIENTED_EDGE ( 'NONE', *, *, #9823, .F. ) ;
#7516=CARTESIAN_POINT ( 'NONE',  ( 9.164312934263135091, -5.579507257161629319, 6.755493088102384469 ) ) ;
#7517=CARTESIAN_POINT ( 'NONE',  ( 8.860769353209001054, -2.935738482289000029, 6.259841087764999479 ) ) ;
#7520=CARTESIAN_POINT ( 'NONE',  ( 11.07074853682000004, -6.638037936241000025, 5.577182366698000493 ) ) ;
#7522=ORIENTED_EDGE ( 'NONE', *, *, #30336, .T. ) ;
#7524=EDGE_CURVE ( 'NONE', #38985, #48366, #12527, .T. ) ;
#7525=CARTESIAN_POINT ( 'NONE',  ( 11.08558905797000094, -2.762729330199000355, -5.050875529400999930 ) ) ;
#7528=ADVANCED_FACE ( 'NONE', ( #50573 ), #55824, .F. ) ;
#7531=CARTESIAN_POINT ( 'NONE',  ( 9.316120559621998254, -3.677416446733000388, 9.250734868033999803 ) ) ;
#7553=CARTESIAN_POINT ( 'NONE',  ( 8.579433303903055474, -4.102305646687347540, 5.763126848776402689 ) ) ;
#7554=CARTESIAN_POINT ( 'NONE',  ( 9.073148997461000675, -5.167567567567999731, -6.822293592207000934 ) ) ;
#7559=ORIENTED_EDGE ( 'NONE', *, *, #23517, .F. ) ;
#7560=CARTESIAN_POINT ( 'NONE',  ( 9.488131779409266997, -4.942974209866618729, 8.465868502208129698 ) ) ;
#7563=B_SPLINE_CURVE_WITH_KNOTS ( 'NONE', 3,
 ( #51998, #4102, #25437, #61475 ),
 .UNSPECIFIED., .F., .F.,
 ( 4, 4 ),
 ( 0.000000000000000000, 1.000000000000000000 ),
 .UNSPECIFIED. ) ;
#7570=DIRECTION ( 'NONE',  ( -1.000000000000000000, 0.000000000000000000, -9.837659932951999203E-14 ) ) ;
#7572=CARTESIAN_POINT ( 'NONE',  ( 8.620740978634000129, -4.599999999999999645, 5.898823289756999877 ) ) ;
#7575=ADVANCED_FACE ( 'NONE', ( #35192 ), #27605, .F. ) ;
#7596=CARTESIAN_POINT ( 'NONE',  ( 9.831596185961002377, -3.539228349258999984, -8.956015611440999891 ) ) ;
#7601=VERTEX_POINT ( 'NONE', #43691 ) ;
#7606=CARTESIAN_POINT ( 'NONE',  ( 10.76087777166854131, -3.646736399437864762, -8.814656132371565533 ) ) ;
#7607=DIRECTION ( 'NONE',  ( -1.070254833719000005E-12, -1.000000000000000000, 8.737453881089000797E-12 ) ) ;
#7608=FACE_OUTER_BOUND ( 'NONE', #43895, .T. ) ;
#7609=AXIS2_PLACEMENT_3D ( 'NONE', #48742, #1193, #22852 ) ;
#7615=AXIS2_PLACEMENT_3D ( 'NONE', #63685, #54230, #21048 ) ;
#7620=CARTESIAN_POINT ( 'NONE',  ( 8.271691940379001906, -5.629389383493999865, 8.631822608164000599 ) ) ;
#7633=CARTESIAN_POINT ( 'NONE',  ( 10.39106278671000005, -4.025320977579999848, 9.261121875182000807 ) ) ;
#7639=CARTESIAN_POINT ( 'NONE',  ( 7.965071509961973995, -2.295647626639265138, 7.153698218240838180 ) ) ;
#7640=CARTESIAN_POINT ( 'NONE',  ( 10.74609562913000005, -4.263104965433000437, 9.276976808608999647 ) ) ;
#7649=CARTESIAN_POINT ( 'NONE',  ( 9.355720302797999821, -5.362859773739999447, -6.470306978669999154 ) ) ;
#7662=EDGE_LOOP ( 'NONE', ( #30546, #11248, #56079, #66465, #41623, #6636, #8140 ) ) ;
#7663=CARTESIAN_POINT ( 'NONE',  ( 8.829019353210000531, -5.290204991635000020, 8.768102264518001121 ) ) ;
#7668=CARTESIAN_POINT ( 'NONE',  ( 10.26694555961999988, -5.500014128486999887, -6.419508248405999318 ) ) ;
#7679=EDGE_CURVE ( 'NONE', #57810, #22584, #47739, .T. ) ;
#7686=ADVANCED_FACE ( 'NONE', ( #35867 ), #26064, .F. ) ;
#7709=CARTESIAN_POINT ( 'NONE',  ( 9.010191940380000375, -5.040796345420999636, 8.522966281393001609 ) ) ;
#7729=EDGE_LOOP ( 'NONE', ( #14112, #23245, #37244, #33535 ) ) ;
#7731=CARTESIAN_POINT ( 'NONE',  ( 10.72614816446315267, -5.074971087576590989, 5.079084875746824324 ) ) ;
#7742=ORIENTED_EDGE ( 'NONE', *, *, #19397, .T. ) ;
#7758=CARTESIAN_POINT ( 'NONE',  ( 10.36409413284604497, -3.282837288405540122, -4.954046114881531793 ) ) ;
#7759=ORIENTED_EDGE ( 'NONE', *, *, #1278, .T. ) ;
#7762=DIRECTION ( 'NONE',  ( 0.000000000000000000, -1.000000000000000000, 0.000000000000000000 ) ) ;
#7763=CARTESIAN_POINT ( 'NONE',  ( 10.26028798067999936, -4.571539164417999679, 4.531786735957999745 ) ) ;
#7766=DIRECTION ( 'NONE',  ( 1.000000000000000000, 0.000000000000000000, 0.000000000000000000 ) ) ;
#7768=CARTESIAN_POINT ( 'NONE',  ( 10.42595817177000050, -5.042180160032999403, 8.702227297563000619 ) ) ;
#7775=CARTESIAN_POINT ( 'NONE',  ( 10.54885391751724022, -4.021057898797131713, 8.964616684112781897 ) ) ;
#7785=CARTESIAN_POINT ( 'NONE',  ( 9.656157842586999607, -4.949038487346999915, -8.498994087616001281 ) ) ;
#7791=CARTESIAN_POINT ( 'NONE',  ( 10.85025860864000080, -2.931433838835999950, 5.153723152236999283 ) ) ;
#7794=CARTESIAN_POINT ( 'NONE',  ( 10.27427156480999848, -3.399999787207999447, 4.944156960757000618 ) ) ;
#7795=CARTESIAN_POINT ( 'NONE',  ( 9.290195424034999760, -2.377814350880000038, 7.540992175424999999 ) ) ;
#7800=CARTESIAN_POINT ( 'NONE',  ( 9.228135700785001561, -2.875364528161000077, 8.669943154892999715 ) ) ;
#7808=CARTESIAN_POINT ( 'NONE',  ( 8.675212715831998267, -2.915713811628002361, -6.499218380552004071 ) ) ;
#7812=CARTESIAN_POINT ( 'NONE',  ( 9.397313405920000307, -4.010297355695000121, -9.208122400763999238 ) ) ;
#7828=B_SPLINE_CURVE_WITH_KNOTS ( 'NONE', 3,
 ( #24029, #18105, #17763, #28244 ),
 .UNSPECIFIED., .F., .F.,
 ( 4, 4 ),
 ( 0.000000000000000000, 1.000000000000000000 ),
 .UNSPECIFIED. ) ;
#7836=CARTESIAN_POINT ( 'NONE',  ( 11.10000000000000320, -2.858656910680171581, -8.645179761462580714 ) ) ;
#7838=CARTESIAN_POINT ( 'NONE',  ( 9.312954706844832842, -5.052526710679146049, -6.210582334949435790 ) ) ;
#7846=CARTESIAN_POINT ( 'NONE',  ( 10.98768491210000064, -8.067891622241001315, 6.818837029638999958 ) ) ;
#7854=B_SPLINE_CURVE_WITH_KNOTS ( 'NONE', 3,
 ( #2407, #23730, #45068, #66721 ),
 .UNSPECIFIED., .F., .F.,
 ( 4, 4 ),
 ( 0.000000000000000000, 1.000000000000000000 ),
 .UNSPECIFIED. ) ;
#7856=CARTESIAN_POINT ( 'NONE',  ( 9.409633934533484734, -2.474451488929216403, 8.335641178190561718 ) ) ;
#7863=CARTESIAN_POINT ( 'NONE',  ( 11.08992739829000129, -5.210546653347999602, 8.327600405525998895 ) ) ;
#7868=VERTEX_POINT ( 'NONE', #12048 ) ;
#7872=CARTESIAN_POINT ( 'NONE',  ( 9.263741181053154250, -5.204002092419764303, 8.765996337996943666 ) ) ;
#7873=CARTESIAN_POINT ( 'NONE',  ( 8.668206853210000062, -3.979464503892999439, 9.134080454305001595 ) ) ;
#7889=CARTESIAN_POINT ( 'NONE',  ( 10.21685100254000034, -2.832432432432000269, 6.822293592207000934 ) ) ;
#7892=CARTESIAN_POINT ( 'NONE',  ( 7.729221580034996819, -5.085115902530001897, 6.553339126910996626 ) ) ;
#7902=EDGE_LOOP ( 'NONE', ( #57443, #56918, #12612, #5830, #27021 ) ) ;
#7905=B_SPLINE_CURVE_WITH_KNOTS ( 'NONE', 3,
 ( #54487, #59728, #64273, #26895 ),
 .UNSPECIFIED., .F., .F.,
 ( 4, 4 ),
 ( 0.8745818872751025541, 1.000000000000000000 ),
 .UNSPECIFIED. ) ;
#7906=CARTESIAN_POINT ( 'NONE',  ( 9.567166575710958298, -2.899999999999999911, -6.351075879690426973 ) ) ;
#7910=ORIENTED_EDGE ( 'NONE', *, *, #19837, .T. ) ;
#7913=CARTESIAN_POINT ( 'NONE',  ( 9.490614771213035539, -4.913405583856841119, 8.493963967124175340 ) ) ;
#7917=VERTEX_POINT ( 'NONE', #64137 ) ;
#7918=CARTESIAN_POINT ( 'NONE',  ( 9.131856313922000368, -8.648524463724998057, 6.068074759017999753 ) ) ;
#7933=CARTESIAN_POINT ( 'NONE',  ( 10.98845665678465799, -2.811543343220049174, -6.624101343727395452 ) ) ;
#7945=CARTESIAN_POINT ( 'NONE',  ( 10.36629943602999937, -5.852732332139999549, -7.568014220767000033 ) ) ;
#7947=CARTESIAN_POINT ( 'NONE',  ( 9.032937857236275292, -5.014695576459849313, 8.393597907926556800 ) ) ;
#7954=DIRECTION ( 'NONE',  ( 1.000000000000000000, 0.000000000000000000, 0.000000000000000000 ) ) ;
#7965=AXIS2_PLACEMENT_3D ( 'NONE', #60903, #30137, #39931 ) ;
#7969=CARTESIAN_POINT ( 'NONE',  ( 8.977754440379998258, -2.019079883662000086, 7.390983468784999566 ) ) ;
#7973=CARTESIAN_POINT ( 'NONE',  ( 11.09998944727697356, -2.658360006774485917, 6.717872455900587347 ) ) ;
#7985=CARTESIAN_POINT ( 'NONE',  ( 10.94797187187000098, -2.864324950622999744, 8.846246404612999825 ) ) ;
#7990=CARTESIAN_POINT ( 'NONE',  ( 10.27366694038000006, -3.065543393453000309, -8.487918777453998587 ) ) ;
#7991=CARTESIAN_POINT ( 'NONE',  ( 7.932978819056404340, -2.299600510671482301, 7.867486896083077497 ) ) ;
#7992=CARTESIAN_POINT ( 'NONE',  ( 9.075489683949001574, -4.020837068201999820, 8.948702918089999514 ) ) ;
#8011=CARTESIAN_POINT ( 'NONE',  ( 8.213543146793000460, -3.608524635952000459, 5.913372239166000632 ) ) ;
#8018=DIRECTION ( 'NONE',  ( -0.7071067811865329178, -0.1740570520339079497, 0.6853496499140319109 ) ) ;
#8032=VECTOR ( 'NONE', #525, 1000.000000000000000 ) ;
#8052=CARTESIAN_POINT ( 'NONE',  ( 10.81771127433663970, -4.157152761341111891, 9.232783412159369263 ) ) ;
#8053=CARTESIAN_POINT ( 'NONE',  ( 7.533879440377999614, -4.623636604834999275, 8.651469651195000665 ) ) ;
#8063=CYLINDRICAL_SURFACE ( 'NONE', #55886, 1.350000000000000089 ) ;
#8068=CARTESIAN_POINT ( 'NONE',  ( 7.731793146792000471, -4.580607464247000493, 9.213361409141999303 ) ) ;
#8071=EDGE_CURVE ( 'NONE', #61687, #42399, #27507, .T. ) ;
#8073=CARTESIAN_POINT ( 'NONE',  ( 7.433354470783482881, -2.295550242067167179, 7.846515896910211119 ) ) ;
#8074=VECTOR ( 'NONE', #61270, 1000.000000000000000 ) ;
#8084=CARTESIAN_POINT ( 'NONE',  ( 5.700000000000000178, -1.300000000000000044, -9.662944685757000940 ) ) ;
#8085=CARTESIAN_POINT ( 'NONE',  ( 7.000000000000000000, 0.8000000000000000444, 3.149999999999999911 ) ) ;
#8087=LINE ( 'NONE', #44473, #12031 ) ;
#8090=VERTEX_POINT ( 'NONE', #66828 ) ;
#8101=CARTESIAN_POINT ( 'NONE',  ( 9.681180837610000367, -2.612237299844000216, 7.804680206899999639 ) ) ;
#8115=CARTESIAN_POINT ( 'NONE',  ( 10.20319453770999907, -3.421758889707999796, 6.017729046583999875 ) ) ;
#8125=CARTESIAN_POINT ( 'NONE',  ( 8.970944094206998898, -5.100000000000000533, 6.571291218949999902 ) ) ;
#8128=CARTESIAN_POINT ( 'NONE',  ( 10.06493315628555862, -5.349942305088194239, -7.500003965376651038 ) ) ;
#8130=FACE_OUTER_BOUND ( 'NONE', #6957, .T. ) ;
#8140=ORIENTED_EDGE ( 'NONE', *, *, #30948, .T. ) ;
#8142=CARTESIAN_POINT ( 'NONE',  ( 10.68403590588000007, -5.436611040123999317, 8.578433628717998971 ) ) ;
#8145=CARTESIAN_POINT ( 'NONE',  ( 9.601186317138909132, -5.349829778710892825, -7.263235859471102174 ) ) ;
#8151=CARTESIAN_POINT ( 'NONE',  ( 10.73543045066558399, -5.073272730021160193, -5.075194819112775590 ) ) ;
#8153=ADVANCED_FACE ( 'NONE', ( #67163, #67850 ), #24870, .F. ) ;
#8155=CARTESIAN_POINT ( 'NONE',  ( 10.87180915648999857, -2.933919166010999557, 5.127994723445000069 ) ) ;
#8159=CARTESIAN_POINT ( 'NONE',  ( 9.177304894000000601, -4.588307032459999490, -5.987050435448999508 ) ) ;
#8160=CARTESIAN_POINT ( 'NONE',  ( 5.700000000378000031, -0.2999999996220999443, 3.150000004979999879 ) ) ;
#8162=LINE ( 'NONE', #29509, #15448 ) ;
#8180=DIRECTION ( 'NONE',  ( 0.000000000000000000, 0.000000000000000000, -1.000000000000000000 ) ) ;
#8185=VERTEX_POINT ( 'NONE', #25900 ) ;
#8196=CARTESIAN_POINT ( 'NONE',  ( 9.381146409496318839, -2.870643679914145707, 8.823445380589753029 ) ) ;
#8205=CARTESIAN_POINT ( 'NONE',  ( 11.05639424537999993, -5.030223832177999732, 6.028291574375000295 ) ) ;
#8213=CARTESIAN_POINT ( 'NONE',  ( 9.299999999999998934, -4.537600397704999899, 9.154563893594000135 ) ) ;
#8219=CARTESIAN_POINT ( 'NONE',  ( 10.96504121510999852, -5.560326135739999565, 4.905747935756999745 ) ) ;
#8221=CARTESIAN_POINT ( 'NONE',  ( 8.429610941929999157, -5.086930576191002196, -6.619396742377001708 ) ) ;
#8225=CARTESIAN_POINT ( 'NONE',  ( 11.03789961707000167, -2.850875858055000212, -5.120756380231999749 ) ) ;
#8230=CARTESIAN_POINT ( 'NONE',  ( 11.13477878846000024, -5.334327202385000355, 5.176824473787999814 ) ) ;
#8240=CARTESIAN_POINT ( 'NONE',  ( 7.790489386131184801, -2.917550760077413763, 6.652506093142642740 ) ) ;
#8251=CONICAL_SURFACE ( 'NONE', #37288, 0.3796172482170003804, 0.7853981633972997312 ) ;
#8252=CARTESIAN_POINT ( 'NONE',  ( 9.444317341922999987, -2.927260449021000355, 8.897015448164999896 ) ) ;
#8255=CARTESIAN_POINT ( 'NONE',  ( 7.892605646791999163, -5.480312458445999901, 8.192326492433998908 ) ) ;
#8257=VERTEX_POINT ( 'NONE', #61585 ) ;
#8258=CARTESIAN_POINT ( 'NONE',  ( 6.871402371741999637, -9.249258202502000259, 5.114981648749999721 ) ) ;
#8263=VERTEX_POINT ( 'NONE', #46545 ) ;
#8264=CARTESIAN_POINT ( 'NONE',  ( 8.709204462306566086, -2.899999999999999911, 6.662590550605525408 ) ) ;
#8279=EDGE_CURVE ( 'NONE', #65964, #27255, #53391, .T. ) ;
#8287=B_SPLINE_CURVE_WITH_KNOTS ( 'NONE', 3,
 ( #62197, #24459, #14318, #40529, #35643, #56273, #19205, #34958, #45782, #61854, #13973, #35300, #51703, #56955, #9057, #3800, #42263, #31769 ),
 .UNSPECIFIED., .F., .F.,
 ( 4, 2, 2, 2, 2, 2, 2, 2, 4 ),
 ( 0.1254120260046326096, 0.2190586444436944391, 0.3127052628827562963, 0.4063518813218180981, 0.4999984997608799553, 0.5936451181999418125, 0.6872917366390036698, 0.7809383550780655270, 0.8745849735171273842 ),
 .UNSPECIFIED. ) ;
#8291=CARTESIAN_POINT ( 'NONE',  ( 10.64126772939999910, -2.258710642251000156, -6.863482599505999815 ) ) ;
#8311=CARTESIAN_POINT ( 'NONE',  ( 8.437855646795000553, -2.606998386752999775, 6.345764833140000505 ) ) ;
#8328=CARTESIAN_POINT ( 'NONE',  ( 9.353731048338000065, -2.823575173856999410, 9.032043499493001448 ) ) ;
#8332=CARTESIAN_POINT ( 'NONE',  ( 10.57656694038000111, -5.344897889496000865, -7.298883676216999739 ) ) ;
#8333=CARTESIAN_POINT ( 'NONE',  ( 8.059281404067426990, -3.659214940308822328, 5.794006878043420627 ) ) ;
#8334=CARTESIAN_POINT ( 'NONE',  ( 10.03491210303999992, -5.615910465798999773, 7.351455544018000943 ) ) ;
#8338=CARTESIAN_POINT ( 'NONE',  ( 10.33482971575999976, -4.577985512478999652, -4.713492043800000530 ) ) ;
#8353=CARTESIAN_POINT ( 'NONE',  ( 7.956793146791999227, -4.524489047957000132, 9.047757046927999980 ) ) ;
#8359=CARTESIAN_POINT ( 'NONE',  ( 9.978906853208000527, -5.007779786185999171, -8.772596342864998675 ) ) ;
#8362=EDGE_CURVE ( 'NONE', #10252, #52199, #22548, .T. ) ;
#8366=DIRECTION ( 'NONE',  ( 0.000000000000000000, 0.000000000000000000, -1.000000000000000000 ) ) ;
#8372=ORIENTED_EDGE ( 'NONE', *, *, #30018, .F. ) ;
#8373=( NAMED_UNIT ( * ) SI_UNIT ( $, .STERADIAN. ) SOLID_ANGLE_UNIT ( ) );
#8374=CARTESIAN_POINT ( 'NONE',  ( 8.486008579191000933, -3.399999999999999911, 5.976611076844000614 ) ) ;
#8397=CARTESIAN_POINT ( 'NONE',  ( 7.635855646791999796, -2.466384407480000096, 6.935560677555000275 ) ) ;
#8407=CARTESIAN_POINT ( 'NONE',  ( 7.000000000000000000, -6.255435840762999966, 3.000000000000000000 ) ) ;
#8413=CARTESIAN_POINT ( 'NONE',  ( 8.464254440379999522, -2.029110377978999846, 7.726994002375999315 ) ) ;
#8418=CARTESIAN_POINT ( 'NONE',  ( 10.64200660897471451, -3.294104879791286855, 8.705431914969567586 ) ) ;
#8427=CARTESIAN_POINT ( 'NONE',  ( 10.39709479648126944, -5.286020290092475094, 7.026710849311109008 ) ) ;
#8444=CARTESIAN_POINT ( 'NONE',  ( 11.18483536755999808, -2.599651619047000040, 7.740676724427999922 ) ) ;
#8452=ORIENTED_EDGE ( 'NONE', *, *, #38258, .F. ) ;
#8454=CARTESIAN_POINT ( 'NONE',  ( 11.12483846379999974, -6.576344547557000375, -5.637698688823999937 ) ) ;
#8457=DIRECTION ( 'NONE',  ( 0.8480635683784220058, 0.000000000000000000, 0.5298945026977139872 ) ) ;
#8460=CARTESIAN_POINT ( 'NONE',  ( 10.55813551225999980, -2.466564559586000183, 6.633531786299999844 ) ) ;
#8466=CARTESIAN_POINT ( 'NONE',  ( 10.58079553768976666, -5.100000000000000533, -6.662590550605365536 ) ) ;
#8476=CARTESIAN_POINT ( 'NONE',  ( 9.128137413980999426, -5.235394649229000663, -8.110359502241001550 ) ) ;
#8486=CARTESIAN_POINT ( 'NONE',  ( 10.43579701286999928, -2.587605342384000195, 6.390039770907999461 ) ) ;
#8489=CARTESIAN_POINT ( 'NONE',  ( 10.62698276521000196, -3.142914536759000121, 8.668455626664998803 ) ) ;
#8492=CARTESIAN_POINT ( 'NONE',  ( 10.28912155192348621, -2.704284023348029642, -7.938084390888727526 ) ) ;
#8497=CARTESIAN_POINT ( 'NONE',  ( 8.517762173746001864, -3.198146119290998346, -6.396303957889001524 ) ) ;
#8501=CARTESIAN_POINT ( 'NONE',  ( 9.656157842586999607, -4.949038487346999915, -8.498994087616001281 ) ) ;
#8507=CARTESIAN_POINT ( 'NONE',  ( 8.933148997457999840, -5.167567567567999731, 6.822293592207000934 ) ) ;
#8511=ORIENTED_EDGE ( 'NONE', *, *, #63757, .F. ) ;
#8532=VERTEX_POINT ( 'NONE', #27028 ) ;
#8537=DIRECTION ( 'NONE',  ( 0.8660254037844289376, 0.000000000000000000, -0.5000000000000169864 ) ) ;
#8538=EDGE_LOOP ( 'NONE', ( #42409, #40463, #60314, #50560, #37986 ) ) ;
#8543=CARTESIAN_POINT ( 'NONE',  ( 11.09999999999999964, -4.000000000000000000, 7.500000000000000000 ) ) ;
#8545=AXIS2_PLACEMENT_3D ( 'NONE', #10055, #5838, #36283 ) ;
#8550=CARTESIAN_POINT ( 'NONE',  ( 10.90635170712999980, -3.089674976714000376, -6.534319251717000121 ) ) ;
#8562=CARTESIAN_POINT ( 'NONE',  ( 8.627495311384997478, -5.082984106378005684, -6.521832623478995394 ) ) ;
#8567=CARTESIAN_POINT ( 'NONE',  ( 9.751735624253999646, -3.361793157411000266, -5.915550373431999631 ) ) ;
#8570=FACE_OUTER_BOUND ( 'NONE', #44875, .T. ) ;
#8583=CARTESIAN_POINT ( 'NONE',  ( 10.47253786429000044, -2.899999999999999911, -6.571291218949999902 ) ) ;
#8593=CARTESIAN_POINT ( 'NONE',  ( 10.62792628238999981, -3.100579357212000176, 8.599905962393000536 ) ) ;
#8595=CARTESIAN_POINT ( 'NONE',  ( 8.379867906070000316, -2.923743482135000349, 6.439439799216000182 ) ) ;
#8596=CARTESIAN_POINT ( 'NONE',  ( 7.443293146792999693, -4.698358408974000255, 8.789434435623999065 ) ) ;
#8600=CARTESIAN_POINT ( 'NONE',  ( 11.04859286640970417, -4.978068212541741033, -8.665561624479661162 ) ) ;
#8607=ADVANCED_FACE ( 'NONE', ( #43456 ), #21245, .T. ) ;
#8616=CARTESIAN_POINT ( 'NONE',  ( 10.94592196013603136, -2.831029695124928747, -6.714227100558820993 ) ) ;
#8630=CARTESIAN_POINT ( 'NONE',  ( 10.68054891417000007, -2.768175152062000155, -6.114413274984999980 ) ) ;
#8637=CARTESIAN_POINT ( 'NONE',  ( 8.079129440378000737, -3.524751762020000179, 5.573845465339999805 ) ) ;
#8648=VECTOR ( 'NONE', #7607, 1000.000000000000000 ) ;
#8651=CARTESIAN_POINT ( 'NONE',  ( 8.154706853209001238, -4.255646685191999623, 9.114089645792999406 ) ) ;
#8656=CIRCLE ( 'NONE', #44410, 1.100000000000000089 ) ;
#8663=ADVANCED_FACE ( 'NONE', ( #57034 ), #9136, .F. ) ;
#8666=CARTESIAN_POINT ( 'NONE',  ( 9.416094968574279633, -5.100000000000000533, -6.473186325184255629 ) ) ;
#8668=CARTESIAN_POINT ( 'NONE',  ( 10.91307648679999964, -2.096298111716999646, 7.827187677719999570 ) ) ;
#8669=DIRECTION ( 'NONE',  ( 0.7071067811865474617, -0.7071067811865474617, 1.247903205617082848E-09 ) ) ;
#8670=ORIENTED_EDGE ( 'NONE', *, *, #46449, .T. ) ;
#8672=CARTESIAN_POINT ( 'NONE',  ( 10.91732944037999964, -3.256268970540999952, -6.361552695759000287 ) ) ;
#8673=CARTESIAN_POINT ( 'NONE',  ( 8.128394320951036534, -5.084803757088047327, 6.140078532315731863 ) ) ;
#8682=CARTESIAN_POINT ( 'NONE',  ( 9.221132306829000314, -4.645169647889000331, -5.840816811670999975 ) ) ;
#8683=CARTESIAN_POINT ( 'NONE',  ( 10.97413042750000045, -2.700916140920000430, -4.938597722914999544 ) ) ;
#8690=B_SPLINE_CURVE_WITH_KNOTS ( 'NONE', 3,
 ( #24923, #56049, #2230, #51157 ),
 .UNSPECIFIED., .F., .F.,
 ( 4, 4 ),
 ( 0.000000000000000000, 1.000000000000000000 ),
 .UNSPECIFIED. ) ;
#8692=ORIENTED_EDGE ( 'NONE', *, *, #22654, .T. ) ;
#8694=VECTOR ( 'NONE', #55980, 1000.000000000000000 ) ;
#8696=CARTESIAN_POINT ( 'NONE',  ( 9.368918146792999835, -5.618388245857000030, 7.727743016644000207 ) ) ;
#8702=CARTESIAN_POINT ( 'NONE',  ( 10.96333185321000059, -5.283547384770999500, -8.592770849731000027 ) ) ;
#8713=DIRECTION ( 'NONE',  ( -1.000000000000000000, 0.000000000000000000, 0.000000000000000000 ) ) ;
#8737=CARTESIAN_POINT ( 'NONE',  ( 10.92125287134683909, -2.370162430443217616, 8.128085326470900540 ) ) ;
#8738=CARTESIAN_POINT ( 'NONE',  ( 9.566483607044000692, -4.108965473266000146, 8.851626696081998702 ) ) ;
#8742=ORIENTED_EDGE ( 'NONE', *, *, #35614, .T. ) ;
#8746=CARTESIAN_POINT ( 'NONE',  ( 11.09999999999999964, -0.5000000000000000000, -5.124965750789000296 ) ) ;
#8754=CARTESIAN_POINT ( 'NONE',  ( 11.09999999999999964, 0.000000000000000000, 0.000000000000000000 ) ) ;
#8755=CARTESIAN_POINT ( 'NONE',  ( 8.566230646795000681, -5.212258818969000451, 6.157189191035000064 ) ) ;
#8760=CARTESIAN_POINT ( 'NONE',  ( 7.451068553725185062, -2.261323975060523850, 7.457013478475167823 ) ) ;
#8767=CARTESIAN_POINT ( 'NONE',  ( 10.84530628050273293, -5.097570467516499448, 5.114908450777414295 ) ) ;
#8774=CARTESIAN_POINT ( 'NONE',  ( 11.03776785110999903, -5.237767851104999650, 6.571291218949999902 ) ) ;
#8786=CARTESIAN_POINT ( 'NONE',  ( 9.903944471677000649, -5.205019707614999547, 6.747219600580999455 ) ) ;
#8789=CARTESIAN_POINT ( 'NONE',  ( 10.79839246847000034, -5.269358106415999110, -6.148714306659999629 ) ) ;
#8794=CARTESIAN_POINT ( 'NONE',  ( 11.07074860546000039, -6.638029483401999720, -5.577172573415000834 ) ) ;
#8798=CARTESIAN_POINT ( 'NONE',  ( 10.71081754702595923, -3.646708176540920832, -8.814774986206142415 ) ) ;
#8806=ORIENTED_EDGE ( 'NONE', *, *, #13361, .F. ) ;
#8811=CARTESIAN_POINT ( 'NONE',  ( 10.22514748322304534, -2.649941783575446408, 7.500008211948054004 ) ) ;
#8815=CYLINDRICAL_SURFACE ( 'NONE', #46394, 1.099999999999999867 ) ;
#8826=CARTESIAN_POINT ( 'NONE',  ( 10.53138988903999973, -5.607755226963999640, 7.280101849877000042 ) ) ;
#8830=EDGE_CURVE ( 'NONE', #46950, #25841, #48528, .T. ) ;
#8831=CARTESIAN_POINT ( 'NONE',  ( 10.44080359545000114, -5.435731278187999393, 7.303630150377999009 ) ) ;
#8845=CARTESIAN_POINT ( 'NONE',  ( 9.306727112333998519, -4.009302068291999532, -9.043024413115999138 ) ) ;
#8853=EDGE_CURVE ( 'NONE', #57495, #51180, #69074, .T. ) ;
#8857=CARTESIAN_POINT ( 'NONE',  ( 8.539089945104535673, -4.176610156107928518, 8.851086029037793068 ) ) ;
#8859=ORIENTED_EDGE ( 'NONE', *, *, #61977, .T. ) ;
#8868=CARTESIAN_POINT ( 'NONE',  ( 10.16000000000000014, -4.496968146123999865, -8.755198255949000696 ) ) ;
#8872=EDGE_LOOP ( 'NONE', ( #52442, #32116, #26317, #65496, #53602 ) ) ;
#8880=EDGE_CURVE ( 'NONE', #63766, #67307, #55150, .T. ) ;
#8884=CARTESIAN_POINT ( 'NONE',  ( 9.049519800792998225, -8.676607829236999692, -6.163757080959000767 ) ) ;
#8888=CARTESIAN_POINT ( 'NONE',  ( 11.04678944127999962, -5.235596213805000509, -5.039805523473999571 ) ) ;
#8892=CARTESIAN_POINT ( 'NONE',  ( 10.72303951155000057, -3.890113427500999421, -8.859339185702999941 ) ) ;
#8894=ORIENTED_EDGE ( 'NONE', *, *, #25790, .T. ) ;
#8906=CARTESIAN_POINT ( 'NONE',  ( 10.75775061949999944, -2.788892539766000045, -4.903545070807000528 ) ) ;
#8907=CARTESIAN_POINT ( 'NONE',  ( 9.441140818749000019, -4.011292643094999555, -9.373220388412001114 ) ) ;
#8909=B_SPLINE_CURVE_WITH_KNOTS ( 'NONE', 3,
 ( #61767, #34866, #56183, #45700, #13885, #67009, #9652, #68721, #20495, #202, #21521, #52651, #5783, #27126, #42854, #63476, #64165, #4746, #36231, #9999, #62788, #37265, #16279, #63127, #48443, #53003 ),
 .UNSPECIFIED., .F., .F.,
 ( 4, 2, 2, 2, 2, 2, 2, 2, 2, 2, 2, 2, 4 ),
 ( 0.000000000000000000, 0.06249999999999986122, 0.1249999999999997224, 0.2499999999999992506, 0.3749999999999987788, 0.4999999999999983347, 0.6249999999999978906, 0.6874999999999977796, 0.7499999999999977796, 0.8124999999999983347, 0.8749999999999987788, 0.9374999999999993339, 1.000000000000000000 ),
 .UNSPECIFIED. ) ;
#8935=ORIENTED_EDGE ( 'NONE', *, *, #24998, .T. ) ;
#8936=CARTESIAN_POINT ( 'NONE',  ( 11.29621718459000057, -3.561654022787999807, 6.266039799355000106 ) ) ;
#8938=DIRECTION ( 'NONE',  ( 1.000000000000000000, 0.000000000000000000, 0.000000000000000000 ) ) ;
#8939=CARTESIAN_POINT ( 'NONE',  ( 7.507480646791999668, -3.501517589953999643, 9.055975309745999624 ) ) ;
#8943=CARTESIAN_POINT ( 'NONE',  ( 10.97807333593999957, -5.235090452703000885, -6.783100406990000053 ) ) ;
#8947=ORIENTED_EDGE ( 'NONE', *, *, #16170, .T. ) ;
#8948=CARTESIAN_POINT ( 'NONE',  ( 9.533427734455999669, -2.564762519363000148, 6.150594768287000136 ) ) ;
#8951=CARTESIAN_POINT ( 'NONE',  ( 10.88016425062000003, -2.793121555136000023, -6.864957546339999439 ) ) ;
#8958=EDGE_CURVE ( 'NONE', #26424, #55718, #60821, .T. ) ;
#8976=CARTESIAN_POINT ( 'NONE',  ( 11.09999999999999964, -2.488501404117073434, -6.685067957705506991 ) ) ;
#8988=CARTESIAN_POINT ( 'NONE',  ( 7.256081853207000165, -2.531197775378000170, 8.216705951490000714 ) ) ;
#8993=CARTESIAN_POINT ( 'NONE',  ( 11.09999999999999964, -7.940796613052000019, -6.945951997396999644 ) ) ;
#8998=VERTEX_POINT ( 'NONE', #39075 ) ;
#8999=CARTESIAN_POINT ( 'NONE',  ( 10.76685100253999927, -2.832432432432000269, 6.822293592207000934 ) ) ;
#9009=CARTESIAN_POINT ( 'NONE',  ( 8.210268599937796452, -5.723642697224037512, 7.747033231994619129 ) ) ;
#9013=CARTESIAN_POINT ( 'NONE',  ( 11.08464238854999984, -5.237407606198999588, -5.050454952618999904 ) ) ;
#9016=EDGE_CURVE ( 'NONE', #8185, #8090, #33836, .T. ) ;
#9019=CARTESIAN_POINT ( 'NONE',  ( 10.15291672334000062, -4.949038487346999915, -8.498994087616001281 ) ) ;
#9028=CARTESIAN_POINT ( 'NONE',  ( 9.406706853206999952, -3.705847642455000202, 9.096432253453999195 ) ) ;
#9030=ORIENTED_EDGE ( 'NONE', *, *, #46488, .F. ) ;
#9033=CARTESIAN_POINT ( 'NONE',  ( 10.66043185321000131, -2.315667072036000196, -7.431702410656999547 ) ) ;
#9043=ORIENTED_EDGE ( 'NONE', *, *, #48715, .T. ) ;
#9053=CARTESIAN_POINT ( 'NONE',  ( 11.09999999999999964, -4.000000000000000000, 7.500000000000000000 ) ) ;
#9057=CARTESIAN_POINT ( 'NONE',  ( 10.15670292967786104, -5.179682183662243311, -8.179940953559762917 ) ) ;
#9069=CARTESIAN_POINT ( 'NONE',  ( 9.220176149162259804, -2.652345172034098475, 7.581873905328563090 ) ) ;
#9073=EDGE_CURVE ( 'NONE', #16664, #4537, #11332, .T. ) ;
#9090=CARTESIAN_POINT ( 'NONE',  ( 7.475043146792000215, -3.276313010012999793, 5.841993238691999935 ) ) ;
#9091=VERTEX_POINT ( 'NONE', #34068 ) ;
#9095=CARTESIAN_POINT ( 'NONE',  ( 7.555344015604732455, -3.596964894108017230, 5.798493967524453119 ) ) ;
#9102=CARTESIAN_POINT ( 'NONE',  ( 10.64116087492386420, -5.048254848383018079, 5.053851215417545006 ) ) ;
#9114=CARTESIAN_POINT ( 'NONE',  ( 9.769471092180999960, -5.100000000000000533, -6.152188490330000370 ) ) ;
#9118=VECTOR ( 'NONE', #37243, 1000.000000000000000 ) ;
#9122=CARTESIAN_POINT ( 'NONE',  ( 10.09181272066999924, -2.440908155048000516, 7.817368209339999652 ) ) ;
#9124=CARTESIAN_POINT ( 'NONE',  ( 10.05204995789999955, -2.669899884077999719, -8.791535702747999892 ) ) ;
#9129=CARTESIAN_POINT ( 'NONE',  ( 10.35646369189390192, -5.100000000000000533, 6.665341197326519307 ) ) ;
#9136=CYLINDRICAL_SURFACE ( 'NONE', #24421, 1.350000000000000089 ) ;
#9137=ORIENTED_EDGE ( 'NONE', *, *, #27535, .T. ) ;
#9148=CARTESIAN_POINT ( 'NONE',  ( 5.700000000000000178, -1.433333333332999837, -10.65401593558000037 ) ) ;
#9150=CARTESIAN_POINT ( 'NONE',  ( 9.663906509039998483, -2.491831134779999957, -6.388915175267000812 ) ) ;
#9158=CARTESIAN_POINT ( 'NONE',  ( 10.96291115432987340, -5.162911154332890717, -6.648309209561353406 ) ) ;
#9159=VERTEX_POINT ( 'NONE', #63361 ) ;
#9162=FACE_OUTER_BOUND ( 'NONE', #49547, .T. ) ;
#9171=CARTESIAN_POINT ( 'NONE',  ( 10.60267905665539523, -5.009718911382226025, -5.031837394736871083 ) ) ;
#9180=FACE_OUTER_BOUND ( 'NONE', #13174, .T. ) ;
#9188=CARTESIAN_POINT ( 'NONE',  ( 9.219210542222684879, -4.353245349593146685, -8.814482920002204125 ) ) ;
#9198=ORIENTED_EDGE ( 'NONE', *, *, #36321, .T. ) ;
#9210=DIRECTION ( 'NONE',  ( -1.000000000000000000, 0.000000000000000000, 0.000000000000000000 ) ) ;
#9211=EDGE_CURVE ( 'NONE', #16713, #61413, #46580, .T. ) ;
#9213=CARTESIAN_POINT ( 'NONE',  ( 10.99698512684000029, -8.058258747261000110, -7.169000291589999740 ) ) ;
#9217=CARTESIAN_POINT ( 'NONE',  ( 8.174990947233128580, -2.650692654197974729, 7.500004443805800669 ) ) ;
#9233=CARTESIAN_POINT ( 'NONE',  ( 8.833308238655002143, -4.875955647784997460, -6.190001260256996929 ) ) ;
#9234=ORIENTED_EDGE ( 'NONE', *, *, #64028, .T. ) ;
#9237=CARTESIAN_POINT ( 'NONE',  ( 10.31495997652000085, -3.356726044455999425, -4.564232296395000610 ) ) ;
#9238=CARTESIAN_POINT ( 'NONE',  ( 9.793154437819998392, -5.792391408692000532, -6.955579396894000510 ) ) ;
#9244=CARTESIAN_POINT ( 'NONE',  ( 8.251326917914997949, -4.957166827433998613, 6.172577619222003875 ) ) ;
#9246=EDGE_CURVE ( 'NONE', #25113, #48331, #65727, .T. ) ;
#9258=SHAPE_DEFINITION_REPRESENTATION ( #13187, #30050 ) ;
#9264=CARTESIAN_POINT ( 'NONE',  ( 9.757667269575000191, -4.489271889653999814, 5.986031004145000445 ) ) ;
#9266=CARTESIAN_POINT ( 'NONE',  ( 8.505089800085370300, -3.298395928475978511, 5.974470256167060178 ) ) ;
#9267=CARTESIAN_POINT ( 'NONE',  ( 9.566483607044000692, -4.108965473266000146, 8.851626696081998702 ) ) ;
#9281=ORIENTED_EDGE ( 'NONE', *, *, #14470, .T. ) ;
#9284=CARTESIAN_POINT ( 'NONE',  ( 9.258050732556000639, -4.895927245463000510, -6.008721945297999412 ) ) ;
#9304=CARTESIAN_POINT ( 'NONE',  ( 9.843620110012999191, -5.021680390140000227, -8.761463725090999688 ) ) ;
#9306=CARTESIAN_POINT ( 'NONE',  ( 9.005622771607709964, -5.254628312680063473, 7.997745863565469904 ) ) ;
#9323=CARTESIAN_POINT ( 'NONE',  ( 8.320870559624999885, -3.894643656844000379, 6.044452984962999764 ) ) ;
#9339=CARTESIAN_POINT ( 'NONE',  ( 7.835503439526941172, -4.950930448547884666, 6.483249265681529927 ) ) ;
#9341=CARTESIAN_POINT ( 'NONE',  ( 8.099647544207300598, -4.546102203237349038, 5.848288472323551090 ) ) ;
#9345=CARTESIAN_POINT ( 'NONE',  ( 11.13224971717000145, -5.325575099955998759, -4.980474265038999704 ) ) ;
#9350=VERTEX_POINT ( 'NONE', #54607 ) ;
#9351=CARTESIAN_POINT ( 'NONE',  ( 9.523148997461001741, -5.167567567567999731, -6.822293592207000934 ) ) ;
#9352=CARTESIAN_POINT ( 'NONE',  ( 10.98768577056000062, -2.700436730051000378, -4.945210085382000464 ) ) ;
#9358=ORIENTED_EDGE ( 'NONE', *, *, #10950, .T. ) ;
#9365=CARTESIAN_POINT ( 'NONE',  ( 10.47111935320999976, -5.170637620872999385, -8.712950754783999940 ) ) ;
#9370=AXIS2_PLACEMENT_3D ( 'NONE', #50309, #28648, #39126 ) ;
#9372=FACE_OUTER_BOUND ( 'NONE', #21580, .T. ) ;
#9377=ORIENTED_EDGE ( 'NONE', *, *, #224, .T. ) ;
#9381=CARTESIAN_POINT ( 'NONE',  ( 11.09999999999999964, -2.399999999999999911, 6.571291218949999902 ) ) ;
#9388=CARTESIAN_POINT ( 'NONE',  ( 10.81746213571000048, -5.100000000000000533, 6.571291218949999902 ) ) ;
#9398=EDGE_CURVE ( 'NONE', #57810, #22542, #51643, .T. ) ;
#9408=B_SPLINE_CURVE_WITH_KNOTS ( 'NONE', 3,
 ( #35527, #56848, #20122, #30287, #51590, #25026, #46357, #57518, #52281, #11688, #16247, #63449, #11345, #26757, #58214, #64133, #6098 ),
 .UNSPECIFIED., .F., .F.,
 ( 4, 2, 2, 2, 1, 2, 2, 2, 4 ),
 ( 0.000000000000000000, 0.2500000000000272560, 0.3750000000000394684, 0.4375000000000455747, 0.4687500000000475731, 0.4843750000000475731, 0.5000000000000476286, 0.7500000000000237588, 1.000000000000000000 ),
 .UNSPECIFIED. ) ;
#9414=CARTESIAN_POINT ( 'NONE',  ( 10.48170095836776028, -2.322637725008158238, 6.770404810779447224 ) ) ;
#9424=CARTESIAN_POINT ( 'NONE',  ( 7.886566940378000545, -3.084082018960999871, 9.259837032825000591 ) ) ;
#9429=CARTESIAN_POINT ( 'NONE',  ( 7.591617075526322367, -4.370784861422539080, 5.800362021175127225 ) ) ;
#9444=CIRCLE ( 'NONE', #6103, 0.8000000000000000444 ) ;
#9447=VERTEX_POINT ( 'NONE', #60893 ) ;
#9449=CARTESIAN_POINT ( 'NONE',  ( 9.652931135702420562, -5.100000000000000533, -6.444141223381761208 ) ) ;
#9450=ORIENTED_EDGE ( 'NONE', *, *, #30926, .T. ) ;
#9457=CARTESIAN_POINT ( 'NONE',  ( 10.46085355684000007, -5.403406918566000527, 7.721809917403000156 ) ) ;
#9465=CARTESIAN_POINT ( 'NONE',  ( 11.01655322883999943, -5.424331390032000044, -4.991943751707999866 ) ) ;
#9472=CARTESIAN_POINT ( 'NONE',  ( 10.18909467608999897, -5.907859813488999912, 7.801539220053999912 ) ) ;
#9479=CARTESIAN_POINT ( 'NONE',  ( 9.124702828701000357, -4.778665285493000070, 8.799745834808000211 ) ) ;
#9489=CARTESIAN_POINT ( 'NONE',  ( 9.265308298767999773, -5.700621988293000264, -7.339579610785999186 ) ) ;
#9498=ORIENTED_EDGE ( 'NONE', *, *, #62502, .F. ) ;
#9502=CARTESIAN_POINT ( 'NONE',  ( 9.447848023450999833, -5.447470167531999863, 7.431328114251999573 ) ) ;
#9507=DIRECTION ( 'NONE',  ( 1.000000000000000000, 0.000000000000000000, -5.786858783960000242E-14 ) ) ;
#9509=ORIENTED_EDGE ( 'NONE', *, *, #26997, .T. ) ;
#9515=CARTESIAN_POINT ( 'NONE',  ( 10.95359096189000070, -2.844919157736999882, 5.175303575009000845 ) ) ;
#9517=ADVANCED_FACE ( 'NONE', ( #34336 ), #46191, .T. ) ;
#9520=CARTESIAN_POINT ( 'NONE',  ( 10.88138019924999966, -2.936733240055999783, -5.079281455792999722 ) ) ;
#9523=AXIS2_PLACEMENT_3D ( 'NONE', #36406, #40618, #19644 ) ;
#9541=ORIENTED_EDGE ( 'NONE', *, *, #7524, .T. ) ;
#9562=CARTESIAN_POINT ( 'NONE',  ( 8.060295491240839993, -3.823126980273272579, 8.848192560902774062 ) ) ;
#9567=CARTESIAN_POINT ( 'NONE',  ( 10.21238410957999854, -4.072568653311000375, -8.861841462475000597 ) ) ;
#9578=CARTESIAN_POINT ( 'NONE',  ( 7.722414202460995192, -2.834216095980001349, 6.826613447391997269 ) ) ;
#9581=AXIS2_PLACEMENT_3D ( 'NONE', #28876, #50184, #44947 ) ;
#9582=FACE_OUTER_BOUND ( 'NONE', #45929, .T. ) ;
#9589=CARTESIAN_POINT ( 'NONE',  ( 7.802608290491005683, -4.876635182444005068, 6.352765399118998069 ) ) ;
#9601=CARTESIAN_POINT ( 'NONE',  ( 7.100000000000000533, -4.000000000000000000, 8.849999999999999645 ) ) ;
#9602=CARTESIAN_POINT ( 'NONE',  ( 9.035438658680838842, -2.896181042233768377, -6.646458295446667108 ) ) ;
#9603=ORIENTED_EDGE ( 'NONE', *, *, #46926, .F. ) ;
#9604=CARTESIAN_POINT ( 'NONE',  ( -15.86200481174999943, -5.599999999999999645, -6.571291218949999902 ) ) ;
#9612=CARTESIAN_POINT ( 'NONE',  ( 11.18706725482999964, -3.186788126275999833, 6.232699537089999353 ) ) ;
#9614=CARTESIAN_POINT ( 'NONE',  ( 8.506326034927656821, -3.199837828248755844, 6.012289131673731468 ) ) ;
#9615=CARTESIAN_POINT ( 'NONE',  ( 9.278331853207999913, -5.791549888895000109, 7.752110689268000954 ) ) ;
#9623=EDGE_LOOP ( 'NONE', ( #1117, #23046, #11223, #23625, #7759 ) ) ;
#9638=CARTESIAN_POINT ( 'NONE',  ( 7.881897435323000245, -5.128252730674000226, 6.737016898340999482 ) ) ;
#9642=CARTESIAN_POINT ( 'NONE',  ( 7.674540706797001732, -4.591334964886001124, 6.448517731106997886 ) ) ;
#9652=CARTESIAN_POINT ( 'NONE',  ( 9.576555093678434716, -2.247948244796866835, -7.800247541287225417 ) ) ;
#9659=CARTESIAN_POINT ( 'NONE',  ( 11.04678944127999962, -5.235596213805000509, -5.039805523473999571 ) ) ;
#9666=CARTESIAN_POINT ( 'NONE',  ( 9.472537864290000442, -2.899999999999999911, -6.571291218949999902 ) ) ;
#9669=CARTESIAN_POINT ( 'NONE',  ( 7.577019353207000485, -5.480312458445999901, 8.192326492433998908 ) ) ;
#9676=AXIS2_PLACEMENT_3D ( 'NONE', #40345, #19020, #18341 ) ;
#9679=VERTEX_POINT ( 'NONE', #3441 ) ;
#9685=AXIS2_PLACEMENT_3D ( 'NONE', #24663, #29928, #51908 ) ;
#9692=CARTESIAN_POINT ( 'NONE',  ( 8.093953312661190225, -4.429161490856333039, 5.814587964491527039 ) ) ;
#9696=CARTESIAN_POINT ( 'NONE',  ( 10.37122190540000055, -4.584050552809999068, -5.010296351866999842 ) ) ;
#9702=CARTESIAN_POINT ( 'NONE',  ( 9.668897997121000287, -4.730747404809998891, -8.668230005597001409 ) ) ;
#9703=CARTESIAN_POINT ( 'NONE',  ( 9.050000000000000711, 0.000000000000000000, -4.000000000000000000 ) ) ;
#9712=CARTESIAN_POINT ( 'NONE',  ( 8.545870559624999530, -3.856773448568000084, 5.521258396339000285 ) ) ;
#9714=ORIENTED_EDGE ( 'NONE', *, *, #66043, .T. ) ;
#9722=CARTESIAN_POINT ( 'NONE',  ( 8.498030440990834933, -5.100000000000000533, 6.489929440899814495 ) ) ;
#9725=DIRECTION ( 'NONE',  ( 0.000000000000000000, -1.000000000000000000, 0.000000000000000000 ) ) ;
#9727=DIRECTION ( 'NONE',  ( 1.000000000000000000, 0.000000000000000000, 0.000000000000000000 ) ) ;
#9730=EDGE_CURVE ( 'NONE', #68446, #14991, #52022, .T. ) ;
#9739=ORIENTED_EDGE ( 'NONE', *, *, #26547, .F. ) ;
#9752=CARTESIAN_POINT ( 'NONE',  ( 9.136334870123905105, -3.395591289844346328, 8.727132796763758193 ) ) ;
#9765=FACE_OUTER_BOUND ( 'NONE', #51283, .T. ) ;
#9768=B_SPLINE_CURVE_WITH_KNOTS ( 'NONE', 3,
 ( #68036, #19465, #14229, #3715, #40441, #67685, #9306, #40117, #19811, #50942, #18787, #66667, #7947, #14572, #57203, #29980, #4057, #25392, #20152, #61086, #29284, #24369, #50598, #2700, #45359 ),
 .UNSPECIFIED., .F., .F.,
 ( 4, 2, 2, 2, 2, 2, 2, 2, 2, 1, 2, 2, 4 ),
 ( 0.2955573413587750942, 0.4716680060191286161, 0.4936818391016731256, 0.5156956721842176350, 0.5597233383493066539, 0.6477786706794828042, 0.7358340030096590656, 0.7468409195509307930, 0.7523443778215666011, 0.7578478360922024093, 0.7798616691747313201, 0.8238893353397851449, 1.000000000000000000 ),
 .UNSPECIFIED. ) ;
#9772=CARTESIAN_POINT ( 'NONE',  ( 9.143918146793000190, -5.791549888895000109, 7.752110689268000954 ) ) ;
#9778=CARTESIAN_POINT ( 'NONE',  ( 10.91060805961999947, -4.702347118766000200, -9.210032991522000501 ) ) ;
#9779=CARTESIAN_POINT ( 'NONE',  ( 7.495957138799123065, -2.535418675573966052, 6.532461274932616746 ) ) ;
#9783=ORIENTED_EDGE ( 'NONE', *, *, #15355, .T. ) ;
#9794=EDGE_CURVE ( 'NONE', #34400, #14644, #42919, .T. ) ;
#9804=CARTESIAN_POINT ( 'NONE',  ( 10.27335506660999975, -4.750713325691999778, 4.596758554457999857 ) ) ;
#9809=CARTESIAN_POINT ( 'NONE',  ( 10.02202195053999922, -3.298019507654999849, 5.700533868754000366 ) ) ;
#9814=CARTESIAN_POINT ( 'NONE',  ( 10.90454231406000041, -5.099691312770999296, -5.130383474399000221 ) ) ;
#9822=CARTESIAN_POINT ( 'NONE',  ( 9.632185590920999019, -5.638162562978999759, 6.476633609657000079 ) ) ;
#9823=EDGE_CURVE ( 'NONE', #60343, #11189, #616, .T. ) ;
#9830=CARTESIAN_POINT ( 'NONE',  ( 9.972852379787999766, -5.044471434015000533, 6.258101649750000384 ) ) ;
#9835=B_SPLINE_CURVE_WITH_KNOTS ( 'NONE', 3,
 ( #43641, #48190, #48883, #59710 ),
 .UNSPECIFIED., .F., .F.,
 ( 4, 4 ),
 ( 0.000000000000000000, 1.000000000000000000 ),
 .UNSPECIFIED. ) ;
#9852=CARTESIAN_POINT ( 'NONE',  ( 10.50286331871000023, -5.158900740613000302, 8.369962360110999811 ) ) ;
#9858=CARTESIAN_POINT ( 'NONE',  ( 9.523148997461001741, -5.167567567567999731, -6.822293592207000934 ) ) ;
#9871=CARTESIAN_POINT ( 'NONE',  ( 10.95383834890000152, -2.844912728619000131, -5.168232267893999143 ) ) ;
#9872=CARTESIAN_POINT ( 'NONE',  ( 11.02419555961999897, -2.407899345275000158, -8.439548421502999886 ) ) ;
#9873=CARTESIAN_POINT ( 'NONE',  ( 9.090964864865910045, -3.294502121218175983, 8.704449896995548386 ) ) ;
#9877=CARTESIAN_POINT ( 'NONE',  ( 9.087099331641999456, -5.286372936495260966, -7.026974105800379178 ) ) ;
#9883=ORIENTED_EDGE ( 'NONE', *, *, #68032, .F. ) ;
#9884=CYLINDRICAL_SURFACE ( 'NONE', #27283, 0.4999999999999998335 ) ;
#9913=CARTESIAN_POINT ( 'NONE',  ( 7.924878289113923557, -5.349357204871147076, 7.500005630225521358 ) ) ;
#9917=CARTESIAN_POINT ( 'NONE',  ( 10.44807121817999906, -3.684978196963999864, -6.173109031625999776 ) ) ;
#9930=CARTESIAN_POINT ( 'NONE',  ( 7.411085905969002852, -3.233236485764999113, 6.481842843012996624 ) ) ;
#9933=CARTESIAN_POINT ( 'NONE',  ( 7.666438387056996540, -3.213133027605000525, 6.349775630263004622 ) ) ;
#9934=CARTESIAN_POINT ( 'NONE',  ( 9.624896294737000702, -5.235394649229000663, -8.110359502241001550 ) ) ;
#9937=CARTESIAN_POINT ( 'NONE',  ( 10.06343867337000120, -5.156226070197000411, 6.125223053176999777 ) ) ;
#9942=DIRECTION ( 'NONE',  ( -1.000000000000000000, 0.000000000000000000, 0.000000000000000000 ) ) ;
#9957=CARTESIAN_POINT ( 'NONE',  ( 9.584226531641581559, -2.899999999999999911, 6.304440313841762844 ) ) ;
#9964=CARTESIAN_POINT ( 'NONE',  ( 10.35616740164000049, -2.777283710737999733, 8.995265811011998736 ) ) ;
#9967=DIRECTION ( 'NONE',  ( 0.000000000000000000, -0.8648648648648717963, 0.5020047465136829867 ) ) ;
#9968=CARTESIAN_POINT ( 'NONE',  ( 9.342519353207999089, -5.057079407184000175, 8.967634647348999621 ) ) ;
#9970=ORIENTED_EDGE ( 'NONE', *, *, #29481, .F. ) ;
#9976=CARTESIAN_POINT ( 'NONE',  ( 10.43579701286999928, -2.587605342384000195, 6.390039770907999461 ) ) ;
#9982=LINE ( 'NONE', #183, #62188 ) ;
#9989=CARTESIAN_POINT ( 'NONE',  ( 9.959635380193999410, -5.406637819064000539, 7.700301345050000634 ) ) ;
#9991=FACE_OUTER_BOUND ( 'NONE', #53822, .T. ) ;
#9994=CARTESIAN_POINT ( 'NONE',  ( 10.98768553379999879, -5.299329486732999861, 4.945210549701000602 ) ) ;
#9999=CARTESIAN_POINT ( 'NONE',  ( 9.324996057314875131, -5.719375876571866968, -7.175980490421300040 ) ) ;
#10007=CARTESIAN_POINT ( 'NONE',  ( 7.218293146793000048, -4.773080213113000347, 8.927399220053999329 ) ) ;
#10016=CARTESIAN_POINT ( 'NONE',  ( 10.98768472633000037, -6.720753151621999599, -5.471698430863999540 ) ) ;
#10019=CARTESIAN_POINT ( 'NONE',  ( 7.326308059621999824, -3.394845988290999816, 9.388942682504000103 ) ) ;
#10025=EDGE_CURVE ( 'NONE', #49363, #20272, #7238, .T. ) ;
#10038=CARTESIAN_POINT ( 'NONE',  ( 8.151588397734400360, -5.460081713051196495, 6.513119554412222456 ) ) ;
#10040=ORIENTED_EDGE ( 'NONE', *, *, #28810, .F. ) ;
#10045=EDGE_CURVE ( 'NONE', #39230, #46950, #43747, .T. ) ;
#10050=B_SPLINE_CURVE_WITH_KNOTS ( 'NONE', 3,
 ( #45388, #66699, #18821, #40146, #30343, #69106, #47446, #4090, #19843, #31370, #31713, #42542 ),
 .UNSPECIFIED., .F., .F.,
 ( 4, 2, 1, 1, 2, 2, 4 ),
 ( 0.000000000000000000, 0.2500000000000195954, 0.3750000000000261458, 0.4375000000000285327, 0.4687500000000288103, 0.5000000000000290878, 1.000000000000000000 ),
 .UNSPECIFIED. ) ;
#10051=CARTESIAN_POINT ( 'NONE',  ( 9.507558421712998253, -4.699533657262000119, -6.366989705700999203 ) ) ;
#10055=CARTESIAN_POINT ( 'NONE',  ( 4.000000000000000000, 0.000000000000000000, 0.000000000000000000 ) ) ;
#10101=CARTESIAN_POINT ( 'NONE',  ( 9.160381251338680642, -3.070110540811217703, 8.479443955494096130 ) ) ;
#10107=LINE ( 'NONE', #63924, #50778 ) ;
#10116=UNCERTAINTY_MEASURE_WITH_UNIT (LENGTH_MEASURE( 1.000000000000000082E-05 ), #20568, 'distance_accuracy_value', 'NONE');
#10124=CARTESIAN_POINT ( 'NONE',  ( -15.86200481174999943, -2.399999999999999911, 6.571291218949999902 ) ) ;
#10125=CARTESIAN_POINT ( 'NONE',  ( 8.283081853209001366, -2.376522687267000222, 7.686981355459999499 ) ) ;
#10126=ORIENTED_EDGE ( 'NONE', *, *, #10950, .F. ) ;
#10130=CARTESIAN_POINT ( 'NONE',  ( 7.472002294636990172, -2.326570465340251026, 7.022491050036767213 ) ) ;
#10151=DIRECTION ( 'NONE',  ( 1.654177832420999993E-10, 1.654177150564999918E-10, 1.000000000000000000 ) ) ;
#10156=CARTESIAN_POINT ( 'NONE',  ( 10.58728840301827923, -2.899999999999999911, -6.305985889763610963 ) ) ;
#10159=CARTESIAN_POINT ( 'NONE',  ( 10.39106278671000005, -4.025320977579999848, 9.261121875182000807 ) ) ;
#10174=LINE ( 'NONE', #41990, #56020 ) ;
#10182=CARTESIAN_POINT ( 'NONE',  ( 11.15982711745999900, -5.578228817597000955, 8.067792329320999656 ) ) ;
#10188=CARTESIAN_POINT ( 'NONE',  ( 9.397313405920000307, -4.010297355695000121, -9.208122400763999238 ) ) ;
#10192=ADVANCED_FACE ( 'NONE', ( #36560 ), #57885, .F. ) ;
#10195=CARTESIAN_POINT ( 'NONE',  ( 10.90145065189000029, -2.900000000488999863, 5.151029872614000027 ) ) ;
#10217=CARTESIAN_POINT ( 'NONE',  ( 10.98633305961999973, -3.015090804604000141, -9.064432363387998848 ) ) ;
#10221=CARTESIAN_POINT ( 'NONE',  ( 10.45746213570999927, -5.100000000000000533, -6.571291218949999902 ) ) ;
#10243=ORIENTED_EDGE ( 'NONE', *, *, #44598, .F. ) ;
#10252=VERTEX_POINT ( 'NONE', #49112 ) ;
#10255=CARTESIAN_POINT ( 'NONE',  ( 8.029017301488174496, -4.353549739959088782, 8.815463536202724271 ) ) ;
#10261=CARTESIAN_POINT ( 'NONE',  ( 10.52663358771999924, -4.933730002636999679, -6.506004698255999585 ) ) ;
#10263=ORIENTED_EDGE ( 'NONE', *, *, #19823, .T. ) ;
#10265=DIRECTION ( 'NONE',  ( 0.000000000000000000, -0.1333333333333049375, -0.9910712498212375099 ) ) ;
#10272=CARTESIAN_POINT ( 'NONE',  ( 10.26648554153000070, -3.436497692079999666, 4.689477345002000419 ) ) ;
#10273=CARTESIAN_POINT ( 'NONE',  ( 8.030239402831002238, -2.905307396403002507, 6.399703979581998325 ) ) ;
#10274=VERTEX_POINT ( 'NONE', #60641 ) ;
#10277=CARTESIAN_POINT ( 'NONE',  ( 8.437014469680988782, -2.901284097310000920, 6.624005965434003329 ) ) ;
#10280=CARTESIAN_POINT ( 'NONE',  ( 10.87021507563000000, -2.226042145532000305, 7.782753277595999997 ) ) ;
#10284=CARTESIAN_POINT ( 'NONE',  ( 7.696680409794002919, -4.865376733307997803, 6.399695646141002392 ) ) ;
#10293=CARTESIAN_POINT ( 'NONE',  ( 8.227533346878596276, -4.737976145727974320, 6.141445531791949186 ) ) ;
#10295=CARTESIAN_POINT ( 'NONE',  ( 7.175632800635331598, -4.000032153724883521, 8.979538128313718559 ) ) ;
#10304=AXIS2_PLACEMENT_3D ( 'NONE', #56708, #45187, #39943 ) ;
#10306=CARTESIAN_POINT ( 'NONE',  ( 9.743567407955000093, -5.287392049455999832, 8.939957179821000466 ) ) ;
#10310=CARTESIAN_POINT ( 'NONE',  ( 8.379706853209000883, -4.282999948634999221, 9.286791354293999490 ) ) ;
#10320=CARTESIAN_POINT ( 'NONE',  ( 9.600494040286998043, -5.206548117663999165, 8.585114612872999373 ) ) ;
#10322=DIRECTION ( 'NONE',  ( 1.000000000000000000, 0.000000000000000000, 0.000000000000000000 ) ) ;
#10324=CARTESIAN_POINT ( 'NONE',  ( 10.98768472625999948, -5.449702614167000192, -4.945212061590999575 ) ) ;
#10335=CARTESIAN_POINT ( 'NONE',  ( 7.591287949680001645, -4.587787988499997915, 6.499994349715005448 ) ) ;
#10340=CARTESIAN_POINT ( 'NONE',  ( 9.115000000004000569, -5.349999999999999645, -7.500000000000000000 ) ) ;
#10343=CARTESIAN_POINT ( 'NONE',  ( 9.393246442089999704, -5.100000000000000533, -6.421387671005999387 ) ) ;
#10347=ORIENTED_EDGE ( 'NONE', *, *, #16560, .T. ) ;
#10352=CARTESIAN_POINT ( 'NONE',  ( 7.731793146792000471, -4.580607464247000493, 9.213361409141999303 ) ) ;
#10354=CARTESIAN_POINT ( 'NONE',  ( 7.890669427268998781, -4.660296165433000404, 6.322498843348999920 ) ) ;
#10364=CARTESIAN_POINT ( 'NONE',  ( 8.443894353209000059, -2.905864338704999827, 8.940687151810998046 ) ) ;
#10377=DIRECTION ( 'NONE',  ( 0.5000000000000169864, 0.000000000000000000, 0.8660254037844288266 ) ) ;
#10379=ORIENTED_EDGE ( 'NONE', *, *, #2692, .T. ) ;
#10382=CARTESIAN_POINT ( 'NONE',  ( 8.382401718153786874, -2.849781230174281532, 8.805156601495802704 ) ) ;
#10383=CARTESIAN_POINT ( 'NONE',  ( 10.92328601976000080, -8.084347899873000287, 7.050238229386000199 ) ) ;
#10389=CARTESIAN_POINT ( 'NONE',  ( 7.726719819322242166, -3.010539059095759029, 6.557630456826268883 ) ) ;
#10390=DIRECTION ( 'NONE',  ( 0.000000000000000000, 0.000000000000000000, -1.000000000000000000 ) ) ;
#10404=CARTESIAN_POINT ( 'NONE',  ( 11.09049845538999968, -5.289010560972999819, 5.109759112891000044 ) ) ;
#10408=DIRECTION ( 'NONE',  ( 1.000000000000000000, 0.000000000000000000, 0.000000000000000000 ) ) ;
#10427=CARTESIAN_POINT ( 'NONE',  ( 8.654133428465479838, -4.873369502965289257, -6.470443573412346439 ) ) ;
#10436=EDGE_CURVE ( 'NONE', #46074, #28855, #43643, .T. ) ;
#10460=CARTESIAN_POINT ( 'NONE',  ( 10.25888544622000076, -4.512389816463000081, 5.993697694029000544 ) ) ;
#10461=CARTESIAN_POINT ( 'NONE',  ( 7.486433059621999675, -5.321924421352999701, 8.118250081378000971 ) ) ;
#10465=CARTESIAN_POINT ( 'NONE',  ( 10.98633305961999973, -3.015090804604000141, -9.064432363387998848 ) ) ;
#10466=CARTESIAN_POINT ( 'NONE',  ( 7.613456797751473992, -4.810924280407760989, 5.960869268491793882 ) ) ;
#10476=EDGE_CURVE ( 'NONE', #32830, #27541, #38979, .T. ) ;
#10479=CARTESIAN_POINT ( 'NONE',  ( 8.470944094208999076, -5.100000000000000533, 6.571291218949999902 ) ) ;
#10496=CARTESIAN_POINT ( 'NONE',  ( 11.18706725482999964, -3.186788126275999833, 6.232699537089999353 ) ) ;
#10502=B_SPLINE_CURVE_WITH_KNOTS ( 'NONE', 3,
 ( #5846, #48506, #611, #64567 ),
 .UNSPECIFIED., .F., .F.,
 ( 4, 4 ),
 ( 0.000000000000000000, 1.000000000000000000 ),
 .UNSPECIFIED. ) ;
#10513=VERTEX_POINT ( 'NONE', #63291 ) ;
#10517=CARTESIAN_POINT ( 'NONE',  ( 9.696086916451999826, -2.554404004330999900, 7.600685922079000179 ) ) ;
#10519=ADVANCED_FACE ( 'NONE', ( #62942 ), #57708, .F. ) ;
#10535=AXIS2_PLACEMENT_3D ( 'NONE', #35223, #12511, #33843 ) ;
#10538=CARTESIAN_POINT ( 'NONE',  ( 10.19256470245000123, -2.560274838243000062, 7.664550593243999899 ) ) ;
#10542=CARTESIAN_POINT ( 'NONE',  ( 10.45746213570999927, -5.100000000000000533, -6.571291218949999902 ) ) ;
#10544=EDGE_LOOP ( 'NONE', ( #69001, #35232, #553, #51402 ) ) ;
#10552=CARTESIAN_POINT ( 'NONE',  ( 10.38462472191413255, -2.899999999999999911, 6.445686799157043012 ) ) ;
#10553=VECTOR ( 'NONE', #53676, 1000.000000000000000 ) ;
#10574=CYLINDRICAL_SURFACE ( 'NONE', #26633, 1.350000000000000089 ) ;
#10601=CARTESIAN_POINT ( 'NONE',  ( 10.22440803363000050, -5.317414323721999736, -8.272454209812998727 ) ) ;
#10607=DIRECTION ( 'NONE',  ( 0.000000000000000000, 0.8648648648648470383, -0.5020047465137256193 ) ) ;
#10617=CARTESIAN_POINT ( 'NONE',  ( 7.555544676565999040, -2.930005555947998275, 6.552699291324001862 ) ) ;
#10620=CARTESIAN_POINT ( 'NONE',  ( 9.967845797207999681, -2.034786297409000078, 7.636877353231999344 ) ) ;
#10639=CARTESIAN_POINT ( 'NONE',  ( 7.558872858590611088, -4.679401687839340518, 8.680096940894596713 ) ) ;
#10643=CARTESIAN_POINT ( 'NONE',  ( 10.85685100254000091, -2.832432432432000269, -6.822293592207000934 ) ) ;
#10644=DIRECTION ( 'NONE',  ( -0.8660254037844289376, 0.000000000000000000, 0.5000000000000169864 ) ) ;
#10647=CARTESIAN_POINT ( 'NONE',  ( 9.945535518573000999, -2.906050966242999856, 8.880386511481999534 ) ) ;
#10649=VERTEX_POINT ( 'NONE', #22371 ) ;
#10651=CARTESIAN_POINT ( 'NONE',  ( 7.903995559621998623, -2.095727472214000020, 8.056487497515000484 ) ) ;
#10659=ORIENTED_EDGE ( 'NONE', *, *, #21132, .F. ) ;
#10660=CARTESIAN_POINT ( 'NONE',  ( 9.877259503622999759, -2.207992199716000137, 7.624813542847999059 ) ) ;
#10663=VERTEX_POINT ( 'NONE', #43368 ) ;
#10666=CARTESIAN_POINT ( 'NONE',  ( 10.92546935320999957, -5.641520548727999795, -7.883473948564999390 ) ) ;
#10678=ORIENTED_EDGE ( 'NONE', *, *, #59344, .T. ) ;
#10687=CARTESIAN_POINT ( 'NONE',  ( 9.214598350284001427, -2.899999999999999911, -6.571291218949999902 ) ) ;
#10692=CARTESIAN_POINT ( 'NONE',  ( 9.341483607044001047, -4.148132978932999926, 9.337467253566000380 ) ) ;
#10703=VERTEX_POINT ( 'NONE', #38456 ) ;
#10704=CARTESIAN_POINT ( 'NONE',  ( 8.122956853208000538, -3.566638198986999964, 5.743608852252999775 ) ) ;
#10705=CARTESIAN_POINT ( 'NONE',  ( 8.705995559625000269, -2.542850487891999745, 7.419808283050000064 ) ) ;
#10713=ORIENTED_EDGE ( 'NONE', *, *, #10476, .F. ) ;
#10720=CARTESIAN_POINT ( 'NONE',  ( 7.837267527055786331, -4.794208482798125281, 6.382611110956646350 ) ) ;
#10721=ADVANCED_FACE ( 'NONE', ( #12582 ), #44060, .T. ) ;
#10724=CARTESIAN_POINT ( 'NONE',  ( 8.415023682605584199, -2.417956104865769618, 8.222459336996642776 ) ) ;
#10733=CARTESIAN_POINT ( 'NONE',  ( 9.865041550948088656, -2.650034642413194419, -7.500002425457253707 ) ) ;
#10761=CARTESIAN_POINT ( 'NONE',  ( 11.12438586031000121, -5.546372646562000241, -5.163676736721000360 ) ) ;
#10764=LINE ( 'NONE', #5522, #23298 ) ;
#10767=CARTESIAN_POINT ( 'NONE',  ( 10.40879003340999986, -3.093879171920000282, -6.480773124728999690 ) ) ;
#10771=ORIENTED_EDGE ( 'NONE', *, *, #60141, .T. ) ;
#10789=CARTESIAN_POINT ( 'NONE',  ( 9.925159544971000614, -4.365624317997999881, -9.242254741729000855 ) ) ;
#10802=ORIENTED_EDGE ( 'NONE', *, *, #46092, .F. ) ;
#10806=CARTESIAN_POINT ( 'NONE',  ( 11.18483536755999808, -2.599651619047000040, 7.740676724427999922 ) ) ;
#10807=CARTESIAN_POINT ( 'NONE',  ( 8.192495559623999668, -2.550228841911000188, 7.666975032000999946 ) ) ;
#10813=CARTESIAN_POINT ( 'NONE',  ( 10.39539435320999949, -5.667179153637999178, -7.250689665673000661 ) ) ;
#10814=CARTESIAN_POINT ( 'NONE',  ( 7.773757704034534477, -5.028764116645290549, 8.902433763654059362 ) ) ;
#10815=CARTESIAN_POINT ( 'NONE',  ( 9.877259503622999759, -2.207992199716000137, 7.624813542847999059 ) ) ;
#10835=EDGE_CURVE ( 'NONE', #2041, #33857, #55924, .T. ) ;
#10841=CARTESIAN_POINT ( 'NONE',  ( 10.55813551225999980, -2.466564559586000183, 6.633531786299999844 ) ) ;
#10854=AXIS2_PLACEMENT_3D ( 'NONE', #64032, #54596, #11247 ) ;
#10855=CARTESIAN_POINT ( 'NONE',  ( 9.231612022449091626, -2.652299246284962830, 7.391249027395923932 ) ) ;
#10866=ADVANCED_FACE ( 'NONE', ( #62189 ), #34612, .T. ) ;
#10871=DIRECTION ( 'NONE',  ( 0.000000000000000000, 0.000000000000000000, -1.000000000000000000 ) ) ;
#10876=LINE ( 'NONE', #17149, #61698 ) ;
#10897=EDGE_CURVE ( 'NONE', #47885, #49595, #60329, .T. ) ;
#10902=CARTESIAN_POINT ( 'NONE',  ( 9.317462135714000837, -5.100000000000000533, 6.571291218949999902 ) ) ;
#10903=CARTESIAN_POINT ( 'NONE',  ( 10.22094314679000071, -2.563075248996000255, -8.004105227364998854 ) ) ;
#10909=ORIENTED_EDGE ( 'NONE', *, *, #48802, .F. ) ;
#10917=DIRECTION ( 'NONE',  ( -0.7071067811864950592, 0.6115519262857961325, 0.3549707614102975417 ) ) ;
#10920=CARTESIAN_POINT ( 'NONE',  ( 8.704862649514634398, -2.649860810595624283, 7.852951878455955992 ) ) ;
#10925=CARTESIAN_POINT ( 'NONE',  ( 9.819572261909000233, -2.688237737290000151, -7.873041261681999359 ) ) ;
#10949=CARTESIAN_POINT ( 'NONE',  ( 9.910158555493998378, -2.531067292016000003, -7.917737669614999696 ) ) ;
#10950=EDGE_CURVE ( 'NONE', #1282, #61413, #35635, .T. ) ;
#10955=CARTESIAN_POINT ( 'NONE',  ( 11.09999999999999964, 0.000000000000000000, 0.000000000000000000 ) ) ;
#10966=ORIENTED_EDGE ( 'NONE', *, *, #35752, .F. ) ;
#10968=CARTESIAN_POINT ( 'NONE',  ( 7.682778389973002220, -3.526905737521000006, 6.475916620580998817 ) ) ;
#10969=CARTESIAN_POINT ( 'NONE',  ( 9.536892889968999754, -5.099406281193999746, -6.669356233738001016 ) ) ;
#10971=CARTESIAN_POINT ( 'NONE',  ( 9.939319226872999735, -2.638101016021999978, 6.328632621050000573 ) ) ;
#10980=ORIENTED_EDGE ( 'NONE', *, *, #65651, .T. ) ;
#10983=CARTESIAN_POINT ( 'NONE',  ( 6.799999999999999822, -9.295462635088998837, -5.399710584805999858 ) ) ;
#10996=CARTESIAN_POINT ( 'NONE',  ( 9.242349231304000767, -5.206700957550999931, 8.808818370147001531 ) ) ;
#10997=CARTESIAN_POINT ( 'NONE',  ( 10.90000000164000049, -2.899999999992999733, 5.160242739040000082 ) ) ;
#11000=CARTESIAN_POINT ( 'NONE',  ( 9.176355646795000709, -2.935738482289000029, 6.259841087764999479 ) ) ;
#11010=VERTEX_POINT ( 'NONE', #41553 ) ;
#11011=CARTESIAN_POINT ( 'NONE',  ( 9.414314870535999802, -3.941041813398000304, 5.878346364186999295 ) ) ;
#11016=CARTESIAN_POINT ( 'NONE',  ( 10.08211398012999993, -4.728049789772000189, -8.793977405422999993 ) ) ;
#11026=CARTESIAN_POINT ( 'NONE',  ( 9.299999999999998934, -4.537600397704999899, 9.154563893594000135 ) ) ;
#11045=CARTESIAN_POINT ( 'NONE',  ( 10.99934110471000004, -5.081022574063999819, 8.239050178861999640 ) ) ;
#11047=CARTESIAN_POINT ( 'NONE',  ( 9.015543146794000151, -4.175914961544999748, 5.699510287082000026 ) ) ;
#11051=DIRECTION ( 'NONE',  ( 1.000000000000000000, 0.000000000000000000, 0.000000000000000000 ) ) ;
#11059=CARTESIAN_POINT ( 'NONE',  ( 7.374102686541000651, -4.389298280625000714, 9.135255728583000945 ) ) ;
#11071=CARTESIAN_POINT ( 'NONE',  ( 7.950237460432950876, -4.863279781983014693, 6.348139858574191052 ) ) ;
#11076=CARTESIAN_POINT ( 'NONE',  ( 8.381225618344668504, -2.869678555928259378, 8.822438359558621102 ) ) ;
#11080=B_SPLINE_CURVE_WITH_KNOTS ( 'NONE', 3,
 ( #19774, #36193, #25017, #46348, #67650, #26052, #41100, #47381, #57505, #51922 ),
 .UNSPECIFIED., .F., .F.,
 ( 4, 2, 2, 2, 4 ),
 ( 0.2509294615239107684, 0.4381970961429330624, 0.6254647307619554120, 0.8127323653809777060, 1.000000000000000000 ),
 .UNSPECIFIED. ) ;
#11087=CARTESIAN_POINT ( 'NONE',  ( 10.26947109217999810, -5.100000000000000533, -6.152188490330000370 ) ) ;
#11088=CARTESIAN_POINT ( 'NONE',  ( 9.709999999999999076, -4.496968146123999865, -8.755198255949000696 ) ) ;
#11100=CARTESIAN_POINT ( 'NONE',  ( 10.10107565221251491, -5.349884357716051753, -7.263395957186704166 ) ) ;
#11106=B_SPLINE_CURVE_WITH_KNOTS ( 'NONE', 3,
 ( #60021, #1989, #22953, #12474 ),
 .UNSPECIFIED., .F., .F.,
 ( 4, 4 ),
 ( 0.000000000000000000, 1.000000000000000000 ),
 .UNSPECIFIED. ) ;
#11118=CARTESIAN_POINT ( 'NONE',  ( 10.48735240295000004, -4.351290250877999810, -6.182246784057000788 ) ) ;
#11126=EDGE_CURVE ( 'NONE', #15766, #52017, #18864, .T. ) ;
#11140=CARTESIAN_POINT ( 'NONE',  ( 11.09999999999999964, -2.646159083949000124, 6.745271721726000536 ) ) ;
#11142=ORIENTED_EDGE ( 'NONE', *, *, #57252, .T. ) ;
#11153=CARTESIAN_POINT ( 'NONE',  ( 10.87148543990999983, -5.567571293949000300, 7.772413914480000408 ) ) ;
#11154=CARTESIAN_POINT ( 'NONE',  ( 7.678995559621999867, -2.599231861044000169, 7.909347897884000389 ) ) ;
#11156=CARTESIAN_POINT ( 'NONE',  ( 8.198726617487999135, -3.399995262767999904, 6.142473321098000483 ) ) ;
#11158=CARTESIAN_POINT ( 'NONE',  ( 11.24323064679000161, -2.479730344050999680, -7.587230764681999418 ) ) ;
#11159=CARTESIAN_POINT ( 'NONE',  ( 7.848601693978649152, -3.465122274420019188, 9.162632088545951348 ) ) ;
#11160=CARTESIAN_POINT ( 'NONE',  ( 9.595487457706001422, -3.928425191288000384, 5.531324308465000783 ) ) ;
#11173=ORIENTED_EDGE ( 'NONE', *, *, #33081, .T. ) ;
#11174=CARTESIAN_POINT ( 'NONE',  ( 8.496691940379001551, -5.198566224659999513, 8.332559954171999905 ) ) ;
#11175=PLANE ( 'NONE',  #58078 ) ;
#11183=CARTESIAN_POINT ( 'NONE',  ( 11.00366278039000001, -2.264082614160999984, 7.798350693290999835 ) ) ;
#11189=VERTEX_POINT ( 'NONE', #26167 ) ;
#11191=DIRECTION ( 'NONE',  ( 0.000000000000000000, -0.8648648648648717963, 0.5020047465136829867 ) ) ;
#11203=EDGE_CURVE ( 'NONE', #31672, #15110, #10764, .T. ) ;
#11205=CARTESIAN_POINT ( 'NONE',  ( 9.374586245486254299, -4.497363021594377841, 9.030797514265954007 ) ) ;
#11209=B_SPLINE_SURFACE_WITH_KNOTS ( 'NONE', 3, 3, ( 
 ( #29253, #19775, #46349, #29602, #24680, #40407, #62075, #13515, #35519, #45999, #41101, #34835, #67651, #3344, #35854, #35178, #50905, #51249, #51582, #61394, #24335, #13851, #34500, #51923, #39735, #30278, #67311, #18753, #62416, #67999, #66973, #57170, #56147, #9267, #50562 ),
 ( #8596, #2662, #8939, #30609, #29946, #40752, #19429, #14191, #8255, #61052, #23990, #4020, #56841, #45667, #13172, #55813, #45325, #66634, #3002, #40085, #20115, #5412, #53650, #26053, #30959, #27090, #58207, #69039, #11000, #41444, #32341, #62752, #20803, #41783, #48405 ),
 ( #14871, #20456, #5746, #63088, #53309, #42136, #36194, #31997, #42818, #52614, #15212, #31644, #64126, #52273, #37228, #4368, #48064, #10310, #26748, #52967, #36539, #57864, #25702, #47034, #63786, #68337, #58546, #57506, #167, #5063, #15897, #9615, #9968, #21484, #26400 ),
 ( #47727, #31304, #36893, #21151, #47382, #4708, #42478, #68685, #63442, #16240, #15565, #10651, #37564, #58897, #27429, #60280, #55036, #11335, #39301, #22864, #7136, #1206, #60624, #55380, #32677, #22514, #1546, #34064, #49789, #38963, #17639, #12385, #16922, #54686, #12735 ) ),
 .UNSPECIFIED., .F., .F., .F.,
 ( 4, 4 ),
 ( 4, 1, 1, 1, 1, 1, 1, 1, 1, 1, 1, 1, 1, 1, 1, 1, 1, 1, 1, 1, 1, 1, 1, 1, 1, 1, 1, 1, 1, 1, 1, 1, 4 ),
 ( -0.1039086239011999951, 1.103908623900999864 ),
 ( -0.02000000000000000042, 0.01250000000000000069, 0.04499999999999999833, 0.07749999999999999944, 0.1100000000000000006, 0.1424999999999999878, 0.1749999999999999889, 0.2074999999999999900, 0.2399999999999999911, 0.2725000000000000200, 0.3049999999999999933, 0.3375000000000000222, 0.3699999999999999956, 0.4025000000000000244, 0.4349999999999999978, 0.4675000000000000266, 0.5000000000000000000, 0.5324999999999999734, 0.5649999999999999467, 0.5975000000000000311, 0.6300000000000000044, 0.6624999999999999778, 0.6949999999999999512, 0.7275000000000000355, 0.7600000000000000089, 0.7924999999999999822, 0.8249999999999999556, 0.8575000000000000400, 0.8900000000000000133, 0.9224999999999999867, 0.9549999999999999600, 0.9875000000000000444, 1.020000000000000018 ),
 .UNSPECIFIED. ) ;
#11223=ORIENTED_EDGE ( 'NONE', *, *, #69149, .T. ) ;
#11243=CARTESIAN_POINT ( 'NONE',  ( 10.90246814679000131, -4.554787328265999413, -6.081873034041000103 ) ) ;
#11247=DIRECTION ( 'NONE',  ( 0.000000000000000000, -0.8648648648648717963, 0.5020047465136829867 ) ) ;
#11248=ORIENTED_EDGE ( 'NONE', *, *, #24620, .F. ) ;
#11258=EDGE_CURVE ( 'NONE', #67334, #51763, #67948, .T. ) ;
#11264=CARTESIAN_POINT ( 'NONE',  ( 10.81362580514000094, -3.876947229615999913, -9.022210119840998743 ) ) ;
#11266=ORIENTED_EDGE ( 'NONE', *, *, #16823, .T. ) ;
#11274=CARTESIAN_POINT ( 'NONE',  ( 7.844724262280000637, -4.719412258162999585, 6.357657668295000342 ) ) ;
#11275=CARTESIAN_POINT ( 'NONE',  ( 11.27765354842000001, -3.273798832483999721, 6.368296067120999382 ) ) ;
#11276=CARTESIAN_POINT ( 'NONE',  ( 11.03776249210999971, -8.050323671732000363, -6.914613055281999543 ) ) ;
#11288=CARTESIAN_POINT ( 'NONE',  ( 11.03407957707000087, -2.992853177526999975, -9.056567163506000995 ) ) ;
#11305=CARTESIAN_POINT ( 'NONE',  ( 8.164796825344000197, -3.457406484157000026, 6.165651553258999940 ) ) ;
#11309=CARTESIAN_POINT ( 'NONE',  ( 10.21608469020999976, -5.961703525007000515, 7.319668113368000384 ) ) ;
#11310=CARTESIAN_POINT ( 'NONE',  ( 9.840770501363659051, -3.644193716302523089, 9.240192412087251839 ) ) ;
#11311=CARTESIAN_POINT ( 'NONE',  ( 9.674373738639999942, -2.899999999999999911, -6.185493860157000867 ) ) ;
#11331=CARTESIAN_POINT ( 'NONE',  ( 10.69031285273999821, -5.903020122789000013, 7.830708506196000229 ) ) ;
#11332=LINE ( 'NONE', #10997, #45636 ) ;
#11335=CARTESIAN_POINT ( 'NONE',  ( 8.289120559623999185, -4.310353212080000773, 9.459493062793997709 ) ) ;
#11345=CARTESIAN_POINT ( 'NONE',  ( 8.153325607601846770, -3.117005381769989647, 6.262142143703084862 ) ) ;
#11347=CARTESIAN_POINT ( 'NONE',  ( 10.65550933554000146, -4.237674644795000667, 9.105223721671999115 ) ) ;
#11369=CARTESIAN_POINT ( 'NONE',  ( 10.15402496696000156, -5.267980706381999667, 5.992344456606999437 ) ) ;
#11376=CARTESIAN_POINT ( 'NONE',  ( 9.820206362952999868, -3.883324525498000224, 6.055606607331999847 ) ) ;
#11378=CARTESIAN_POINT ( 'NONE',  ( 7.149102686541000118, -4.351670788182000038, 8.977200644264000218 ) ) ;
#11388=CARTESIAN_POINT ( 'NONE',  ( 10.35685100253999913, -2.832432432432000269, -6.822293592207000934 ) ) ;
#11391=VERTEX_POINT ( 'NONE', #24018 ) ;
#11392=CARTESIAN_POINT ( 'NONE',  ( 9.368918146792999835, -5.618388245857000030, 7.727743016644000207 ) ) ;
#11395=CARTESIAN_POINT ( 'NONE',  ( 9.112942518363999156, -5.100000000000000533, 6.192000867487999827 ) ) ;
#11399=AXIS2_PLACEMENT_3D ( 'NONE', #49911, #2363, #61092 ) ;
#11411=CARTESIAN_POINT ( 'NONE',  ( 8.541164872330046620, -3.301241083931813591, 5.907377702369386085 ) ) ;
#11413=ORIENTED_EDGE ( 'NONE', *, *, #43505, .T. ) ;
#11445=ORIENTED_EDGE ( 'NONE', *, *, #47919, .F. ) ;
#11454=CARTESIAN_POINT ( 'NONE',  ( 10.90000000016000037, -5.167567554889999748, 6.822293570050000255 ) ) ;
#11460=CARTESIAN_POINT ( 'NONE',  ( 10.07314899745999881, -5.167567567567999731, -6.822293592207000934 ) ) ;
#11487=CARTESIAN_POINT ( 'NONE',  ( 10.62792628238999981, -3.100579357212000176, 8.599905962393000536 ) ) ;
#11492=CARTESIAN_POINT ( 'NONE',  ( 11.28109314679000086, -2.660122028910999692, -6.904120269057000492 ) ) ;
#11493=CARTESIAN_POINT ( 'NONE',  ( 7.776208646924445134, -4.986279724221044596, 8.933337815283831418 ) ) ;
#11494=AXIS2_PLACEMENT_3D ( 'NONE', #67736, #35264, #51333 ) ;
#11495=CARTESIAN_POINT ( 'NONE',  ( 9.442841440870999747, -2.691258483914000355, 6.269525829285999663 ) ) ;
#11502=ORIENTED_EDGE ( 'NONE', *, *, #27535, .F. ) ;
#11505=EDGE_CURVE ( 'NONE', #66731, #41719, #46958, .T. ) ;
#11511=CARTESIAN_POINT ( 'NONE',  ( 9.202754440379999679, -2.542850487891999745, 7.419808283050000064 ) ) ;
#11519=CARTESIAN_POINT ( 'NONE',  ( 10.74600376124999990, -5.242711034443999552, 8.978690688221998784 ) ) ;
#11555=FACE_OUTER_BOUND ( 'NONE', #10544, .T. ) ;
#11572=DIRECTION ( 'NONE',  ( 1.000000000000000000, 0.000000000000000000, 0.000000000000000000 ) ) ;
#11578=CARTESIAN_POINT ( 'NONE',  ( 8.616995677562000466, -4.876077402042000131, 5.996974966533000106 ) ) ;
#11579=CARTESIAN_POINT ( 'NONE',  ( 10.92546935320999957, -5.641520548727999795, -7.883473948564999390 ) ) ;
#11599=CARTESIAN_POINT ( 'NONE',  ( 7.100000000000000533, -4.000000000000000000, 7.500000000000000000 ) ) ;
#11602=CARTESIAN_POINT ( 'NONE',  ( 10.22440803363000050, -5.317414323721999736, -8.272454209812998727 ) ) ;
#11618=CARTESIAN_POINT ( 'NONE',  ( 9.736871746126999128, -2.742172332680000046, 6.839224809731999422 ) ) ;
#11621=ORIENTED_EDGE ( 'NONE', *, *, #54695, .F. ) ;
#11629=CARTESIAN_POINT ( 'NONE',  ( 10.87695483801000051, -5.827068285690999438, -7.814745128155998977 ) ) ;
#11630=VERTEX_POINT ( 'NONE', #63815 ) ;
#11635=CARTESIAN_POINT ( 'NONE',  ( 8.560199822370993417, -3.014874134772824732, 6.139748469567640754 ) ) ;
#11642=CARTESIAN_POINT ( 'NONE',  ( 7.799092354096995194, -3.518505934209000152, 6.398021147088998717 ) ) ;
#11649=B_SPLINE_CURVE_WITH_KNOTS ( 'NONE', 3,
 ( #583, #21550, #6852, #42886 ),
 .UNSPECIFIED., .F., .F.,
 ( 4, 4 ),
 ( 0.000000000000000000, 1.000000000000000000 ),
 .UNSPECIFIED. ) ;
#11652=DIRECTION ( 'NONE',  ( 0.000000000000000000, 0.000000000000000000, -1.000000000000000000 ) ) ;
#11653=CARTESIAN_POINT ( 'NONE',  ( 10.59344961228999971, -5.297755890367000120, 8.474197994416998725 ) ) ;
#11662=DIRECTION ( 'NONE',  ( -1.000000000000000000, 0.000000000000000000, 0.000000000000000000 ) ) ;
#11669=EDGE_CURVE ( 'NONE', #11391, #34244, #41166, .T. ) ;
#11680=CARTESIAN_POINT ( 'NONE',  ( 6.976568042970999528, -9.209912048597001188, 5.193747272324000797 ) ) ;
#11688=CARTESIAN_POINT ( 'NONE',  ( 8.155132402557608629, -3.046310786074582833, 6.333683957159311539 ) ) ;
#11689=VERTEX_POINT ( 'NONE', #10340 ) ;
#11690=CARTESIAN_POINT ( 'NONE',  ( 9.034116535116000435, -4.695350938297000454, 8.660677768253002284 ) ) ;
#11691=DIRECTION ( 'NONE',  ( -1.000000000000000000, 0.000000000000000000, 0.000000000000000000 ) ) ;
#11695=CARTESIAN_POINT ( 'NONE',  ( 10.69015444038000062, -4.391267940138999570, -8.802346922965000431 ) ) ;
#11696=VERTEX_POINT ( 'NONE', #31676 ) ;
#11722=CARTESIAN_POINT ( 'NONE',  ( 7.550620559621999739, -4.468370631666999770, 8.882152684713000568 ) ) ;
#11728=CYLINDRICAL_SURFACE ( 'NONE', #22421, 1.350000000000000089 ) ;
#11731=EDGE_CURVE ( 'NONE', #56474, #5840, #64496, .T. ) ;
#11733=CARTESIAN_POINT ( 'NONE',  ( 11.10000000000000142, -5.582818908801700175, 7.477537682244628670 ) ) ;
#11736=CARTESIAN_POINT ( 'NONE',  ( 8.481683059623998489, -2.472358291268000219, 6.234202627038999189 ) ) ;
#11756=CARTESIAN_POINT ( 'NONE',  ( 8.439910304958656795, -2.270935633533203823, 7.713963258081458996 ) ) ;
#11757=CARTESIAN_POINT ( 'NONE',  ( 8.642077642326000841, -2.899999999999999911, 6.463854830420999953 ) ) ;
#11767=ORIENTED_EDGE ( 'NONE', *, *, #20396, .T. ) ;
#11787=DIRECTION ( 'NONE',  ( 1.000000000000000000, 0.000000000000000000, 0.000000000000000000 ) ) ;
#11800=CARTESIAN_POINT ( 'NONE',  ( 10.86493091395000121, -4.678465004315999209, -9.048463592221999363 ) ) ;
#11805=ORIENTED_EDGE ( 'NONE', *, *, #40874, .F. ) ;
#11818=CARTESIAN_POINT ( 'NONE',  ( 7.000000000000000000, 0.000000000000000000, 0.000000000000000000 ) ) ;
#11835=CARTESIAN_POINT ( 'NONE',  ( 10.90638082498000117, -5.227498618488000126, 6.784459667733999666 ) ) ;
#11836=CARTESIAN_POINT ( 'NONE',  ( 9.091120559621998609, -3.762710033898000184, 8.787827024292999667 ) ) ;
#11842=CARTESIAN_POINT ( 'NONE',  ( 11.03905685320999908, -3.855072944465999907, -9.179476187420998912 ) ) ;
#11843=CARTESIAN_POINT ( 'NONE',  ( 7.718572254375063224, -5.707929586103706043, 7.902141240677100775 ) ) ;
#11844=CARTESIAN_POINT ( 'NONE',  ( 10.77462219945999955, -5.575466189878000911, 8.682669263022999573 ) ) ;
#11849=AXIS2_PLACEMENT_3D ( 'NONE', #28577, #11787, #33126 ) ;
#11864=CARTESIAN_POINT ( 'NONE',  ( 9.972493632716181722, -3.822122635138222702, -9.279087650161129019 ) ) ;
#11867=CARTESIAN_POINT ( 'NONE',  ( 10.49412055961999890, -2.866949708568999888, -8.960719633954001395 ) ) ;
#11870=CARTESIAN_POINT ( 'NONE',  ( 10.41185831014999863, -2.101597930377999912, 7.856264717901999539 ) ) ;
#11873=ADVANCED_FACE ( 'NONE', ( #23937 ), #56440, .F. ) ;
#11882=CARTESIAN_POINT ( 'NONE',  ( 5.700000000378000031, -0.2999999996220999443, 3.150000004979999879 ) ) ;
#11883=AXIS2_PLACEMENT_3D ( 'NONE', #69044, #54336, #5749 ) ;
#11889=ORIENTED_EDGE ( 'NONE', *, *, #15959, .T. ) ;
#11909=DIRECTION ( 'NONE',  ( 1.000000000000000000, 0.000000000000000000, 0.000000000000000000 ) ) ;
#11935=CARTESIAN_POINT ( 'NONE',  ( 11.09999999999999964, -2.700000000000000178, -6.461133846875999787 ) ) ;
#11936=CARTESIAN_POINT ( 'NONE',  ( 10.88760685321000032, -5.634843745609000365, -7.088991614236999972 ) ) ;
#11937=CIRCLE ( 'NONE', #20873, 1.250000000000000000 ) ;
#11944=AXIS2_PLACEMENT_3D ( 'NONE', #11818, #68823, #69171 ) ;
#11957=ADVANCED_FACE ( 'NONE', ( #66919 ), #68093, .F. ) ;
#11958=CARTESIAN_POINT ( 'NONE',  ( 10.27571314244999989, -5.689440078020999714, -7.562019725378000601 ) ) ;
#11961=CARTESIAN_POINT ( 'NONE',  ( 10.85632228256448428, -2.901817188071407205, -5.114652766790887206 ) ) ;
#11967=CARTESIAN_POINT ( 'NONE',  ( 10.27152834814000215, -4.757994137332000051, 4.537574396426000689 ) ) ;
#11983=CARTESIAN_POINT ( 'NONE',  ( 10.11858840337999865, -3.393395892949000014, -5.921999462319999630 ) ) ;
#11985=CARTESIAN_POINT ( 'NONE',  ( 10.55101852148010266, -5.350099180695897516, -7.263329207706007651 ) ) ;
#11986=CIRCLE ( 'NONE', #64419, 2.149999999999999911 ) ;
#12001=CARTESIAN_POINT ( 'NONE',  ( 11.27109998545999936, -5.469594811916000054, 8.504700858852999090 ) ) ;
#12004=AXIS2_PLACEMENT_3D ( 'NONE', #27113, #47403, #37251 ) ;
#12005=CARTESIAN_POINT ( 'NONE',  ( 9.758146639703001668, -2.901368778958000050, 6.555068849476000103 ) ) ;
#12006=CARTESIAN_POINT ( 'NONE',  ( 9.710415594366155645, -5.733461026711495379, 7.739234121907153430 ) ) ;
#12019=CARTESIAN_POINT ( 'NONE',  ( -15.86200481174999943, -5.599999999999999645, -6.571291218949999902 ) ) ;
#12031=VECTOR ( 'NONE', #39209, 1000.000000000000114 ) ;
#12045=ORIENTED_EDGE ( 'NONE', *, *, #57521, .T. ) ;
#12046=CARTESIAN_POINT ( 'NONE',  ( 10.93728138146000006, -5.425439422033999648, 7.240583766112999697 ) ) ;
#12048=CARTESIAN_POINT ( 'NONE',  ( 8.960616452296999768, -2.899999999999999911, 6.279946362737000243 ) ) ;
#12050=AXIS2_PLACEMENT_3D ( 'NONE', #1111, #22424, #5313 ) ;
#12052=CARTESIAN_POINT ( 'NONE',  ( 10.95519194037999888, -3.860335380237000180, -6.147338954930000376 ) ) ;
#12070=CARTESIAN_POINT ( 'NONE',  ( 10.89874164595999950, -2.834836218627000193, 9.088455567997000273 ) ) ;
#12078=CARTESIAN_POINT ( 'NONE',  ( 7.309012197735174965, -3.319721303298527104, 6.319100263144195928 ) ) ;
#12080=EDGE_CURVE ( 'NONE', #42842, #5840, #41001, .T. ) ;
#12082=CARTESIAN_POINT ( 'NONE',  ( 8.090519353209000286, -5.342173944271999986, 8.432314172168000610 ) ) ;
#12085=CARTESIAN_POINT ( 'NONE',  ( 11.01817738136000102, -6.612169668047999771, 5.428883362029000459 ) ) ;
#12086=CARTESIAN_POINT ( 'NONE',  ( 9.258115045126002585, -5.097433850589000670, -6.601368032590999135 ) ) ;
#12087=EDGE_CURVE ( 'NONE', #49898, #2068, #38524, .T. ) ;
#12088=CYLINDRICAL_SURFACE ( 'NONE', #16828, 0.4999999999999998335 ) ;
#12091=CARTESIAN_POINT ( 'NONE',  ( 8.316694573732000606, -2.898380360490000029, 6.611503418275999522 ) ) ;
#12095=CARTESIAN_POINT ( 'NONE',  ( 9.059370559623998176, -4.192917962110999319, 5.525484568403999930 ) ) ;
#12102=EDGE_CURVE ( 'NONE', #28877, #29433, #46824, .T. ) ;
#12116=FACE_OUTER_BOUND ( 'NONE', #35621, .T. ) ;
#12126=ORIENTED_EDGE ( 'NONE', *, *, #21237, .F. ) ;
#12128=DIRECTION ( 'NONE',  ( -1.000000000000000000, 0.000000000000000000, 0.000000000000000000 ) ) ;
#12129=B_SPLINE_CURVE_WITH_KNOTS ( 'NONE', 3,
 ( #3566, #56030, #9158, #39609 ),
 .UNSPECIFIED., .F., .F.,
 ( 4, 4 ),
 ( 0.000000000000000000, 1.000000000000000000 ),
 .UNSPECIFIED. ) ;
#12153=ORIENTED_EDGE ( 'NONE', *, *, #10897, .F. ) ;
#12157=CARTESIAN_POINT ( 'NONE',  ( 10.26368921839999970, -4.794141574281000295, -8.804455889106000299 ) ) ;
#12159=CARTESIAN_POINT ( 'NONE',  ( 5.700000000172999570, 0.5292307618289999738, 2.083846155904000241 ) ) ;
#12170=B_SPLINE_CURVE_WITH_KNOTS ( 'NONE', 3,
 ( #10324, #15230, #26068, #68701, #20472, #36210, #15577 ),
 .UNSPECIFIED., .F., .F.,
 ( 4, 1, 1, 1, 4 ),
 ( 0.000000000000000000, 0.2500000039167279420, 0.5000000015353956995, 0.7499999991540633459, 1.000000000000000000 ),
 .UNSPECIFIED. ) ;
#12177=CARTESIAN_POINT ( 'NONE',  ( 8.592629440379999650, -3.856773448568000084, 5.521258396339000285 ) ) ;
#12178=CARTESIAN_POINT ( 'NONE',  ( 9.531727112333999941, -4.010297355695000121, -9.208122400763999238 ) ) ;
#12194=CARTESIAN_POINT ( 'NONE',  ( 10.07771285905000092, -4.622037501707999319, 5.671359981946999973 ) ) ;
#12199=CARTESIAN_POINT ( 'NONE',  ( 10.86460564679000029, -3.843601288168000174, -5.985268170611000471 ) ) ;
#12200=CARTESIAN_POINT ( 'NONE',  ( 7.732099726745981449, -5.601557586365069952, 8.181612574483722256 ) ) ;
#12201=CARTESIAN_POINT ( 'NONE',  ( 9.318721994369999706, -2.755032632138999737, 8.795122807847999269 ) ) ;
#12207=ORIENTED_EDGE ( 'NONE', *, *, #33620, .T. ) ;
#12217=B_SPLINE_CURVE_WITH_KNOTS ( 'NONE', 3,
 ( #35235, #46751, #24391, #68056, #24734, #46061 ),
 .UNSPECIFIED., .F., .F.,
 ( 4, 2, 4 ),
 ( 0.000000000000000000, 0.5000000000000004441, 1.000000000000000000 ),
 .UNSPECIFIED. ) ;
#12219=DIRECTION ( 'NONE',  ( -1.000000000000000000, 0.000000000000000000, 0.000000000000000000 ) ) ;
#12221=EDGE_LOOP ( 'NONE', ( #46801, #27514, #18755, #4206, #8894, #33158, #45747, #49226, #766, #19830 ) ) ;
#12223=CARTESIAN_POINT ( 'NONE',  ( 10.15102996164048932, -2.740893273674518849, -6.282207469075709483 ) ) ;
#12225=CARTESIAN_POINT ( 'NONE',  ( 10.15335805961999860, -3.144986649008000068, -5.860958514434000399 ) ) ;
#12229=CARTESIAN_POINT ( 'NONE',  ( 11.02445830383999947, -3.404091099119999519, 5.822494319281999786 ) ) ;
#12233=CARTESIAN_POINT ( 'NONE',  ( 0.000000000000000000, -5.100000000000000533, 7.500000000000000000 ) ) ;
#12235=EDGE_CURVE ( 'NONE', #33712, #39743, #13533, .T. ) ;
#12248=ORIENTED_EDGE ( 'NONE', *, *, #30483, .F. ) ;
#12266=AXIS2_PLACEMENT_3D ( 'NONE', #58631, #5832, #27170 ) ;
#12293=CARTESIAN_POINT ( 'NONE',  ( 10.59956814679000026, -4.438148200474000937, -8.958389257466000899 ) ) ;
#12298=CARTESIAN_POINT ( 'NONE',  ( 11.09999999999999964, -5.299316147296000423, 5.124965750789000296 ) ) ;
#12305=CARTESIAN_POINT ( 'NONE',  ( 9.113217775048997993, -8.654438058834999836, 6.112263052845000821 ) ) ;
#12306=CYLINDRICAL_SURFACE ( 'NONE', #56611, 1.350000000000000089 ) ;
#12310=CARTESIAN_POINT ( 'NONE',  ( 10.95551720753999980, -4.744041807741999683, -9.198129812222999746 ) ) ;
#12320=CARTESIAN_POINT ( 'NONE',  ( 10.70976172572000173, -5.125515269697999976, 5.002993350055000121 ) ) ;
#12321=CARTESIAN_POINT ( 'NONE',  ( 10.61517041231343761, -2.962049961264340947, 5.046074788812947354 ) ) ;
#12324=CARTESIAN_POINT ( 'NONE',  ( 10.87148543990999983, -5.567571293949000300, 7.772413914480000408 ) ) ;
#12328=ORIENTED_EDGE ( 'NONE', *, *, #45011, .F. ) ;
#12335=DIRECTION ( 'NONE',  ( 1.000000000000000000, 0.000000000000000000, 0.000000000000000000 ) ) ;
#12336=CARTESIAN_POINT ( 'NONE',  ( 10.00074484908000194, -2.373896846742000299, -7.962434077545999855 ) ) ;
#12338=CARTESIAN_POINT ( 'NONE',  ( 11.08757144985999865, -2.712428550139000194, 6.571291218949999902 ) ) ;
#12340=CARTESIAN_POINT ( 'NONE',  ( 9.746744136172999617, -5.062748727288000516, -8.618689820632001286 ) ) ;
#12348=VERTEX_POINT ( 'NONE', #3551 ) ;
#12351=CARTESIAN_POINT ( 'NONE',  ( 10.21608469020999976, -5.961703525007000515, 7.319668113368000384 ) ) ;
#12354=CARTESIAN_POINT ( 'NONE',  ( 9.848732933287999813, -2.769734897491000325, 6.441850735262000249 ) ) ;
#12356=CARTESIAN_POINT ( 'NONE',  ( 11.10000000009000054, -5.300000000088999741, -6.571291220400000022 ) ) ;
#12360=CONICAL_SURFACE ( 'NONE', #51439, 0.8999999994071996579, 0.7853981633972997312 ) ;
#12372=EDGE_LOOP ( 'NONE', ( #1647, #54672, #440, #55697 ) ) ;
#12385=CARTESIAN_POINT ( 'NONE',  ( 9.187745559622999991, -5.964711531933999389, 7.776478361891000723 ) ) ;
#12387=CARTESIAN_POINT ( 'NONE',  ( 11.10000000000000142, -2.264799782219416802, -7.479379319469428467 ) ) ;
#12389=CARTESIAN_POINT ( 'NONE',  ( 9.258050732556000639, -4.895927245463000510, -6.008721945297999412 ) ) ;
#12391=CARTESIAN_POINT ( 'NONE',  ( 10.94166666666863996, -5.229667600279077178, 8.191470186739737258 ) ) ;
#12394=ADVANCED_FACE ( 'NONE', ( #25577 ), #67523, .F. ) ;
#12401=LINE ( 'NONE', #34079, #35405 ) ;
#12402=ORIENTED_EDGE ( 'NONE', *, *, #28727, .F. ) ;
#12410=CARTESIAN_POINT ( 'NONE',  ( 6.869678056658000465, -9.249704301540999651, -5.114242507410000194 ) ) ;
#12419=CARTESIAN_POINT ( 'NONE',  ( 9.347248564704999652, -4.028326926800000152, 9.469437404464001062 ) ) ;
#12428=CARTESIAN_POINT ( 'NONE',  ( 10.56492304196000021, -4.212244324161999565, 8.933470634735002136 ) ) ;
#12430=CARTESIAN_POINT ( 'NONE',  ( 7.614808059621999803, -3.326257819185999942, 8.794522506294001118 ) ) ;
#12433=CARTESIAN_POINT ( 'NONE',  ( 11.07204542438999972, -5.775934056910999814, 5.099638290457999545 ) ) ;
#12440=EDGE_LOOP ( 'NONE', ( #67367, #40747, #66301, #61940, #60768, #24333 ) ) ;
#12450=ORIENTED_EDGE ( 'NONE', *, *, #25572, .T. ) ;
#12452=CARTESIAN_POINT ( 'NONE',  ( 7.805869834195655166, -3.184795896352067501, 6.408392962140504245 ) ) ;
#12453=VECTOR ( 'NONE', #51529, 1000.000000000000114 ) ;
#12460=CARTESIAN_POINT ( 'NONE',  ( 8.586687454835056243, -4.265569429095399379, 5.778312903272157186 ) ) ;
#12464=CARTESIAN_POINT ( 'NONE',  ( 9.792562654643999664, -3.463427761954999795, 6.184385360914999907 ) ) ;
#12470=VERTEX_POINT ( 'NONE', #61946 ) ;
#12472=DIRECTION ( 'NONE',  ( 0.000000000000000000, 1.000000000000000000, 0.000000000000000000 ) ) ;
#12474=CARTESIAN_POINT ( 'NONE',  ( 8.817462135714999150, -5.100000000000000533, 6.571291218949999902 ) ) ;
#12475=CARTESIAN_POINT ( 'NONE',  ( 9.179055905797000037, -2.899999999999999911, 6.571291218949999902 ) ) ;
#12483=ORIENTED_EDGE ( 'NONE', *, *, #18706, .F. ) ;
#12494=B_SPLINE_CURVE_WITH_KNOTS ( 'NONE', 3,
 ( #15543, #26380, #69016, #38146, #56656, #2479 ),
 .UNSPECIFIED., .F., .F.,
 ( 4, 1, 1, 4 ),
 ( 0.000000000000000000, 0.3333333333333000081, 0.6666666666667000474, 1.000000000000000000 ),
 .UNSPECIFIED. ) ;
#12500=CARTESIAN_POINT ( 'NONE',  ( 10.01597818573999987, -4.792673671522000411, -6.390249203106999509 ) ) ;
#12508=B_SPLINE_CURVE_WITH_KNOTS ( 'NONE', 3,
 ( #13164, #34492, #7906, #18745 ),
 .UNSPECIFIED., .F., .F.,
 ( 4, 4 ),
 ( 0.000000000000000000, 1.000000000000000000 ),
 .UNSPECIFIED. ) ;
#12510=CARTESIAN_POINT ( 'NONE',  ( 10.36409408021999923, -3.399999909169000301, -4.954046131279000065 ) ) ;
#12511=DIRECTION ( 'NONE',  ( 1.000000000000000000, 0.000000000000000000, 0.000000000000000000 ) ) ;
#12520=ORIENTED_EDGE ( 'NONE', *, *, #8853, .F. ) ;
#12521=CARTESIAN_POINT ( 'NONE',  ( 7.437254440376999121, -2.216884807317999861, 8.370075800106999253 ) ) ;
#12522=CARTESIAN_POINT ( 'NONE',  ( 10.15291672334000062, -4.949038487346999915, -8.498994087616001281 ) ) ;
#12527=B_SPLINE_CURVE_WITH_KNOTS ( 'NONE', 3,
 ( #17463, #3357, #40419, #3015, #32853, #27957, #18766 ),
 .UNSPECIFIED., .F., .F.,
 ( 4, 1, 1, 1, 4 ),
 ( 0.000000000000000000, 0.2500000143192999680, 0.5000000056314000130, 0.7499999969435999780, 1.000000000000000000 ),
 .UNSPECIFIED. ) ;
#12533=ADVANCED_FACE ( 'NONE', ( #29000 ), #38576, .T. ) ;
#12539=CARTESIAN_POINT ( 'NONE',  ( 9.576494682405000347, -4.593972507100000158, 5.662052676321000177 ) ) ;
#12543=CARTESIAN_POINT ( 'NONE',  ( 10.84160444037999937, -2.641264320582999758, -7.444904971031999885 ) ) ;
#12544=CARTESIAN_POINT ( 'NONE',  ( 8.058954703304616274, -3.652055520346594975, 5.795450222806093343 ) ) ;
#12545=CARTESIAN_POINT ( 'NONE',  ( 10.68403590588000007, -5.436611040123999317, 8.578433628717998971 ) ) ;
#12546=CARTESIAN_POINT ( 'NONE',  ( 10.10331918378244431, -3.090221196180537699, 8.647993508352264769 ) ) ;
#12564=ORIENTED_EDGE ( 'NONE', *, *, #47132, .F. ) ;
#12565=CARTESIAN_POINT ( 'NONE',  ( 8.047379440378000126, -4.468370631666999770, 8.882152684713000568 ) ) ;
#12574=CARTESIAN_POINT ( 'NONE',  ( 8.142152878612618494, -3.293758513149224854, 8.705677052449603437 ) ) ;
#12582=FACE_OUTER_BOUND ( 'NONE', #42536, .T. ) ;
#12608=CARTESIAN_POINT ( 'NONE',  ( 8.817629440380001071, -3.894643656844000379, 6.044452984962999764 ) ) ;
#12612=ORIENTED_EDGE ( 'NONE', *, *, #40874, .T. ) ;
#12619=DIRECTION ( 'NONE',  ( 0.000000000000000000, -0.8707944170444857912, 0.4916473159126918957 ) ) ;
#12622=DIRECTION ( 'NONE',  ( -1.000000000000000000, 0.000000000000000000, 0.000000000000000000 ) ) ;
#12626=LINE ( 'NONE', #60863, #22978 ) ;
#12628=CARTESIAN_POINT ( 'NONE',  ( 7.424682295424686274, -2.345875091448395455, 8.038402344753549755 ) ) ;
#12637=CARTESIAN_POINT ( 'NONE',  ( 9.406851002546000373, -2.832432432432000269, -6.822293592207000934 ) ) ;
#12657=CARTESIAN_POINT ( 'NONE',  ( 11.06133683778999988, -2.503914237677999921, -6.712780725818999983 ) ) ;
#12663=DIRECTION ( 'NONE',  ( 1.000000000000000000, -1.157371756828000031E-14, -5.786858784138000079E-14 ) ) ;
#12664=CARTESIAN_POINT ( 'NONE',  ( 10.27635097765000083, -4.738769859112000660, 4.693832200104000485 ) ) ;
#12667=PLANE ( 'NONE',  #46233 ) ;
#12670=CARTESIAN_POINT ( 'NONE',  ( 9.889844610056000462, -4.052276314598000084, 9.260527932809999641 ) ) ;
#12684=DIRECTION ( 'NONE',  ( 1.000000000000000000, 0.000000000000000000, 0.000000000000000000 ) ) ;
#12686=CARTESIAN_POINT ( 'NONE',  ( 9.526735624254000001, -3.423478821957000040, -6.068694811299999436 ) ) ;
#12692=CARTESIAN_POINT ( 'NONE',  ( 10.57189201149000191, -2.801299163661999714, 4.692232677100000693 ) ) ;
#12695=AXIS2_PLACEMENT_3D ( 'NONE', #51443, #45860, #34694 ) ;
#12697=CARTESIAN_POINT ( 'NONE',  ( 9.476374593785998002, -5.098398394707999159, 6.305533045879999854 ) ) ;
#12701=CARTESIAN_POINT ( 'NONE',  ( 9.290195424034999760, -2.377814350880000038, 7.540992175424999999 ) ) ;
#12712=CARTESIAN_POINT ( 'NONE',  ( 9.258104461123007667, -2.902565898239000131, -6.601372212749001100 ) ) ;
#12717=CARTESIAN_POINT ( 'NONE',  ( 8.576923877145999242, -3.399999999999999911, 5.924121105096999962 ) ) ;
#12718=CARTESIAN_POINT ( 'NONE',  ( 9.524152735436000938, -4.911674715448000050, -6.466751564808000730 ) ) ;
#12721=CARTESIAN_POINT ( 'NONE',  ( 8.960616452296999768, -2.899999999999999911, 6.279946362737000243 ) ) ;
#12726=ADVANCED_FACE ( 'NONE', ( #21722 ), #62, .F. ) ;
#12735=CARTESIAN_POINT ( 'NONE',  ( 9.316120559621998254, -3.677416446733000388, 9.250734868033999803 ) ) ;
#12737=CARTESIAN_POINT ( 'NONE',  ( 11.10000000000000142, -2.373997543953228373, -7.952634597122376192 ) ) ;
#12742=EDGE_LOOP ( 'NONE', ( #48617, #41212, #26507, #46648 ) ) ;
#12743=CARTESIAN_POINT ( 'NONE',  ( 9.447848023450999833, -5.447470167531999863, 7.431328114251999573 ) ) ;
#12744=DIRECTION ( 'NONE',  ( 0.000000000000000000, -0.1333333333333049375, -0.9910712498212375099 ) ) ;
#12758=CARTESIAN_POINT ( 'NONE',  ( 6.789185465859000068, -9.291930834867999422, -5.322879461504999909 ) ) ;
#12767=CARTESIAN_POINT ( 'NONE',  ( 9.566960887370999700, -5.215923019114000247, 6.177729435798999802 ) ) ;
#12778=CARTESIAN_POINT ( 'NONE',  ( 8.218894353209000414, -3.011617647609999615, 8.801438026873999121 ) ) ;
#12781=CARTESIAN_POINT ( 'NONE',  ( 11.12438586031000121, -6.497919266103000524, 5.557820251765999586 ) ) ;
#12785=CARTESIAN_POINT ( 'NONE',  ( 10.42374681322000107, -3.188261102799000213, -5.025588318470999738 ) ) ;
#12787=B_SPLINE_SURFACE_WITH_KNOTS ( 'NONE', 3, 3, ( 
 ( #4411, #25750, #47079, #61772, #18795, #3721, #19123, #25058, #35562, #61436, #13556, #29644, #13893, #8637, #24720, #67693, #46044, #56878, #37270, #208, #47773, #42518, #20501, #32719, #21869, #48452, #32382, #57909, #36935, #20848, #43206, #15260, #36583, #10692, #47421 ),
 ( #10007, #31345, #54031, #53696, #58248, #4754, #16284, #16629, #27472, #10352, #5106, #21528, #68729, #37955, #15603, #69082, #6133, #64509, #42861, #58592, #63827, #21187, #26443, #5789, #15941, #32039, #52658, #59276, #53354, #11047, #5457, #31688, #26792, #27132, #64170 ),
 ( #53009, #11378, #48108, #42181, #68380, #41826, #63134, #26096, #37609, #58940, #560, #63484, #22219, #48797, #66247, #6831, #12082, #16967, #12778, #39004, #906, #28163, #38649, #7182, #22906, #7873, #55426, #1247, #7517, #28872, #59972, #13130, #28519, #49830, #18369 ),
 ( #17679, #33413, #39691, #61012, #44606, #50180, #22561, #34458, #60321, #11722, #12430, #44260, #2283, #55076, #33064, #33761, #17323, #43903, #55771, #1943, #23262, #23601, #65899, #43555, #18027, #64856, #39342, #60663, #44942, #54730, #49479, #34107, #38298, #59628, #54380 ) ),
 .UNSPECIFIED., .F., .F., .F.,
 ( 4, 4 ),
 ( 4, 1, 1, 1, 1, 1, 1, 1, 1, 1, 1, 1, 1, 1, 1, 1, 1, 1, 1, 1, 1, 1, 1, 1, 1, 1, 1, 1, 1, 1, 1, 1, 4 ),
 ( -0.1039086239011999951, 1.103908623900999864 ),
 ( -0.02000000000000000042, 0.01250000000000000069, 0.04499999999999999833, 0.07749999999999999944, 0.1100000000000000006, 0.1424999999999999878, 0.1749999999999999889, 0.2074999999999999900, 0.2399999999999999911, 0.2725000000000000200, 0.3049999999999999933, 0.3375000000000000222, 0.3699999999999999956, 0.4025000000000000244, 0.4349999999999999978, 0.4675000000000000266, 0.5000000000000000000, 0.5324999999999999734, 0.5649999999999999467, 0.5975000000000000311, 0.6300000000000000044, 0.6624999999999999778, 0.6949999999999999512, 0.7275000000000000355, 0.7600000000000000089, 0.7924999999999999822, 0.8249999999999999556, 0.8575000000000000400, 0.8900000000000000133, 0.9224999999999999867, 0.9549999999999999600, 0.9875000000000000444, 1.020000000000000018 ),
 .UNSPECIFIED. ) ;
#12814=CARTESIAN_POINT ( 'NONE',  ( 11.03776249210999971, -8.050323671732000363, -6.914613055281999543 ) ) ;
#12816=CARTESIAN_POINT ( 'NONE',  ( 11.09999999999999964, -4.000000000000000000, 7.500000000000000000 ) ) ;
#12819=CARTESIAN_POINT ( 'NONE',  ( 9.489492991957288126, -4.926916480655023634, 8.481281896443434221 ) ) ;
#12821=AXIS2_PLACEMENT_3D ( 'NONE', #36818, #5332, #26326 ) ;
#12835=CARTESIAN_POINT ( 'NONE',  ( 10.70259541447426344, -2.712334124290769921, 7.031803886929559155 ) ) ;
#12845=ORIENTED_EDGE ( 'NONE', *, *, #13767, .T. ) ;
#12849=CARTESIAN_POINT ( 'NONE',  ( 10.90421209872000041, -3.863781031729999871, -9.185081053980001187 ) ) ;
#12860=CYLINDRICAL_SURFACE ( 'NONE', #10535, 0.4999999999999998335 ) ;
#12870=ORIENTED_EDGE ( 'NONE', *, *, #16275, .F. ) ;
#12871=CARTESIAN_POINT ( 'NONE',  ( 8.143316940379001778, -5.061720701958000390, 5.824087910811999613 ) ) ;
#12883=ORIENTED_EDGE ( 'NONE', *, *, #8830, .F. ) ;
#12887=CARTESIAN_POINT ( 'NONE',  ( 10.72520823780999955, -5.521647200017000934, 6.612992938078999572 ) ) ;
#12888=CARTESIAN_POINT ( 'NONE',  ( 8.513433059625000965, -5.040796345420999636, 8.522966281393001609 ) ) ;
#12892=EDGE_CURVE ( 'NONE', #12470, #60343, #44112, .T. ) ;
#12893=CARTESIAN_POINT ( 'NONE',  ( 7.944408677273556485, -2.261289390559563905, 7.612513792833588866 ) ) ;
#12894=CARTESIAN_POINT ( 'NONE',  ( 10.65550933554000146, -4.237674644795000667, 9.105223721671999115 ) ) ;
#12897=ORIENTED_EDGE ( 'NONE', *, *, #52393, .F. ) ;
#12904=CARTESIAN_POINT ( 'NONE',  ( 9.839739029020998728, -5.130141620686999637, -6.219151643305999677 ) ) ;
#12914=CARTESIAN_POINT ( 'NONE',  ( 8.508081853209001011, -2.202816532622999812, 7.706987678916999762 ) ) ;
#12924=CARTESIAN_POINT ( 'NONE',  ( 8.183771503764621258, -2.796787595787157521, 8.203896902613195152 ) ) ;
#12933=DIRECTION ( 'NONE',  ( 1.000000000000000000, 0.000000000000000000, 0.000000000000000000 ) ) ;
#12943=ORIENTED_EDGE ( 'NONE', *, *, #34508, .T. ) ;
#12954=LINE ( 'NONE', #46138, #14345 ) ;
#12955=VERTEX_POINT ( 'NONE', #54587 ) ;
#12962=CARTESIAN_POINT ( 'NONE',  ( 8.368316940379001423, -4.780993534312999671, 6.267212032957000467 ) ) ;
#12973=CARTESIAN_POINT ( 'NONE',  ( 11.09999999999999964, -4.000000000000000000, -7.500000000000000000 ) ) ;
#12977=CARTESIAN_POINT ( 'NONE',  ( 9.411512147430608266, -5.333029039908475433, 7.282975621311138070 ) ) ;
#12980=DIRECTION ( 'NONE',  ( 1.000000000000000000, 0.000000000000000000, -1.776356839484000040E-14 ) ) ;
#12982=CARTESIAN_POINT ( 'NONE',  ( 7.430335179696497150, -2.310327096630513832, 7.914026420381109261 ) ) ;
#12992=CARTESIAN_POINT ( 'NONE',  ( 10.42511694037999881, -3.371058793856000158, -6.294333763729999198 ) ) ;
#13003=CARTESIAN_POINT ( 'NONE',  ( 8.971881080173746525, -5.348857519615915379, 7.441217429712126297 ) ) ;
#13012=CARTESIAN_POINT ( 'NONE',  ( 10.30297040315999979, -4.081263557776000361, -9.025012210052000938 ) ) ;
#13017=CARTESIAN_POINT ( 'NONE',  ( 11.01870451217999936, -2.731005928090000090, -4.994859145087000130 ) ) ;
#13018=CYLINDRICAL_SURFACE ( 'NONE', #7965, 1.350000000000000089 ) ;
#13019=CARTESIAN_POINT ( 'NONE',  ( 10.42440867506999957, -5.011664035303000198, 4.759074316248999459 ) ) ;
#13020=DIRECTION ( 'NONE',  ( 0.000000000000000000, -1.000000000000000000, 0.000000000000000000 ) ) ;
#13021=CARTESIAN_POINT ( 'NONE',  ( 11.09999999999999964, -4.000000000000000000, 7.500000000000000000 ) ) ;
#13025=CARTESIAN_POINT ( 'NONE',  ( 10.11260824411999870, -3.359889198679999911, 5.859131457670000209 ) ) ;
#13033=FACE_OUTER_BOUND ( 'NONE', #40396, .T. ) ;
#13039=CARTESIAN_POINT ( 'NONE',  ( 9.218723707566001124, -5.383415012847999392, -8.183490493635000362 ) ) ;
#13054=CARTESIAN_POINT ( 'NONE',  ( 10.93227479887999998, -2.539880901735999785, 6.453614191797999666 ) ) ;
#13057=CARTESIAN_POINT ( 'NONE',  ( 9.013429960698999821, -4.933961117404000341, 8.417889755737999025 ) ) ;
#13059=EDGE_LOOP ( 'NONE', ( #57594, #61899, #33203, #50772 ) ) ;
#13064=CARTESIAN_POINT ( 'NONE',  ( 8.525643369680000916, -2.918411554970002708, -6.570687780412999501 ) ) ;
#13069=CARTESIAN_POINT ( 'NONE',  ( 9.793328727373999953, -5.651611919872999934, -7.935921913274999184 ) ) ;
#13089=CARTESIAN_POINT ( 'NONE',  ( 11.09999999999999964, -2.646159083949000124, 6.745271721726000536 ) ) ;
#13091=CARTESIAN_POINT ( 'NONE',  ( 10.00638553269999953, -5.119272496996000399, 8.420388242270998802 ) ) ;
#13098=B_SPLINE_CURVE_WITH_KNOTS ( 'NONE', 3,
 ( #11395, #32734, #15956, #57927 ),
 .UNSPECIFIED., .F., .F.,
 ( 4, 4 ),
 ( 0.000000000000000000, 1.000000000000000000 ),
 .UNSPECIFIED. ) ;
#13105=EDGE_CURVE ( 'NONE', #60343, #29839, #52436, .T. ) ;
#13111=CARTESIAN_POINT ( 'NONE',  ( 9.354368786244091183, -3.362065969394026688, 9.118206140364792489 ) ) ;
#13113=CARTESIAN_POINT ( 'NONE',  ( 8.331682137624000006, -5.101289325373999262, 6.607176193198000647 ) ) ;
#13115=CARTESIAN_POINT ( 'NONE',  ( 11.13500449003999826, -5.334503170127000260, -5.174025948961000765 ) ) ;
#13119=CARTESIAN_POINT ( 'NONE',  ( 9.877259503622999759, -2.207992199716000137, 7.624813542847999059 ) ) ;
#13123=ORIENTED_EDGE ( 'NONE', *, *, #45151, .F. ) ;
#13126=CARTESIAN_POINT ( 'NONE',  ( 7.307500000000000107, -0.2999999999999999889, 3.149999999999999911 ) ) ;
#13128=CARTESIAN_POINT ( 'NONE',  ( 9.143006881379495354, -5.327771165987038593, 6.363180085552491150 ) ) ;
#13130=CARTESIAN_POINT ( 'NONE',  ( 9.053331853208000268, -5.618388245857000030, 7.727743016644000207 ) ) ;
#13136=CARTESIAN_POINT ( 'NONE',  ( 10.98768538770000092, -2.700669876604000041, 4.945210823433001224 ) ) ;
#13141=ORIENTED_EDGE ( 'NONE', *, *, #10897, .T. ) ;
#13146=CARTESIAN_POINT ( 'NONE',  ( 7.954655249370001791, -5.133340916889001626, 6.761736834907998706 ) ) ;
#13155=CARTESIAN_POINT ( 'NONE',  ( 7.810165831303219619, -3.098200876999478215, 6.455848190766955597 ) ) ;
#13157=CARTESIAN_POINT ( 'NONE',  ( 11.01356641589999974, -2.786433584103999994, 6.253463831328000211 ) ) ;
#13158=VECTOR ( 'NONE', #64865, 1000.000000000000114 ) ;
#13164=CARTESIAN_POINT ( 'NONE',  ( 9.472537864290000442, -2.899999999999999911, -6.571291218949999902 ) ) ;
#13172=CARTESIAN_POINT ( 'NONE',  ( 8.277730646792999636, -4.874569256861000177, 6.119503992241999590 ) ) ;
#13174=EDGE_LOOP ( 'NONE', ( #14217, #32445, #61697, #2127, #52827, #24405 ) ) ;
#13175=CARTESIAN_POINT ( 'NONE',  ( 9.091609899095999481, -8.664388034093999380, 6.180722816477000059 ) ) ;
#13179=CARTESIAN_POINT ( 'NONE',  ( 9.883148997457000817, -5.167567567567999731, 6.822293592207000934 ) ) ;
#13185=CARTESIAN_POINT ( 'NONE',  ( 9.753242276648833808, -2.714773723612734724, 7.027402982326762526 ) ) ;
#13187=PRODUCT_DEFINITION_SHAPE ( 'NONE', 'NONE',  #16698 ) ;
#13189=CARTESIAN_POINT ( 'NONE',  ( 10.95677425385773951, -2.827156737707505751, -6.689562958348049371 ) ) ;
#13204=CARTESIAN_POINT ( 'NONE',  ( 9.976697000975999430, -4.172225768856000272, -6.147144998063999388 ) ) ;
#13209=CIRCLE ( 'NONE', #5395, 1.350000000000000533 ) ;
#13212=CARTESIAN_POINT ( 'NONE',  ( 10.61503919148196218, -5.349978903665073560, -7.499997722305344006 ) ) ;
#13223=LINE ( 'NONE', #34549, #64519 ) ;
#13225=VERTEX_POINT ( 'NONE', #44721 ) ;
#13226=CARTESIAN_POINT ( 'NONE',  ( 8.079129440378000737, -3.524751762020000179, 5.573845465339999805 ) ) ;
#13231=B_SPLINE_CURVE_WITH_KNOTS ( 'NONE', 3,
 ( #48056, #849, #64117, #10643 ),
 .UNSPECIFIED., .F., .F.,
 ( 4, 4 ),
 ( 0.000000000000000000, 1.000000000000000000 ),
 .UNSPECIFIED. ) ;
#13241=CARTESIAN_POINT ( 'NONE',  ( 10.05691733561000056, -2.453480799114999833, 6.657106310117000270 ) ) ;
#13244=DIRECTION ( 'NONE',  ( 0.8843050097021329936, 0.1786785991674020024, -0.4313682974156600181 ) ) ;
#13245=CARTESIAN_POINT ( 'NONE',  ( 11.33381694038000020, -2.642393655627000015, -7.577897390831000557 ) ) ;
#13246=CARTESIAN_POINT ( 'NONE',  ( 7.933496154964543301, -2.297183234189244860, 7.856070056283313008 ) ) ;
#13247=CARTESIAN_POINT ( 'NONE',  ( 9.228135700785001561, -2.875364528161000077, 8.669943154892999715 ) ) ;
#13253=ORIENTED_EDGE ( 'NONE', *, *, #42791, .T. ) ;
#13256=CARTESIAN_POINT ( 'NONE',  ( 9.930325322607000516, -5.020908168068000776, -6.342951604057000203 ) ) ;
#13268=CARTESIAN_POINT ( 'NONE',  ( 7.764230646791999924, -4.628942671846000501, 5.991663889842000046 ) ) ;
#13273=CARTESIAN_POINT ( 'NONE',  ( 9.888320559623000605, -5.105186397454999359, -8.895598708036001057 ) ) ;
#13286=AXIS2_PLACEMENT_3D ( 'NONE', #48520, #43276, #6896 ) ;
#13288=DIRECTION ( 'NONE',  ( 0.7071067306621966475, 0.09464344911259944815, 0.7007443820625967046 ) ) ;
#13313=CARTESIAN_POINT ( 'NONE',  ( 10.76375265279853366, -5.207958528999011349, 8.762692967157324375 ) ) ;
#13314=CARTESIAN_POINT ( 'NONE',  ( 8.149355646792999508, -2.583664704444999849, 6.684748541034000624 ) ) ;
#13321=CARTESIAN_POINT ( 'NONE',  ( 11.09999999999999964, -2.700469802787999640, -5.124965750789000296 ) ) ;
#13331=CARTESIAN_POINT ( 'NONE',  ( 7.421943355951564847, -2.366001551502044720, 8.097493604183329197 ) ) ;
#13336=CARTESIAN_POINT ( 'NONE',  ( 27.64127793187000037, -3.399999999999999911, -4.505338571134999803 ) ) ;
#13339=ADVANCED_FACE ( 'NONE', ( #51326 ), #53064, .F. ) ;
#13340=CARTESIAN_POINT ( 'NONE',  ( 10.38314899745999931, -5.167567567567999731, 6.822293592207000934 ) ) ;
#13341=CARTESIAN_POINT ( 'NONE',  ( 11.10664194037999941, -5.324199331986000594, -7.809344861333999965 ) ) ;
#13357=CARTESIAN_POINT ( 'NONE',  ( 10.48164908029000131, -4.022873587130999518, 9.090901241422999490 ) ) ;
#13361=EDGE_CURVE ( 'NONE', #852, #39266, #7563, .T. ) ;
#13365=CARTESIAN_POINT ( 'NONE',  ( 10.38937479142535913, -8.258793008140132841, 6.886170040595600561 ) ) ;
#13368=B_SPLINE_CURVE_WITH_KNOTS ( 'NONE', 3,
 ( #5551, #67801, #58692, #57314, #26201, #46496, #41246, #58014, #9414, #31791, #47180 ),
 .UNSPECIFIED., .F., .F.,
 ( 4, 1, 1, 1, 1, 1, 1, 1, 4 ),
 ( 0.000000000000000000, 0.06984075817144648479, 0.2122522371145511844, 0.3546637160571506908, 0.4970751950002550990, 0.6394866739433597846, 0.7818981528859593189, 0.9243096318290640045, 1.000000000000000000 ),
 .UNSPECIFIED. ) ;
#13372=CARTESIAN_POINT ( 'NONE',  ( 11.14993998249000029, -2.627133311863999676, 6.696092388640000337 ) ) ;
#13378=CYLINDRICAL_SURFACE ( 'NONE', #10304, 0.5000000000000002220 ) ;
#13383=EDGE_CURVE ( 'NONE', #65964, #2231, #4444, .T. ) ;
#13384=CYLINDRICAL_SURFACE ( 'NONE', #23530, 0.4999999999999998335 ) ;
#13389=CARTESIAN_POINT ( 'NONE',  ( 9.617321917839001699, -3.361793157411000266, -5.915550373431999631 ) ) ;
#13396=CARTESIAN_POINT ( 'NONE',  ( 10.26390484475999898, -3.364655826309999931, 4.688340142401999699 ) ) ;
#13399=CARTESIAN_POINT ( 'NONE',  ( 9.860095611463300713, -4.592594002674506015, -8.996708106635217916 ) ) ;
#13400=CARTESIAN_POINT ( 'NONE',  ( 10.37373728961999930, -2.215269876326000364, 7.703982265807999497 ) ) ;
#13409=B_SPLINE_CURVE_WITH_KNOTS ( 'NONE', 3,
 ( #30789, #61914, #29782, #2839 ),
 .UNSPECIFIED., .F., .F.,
 ( 4, 4 ),
 ( 0.000000000000000000, 1.000000000000000000 ),
 .UNSPECIFIED. ) ;
#13414=B_SPLINE_CURVE_WITH_KNOTS ( 'NONE', 3,
 ( #28899, #13500, #39718, #18050 ),
 .UNSPECIFIED., .F., .F.,
 ( 4, 4 ),
 ( 0.000000000000000000, 1.000000000000000000 ),
 .UNSPECIFIED. ) ;
#13418=CARTESIAN_POINT ( 'NONE',  ( 9.971918425727000823, -4.365624317997999881, -9.242254741729000855 ) ) ;
#13429=ORIENTED_EDGE ( 'NONE', *, *, #18454, .T. ) ;
#13455=CARTESIAN_POINT ( 'NONE',  ( 9.402626378948871988, -2.553903598434096089, 8.467682852844752972 ) ) ;
#13462=CARTESIAN_POINT ( 'NONE',  ( 10.24961784311999935, -4.184221496660999406, 9.286877953065999947 ) ) ;
#13478=CARTESIAN_POINT ( 'NONE',  ( 11.07206039417999932, -6.376288328743000555, 5.346922539581000500 ) ) ;
#13481=DIRECTION ( 'NONE',  ( 0.000000000000000000, -0.8648648648648717963, -0.5020047465136829867 ) ) ;
#13487=CARTESIAN_POINT ( 'NONE',  ( 11.03766149047999967, -5.246943569709999977, -5.025196799498999667 ) ) ;
#13500=CARTESIAN_POINT ( 'NONE',  ( 10.94911764820105482, -2.860072064609847864, 5.104013334854830219 ) ) ;
#13512=CARTESIAN_POINT ( 'NONE',  ( 9.388626433405999450, -4.079401915682999480, 9.259353168384000909 ) ) ;
#13513=ORIENTED_EDGE ( 'NONE', *, *, #43279, .T. ) ;
#13515=CARTESIAN_POINT ( 'NONE',  ( 7.919004440377000797, -5.361050935357000391, 6.973449182446000094 ) ) ;
#13525=CARTESIAN_POINT ( 'NONE',  ( 10.58844302970999962, -3.754658547780000521, 5.545362468768000319 ) ) ;
#13526=B_SPLINE_CURVE_WITH_KNOTS ( 'NONE', 3,
 ( #49798, #44906, #2584, #38968, #12391, #7483, #6791, #65516, #49100, #18674, #17286, #29175, #28836, #17988, #23226, #55041, #28480, #13089 ),
 .UNSPECIFIED., .F., .F.,
 ( 4, 2, 2, 2, 2, 2, 2, 2, 4 ),
 ( 0.000000000000000000, 0.1250000000000001110, 0.2500000000000002220, 0.3750000000000003331, 0.5000000000000004441, 0.6250000000000003331, 0.7500000000000002220, 0.8750000000000001110, 1.000000000000000000 ),
 .UNSPECIFIED. ) ;
#13533=B_SPLINE_CURVE_WITH_KNOTS ( 'NONE', 3,
 ( #9217, #31251, #14819, #19722, #35466, #57116, #30555, #41045, #9562, #52215, #10255, #4657, #14138, #25996, #4316, #36480, #15160, #9913 ),
 .UNSPECIFIED., .F., .F.,
 ( 4, 2, 2, 2, 2, 2, 2, 2, 4 ),
 ( 0.1253528645472067604, 0.2189972814376893728, 0.3126416983281720130, 0.4062861152186546532, 0.4999305321091372933, 0.5935749489996199335, 0.6872193658901024627, 0.7808637827805851028, 0.8745081996710677430 ),
 .UNSPECIFIED. ) ;
#13545=CARTESIAN_POINT ( 'NONE',  ( 10.95551720753999980, -4.744041807741999683, -9.198129812222999746 ) ) ;
#13546=EDGE_CURVE ( 'NONE', #57286, #63228, #1283, .T. ) ;
#13549=B_SPLINE_CURVE_WITH_KNOTS ( 'NONE', 3,
 ( #60405, #65979, #54811, #45021 ),
 .UNSPECIFIED., .F., .F.,
 ( 4, 4 ),
 ( 0.8746029590009303245, 1.000000000000000000 ),
 .UNSPECIFIED. ) ;
#13551=EDGE_CURVE ( 'NONE', #49429, #34400, #56731, .T. ) ;
#13556=CARTESIAN_POINT ( 'NONE',  ( 7.886566940378000545, -3.084082018960999871, 9.259837032825000591 ) ) ;
#13567=CARTESIAN_POINT ( 'NONE',  ( 9.341483607044001047, -4.148132978932999926, 9.337467253566000380 ) ) ;
#13582=CARTESIAN_POINT ( 'NONE',  ( 10.00122642709000154, -2.274091010763000131, 7.851325450887000734 ) ) ;
#13589=CARTESIAN_POINT ( 'NONE',  ( 8.026781271869193546, -2.988395543640873786, 6.057288563851790819 ) ) ;
#13590=CARTESIAN_POINT ( 'NONE',  ( 10.93227479887999998, -2.539880901735999785, 6.453614191797999666 ) ) ;
#13594=CARTESIAN_POINT ( 'NONE',  ( 11.03703505992000089, -5.149240112441999528, -5.120435640197999128 ) ) ;
#13599=CARTESIAN_POINT ( 'NONE',  ( 9.842321917838999568, -3.423478821957000040, -6.068694811299999436 ) ) ;
#13606=EDGE_CURVE ( 'NONE', #54965, #65525, #50817, .T. ) ;
#13609=CARTESIAN_POINT ( 'NONE',  ( 8.791230646795000325, -5.095088356574999366, 6.286978111459999852 ) ) ;
#13614=CARTESIAN_POINT ( 'NONE',  ( 11.26847231345999845, -2.565616654150999931, -7.116622328138999976 ) ) ;
#13632=EDGE_CURVE ( 'NONE', #31558, #61812, #67602, .T. ) ;
#13633=CARTESIAN_POINT ( 'NONE',  ( 10.98768472633000037, -5.449702618601000026, 4.945212061625999134 ) ) ;
#13647=B_SPLINE_CURVE_WITH_KNOTS ( 'NONE', 3,
 ( #46703, #68007, #19783, #19436, #41452 ),
 .UNSPECIFIED., .F., .F.,
 ( 4, 1, 4 ),
 ( 0.000000000000000000, 0.006423492687020981168, 0.1253905405517105054 ),
 .UNSPECIFIED. ) ;
#13648=CARTESIAN_POINT ( 'NONE',  ( 10.82095911837782154, -4.087393693045735077, 9.237492157467196208 ) ) ;
#13649=CARTESIAN_POINT ( 'NONE',  ( 8.689254440380000943, -2.550228841911000188, 7.666975032000999946 ) ) ;
#13663=CARTESIAN_POINT ( 'NONE',  ( 7.795980646793000624, -3.164807285701999984, 9.104732190648000767 ) ) ;
#13667=LINE ( 'NONE', #23803, #36240 ) ;
#13668=CARTESIAN_POINT ( 'NONE',  ( 7.437825695874983545, -2.276412617413176687, 7.746772493203951448 ) ) ;
#13669=AXIS2_PLACEMENT_3D ( 'NONE', #2201, #7088, #44517 ) ;
#13679=CARTESIAN_POINT ( 'NONE',  ( 11.35905860703999970, -2.719090443614000208, -7.157642341559000698 ) ) ;
#13697=CARTESIAN_POINT ( 'NONE',  ( 9.813358178091998951, -5.349400659402999914, 6.657024270273000255 ) ) ;
#13704=CARTESIAN_POINT ( 'NONE',  ( 11.12439163055999991, -6.498888995361999932, -5.558825371164000551 ) ) ;
#13711=CARTESIAN_POINT ( 'NONE',  ( 10.22399006116000031, -5.507891002176999784, 6.589804341508000540 ) ) ;
#13725=CARTESIAN_POINT ( 'NONE',  ( 9.436149330669000079, -3.485164486501000081, -6.221839249167999242 ) ) ;
#13735=CARTESIAN_POINT ( 'NONE',  ( 9.786673210037999837, -2.381198102024000285, 7.612749732462000374 ) ) ;
#13749=CARTESIAN_POINT ( 'NONE',  ( 10.88829480895999957, -2.943348573720999894, 5.042864669073000350 ) ) ;
#13752=CARTESIAN_POINT ( 'NONE',  ( 9.707908211423999845, -3.300107492866999781, -5.762405935562999737 ) ) ;
#13756=CARTESIAN_POINT ( 'NONE',  ( 11.04678944127999962, -5.235596213805000509, -5.039805523473999571 ) ) ;
#13763=ORIENTED_EDGE ( 'NONE', *, *, #22466, .T. ) ;
#13764=CARTESIAN_POINT ( 'NONE',  ( 9.125465313390733968, -5.349725526283760857, -7.676666018642554157 ) ) ;
#13767=EDGE_CURVE ( 'NONE', #40775, #20272, #25892, .T. ) ;
#13774=CARTESIAN_POINT ( 'NONE',  ( 11.03775575519999919, -8.050335494570999728, 6.914609630061999468 ) ) ;
#13775=VERTEX_POINT ( 'NONE', #4283 ) ;
#13777=( BOUNDED_SURFACE ( )  B_SPLINE_SURFACE ( 3, 3, ( 
 ( #1185, #1525, #44544, #22494, #17962, #39280, #12712, #23540 ),
 ( #39628, #60949, #13064, #7808, #14438, #19325, #29845, #35759 ),
 ( #19678, #25260, #45902, #8497, #20361, #36097, #3582, #14778 ),
 ( #46599, #51486, #57074, #61983, #56745, #34733, #46937, #57412 ) ),
 .UNSPECIFIED., .F., .F., .F. ) 
 B_SPLINE_SURFACE_WITH_KNOTS ( ( 4, 4 ),
 ( 4, 1, 1, 1, 1, 4 ),
 ( 0.000000000000000000, 1.000000000000000000 ),
 ( 0.8111870735734000304, 0.8462787474214000794, 0.8943647847192999212, 0.9442642648822999751, 1.000000000000000000, 1.006078322774000000 ),
 .UNSPECIFIED. ) 
 GEOMETRIC_REPRESENTATION_ITEM ( )  RATIONAL_B_SPLINE_SURFACE ( (
 ( 1.221012505305000051, 1.221012505305000051, 1.221012505305000051, 1.221012505305000051, 1.221012505305000051, 1.221012505305000051, 1.221012505305000051, 1.221012505305000051),
 ( 0.9263291648981999415, 0.9263291648981999415, 0.9263291648981999415, 0.9263291648981999415, 0.9263291648981999415, 0.9263291648981999415, 0.9263291648981999415, 0.9263291648981999415),
 ( 0.9263291648981999415, 0.9263291648981999415, 0.9263291648981999415, 0.9263291648981999415, 0.9263291648981999415, 0.9263291648981999415, 0.9263291648981999415, 0.9263291648981999415),
 ( 1.221012505305000051, 1.221012505305000051, 1.221012505305000051, 1.221012505305000051, 1.221012505305000051, 1.221012505305000051, 1.221012505305000051, 1.221012505305000051) ) ) 
 REPRESENTATION_ITEM ( '' )  SURFACE ( )  );
#13782=CARTESIAN_POINT ( 'NONE',  ( 10.99600480934999958, -8.065001534460998656, 6.834777879866000383 ) ) ;
#13789=DIRECTION ( 'NONE',  ( 0.9999999999976796339, 1.847154591387964169E-06, 1.108402172101977569E-06 ) ) ;
#13790=CARTESIAN_POINT ( 'NONE',  ( 9.446897644051269083, -2.250365900417164777, 7.566722005472066748 ) ) ;
#13794=CARTESIAN_POINT ( 'NONE',  ( 9.865944350586199008, -5.673398084260703023, -8.064521635305629488 ) ) ;
#13799=CARTESIAN_POINT ( 'NONE',  ( 10.71756905878999966, -3.040221764047000175, 8.808455607108001573 ) ) ;
#13801=CARTESIAN_POINT ( 'NONE',  ( 10.97571094393200042, -2.824289056067999848, 6.306988371318333897 ) ) ;
#13805=ORIENTED_EDGE ( 'NONE', *, *, #37169, .F. ) ;
#13817=CARTESIAN_POINT ( 'NONE',  ( 10.42702554439000195, -2.952854773874999950, 4.671719621119999388 ) ) ;
#13819=CARTESIAN_POINT ( 'NONE',  ( 10.59654005035000068, -3.014401618106000047, -5.075934621078999953 ) ) ;
#13820=CARTESIAN_POINT ( 'NONE',  ( 9.666315108303999537, -3.197530835772000035, -8.817973615970998935 ) ) ;
#13828=B_SPLINE_CURVE_WITH_KNOTS ( 'NONE', 3,
 ( #10983, #32323, #48738, #20788, #59565 ),
 .UNSPECIFIED., .F., .F.,
 ( 4, 1, 4 ),
 ( 0.000000000000000000, 0.5000000000000000000, 1.000000000000000000 ),
 .UNSPECIFIED. ) ;
#13837=CARTESIAN_POINT ( 'NONE',  ( 10.12947109217999930, -5.100000000000000533, 6.152188490330000370 ) ) ;
#13847=CARTESIAN_POINT ( 'NONE',  ( 9.590594544025000445, -2.445960766574000189, 7.841185849078001091 ) ) ;
#13848=ORIENTED_EDGE ( 'NONE', *, *, #4865, .T. ) ;
#13850=CARTESIAN_POINT ( 'NONE',  ( 8.507041456382204103, -3.224154684601456822, 6.000520319185582707 ) ) ;
#13851=CARTESIAN_POINT ( 'NONE',  ( 8.817629440380001071, -3.894643656844000379, 6.044452984962999764 ) ) ;
#13855=CARTESIAN_POINT ( 'NONE',  ( 11.07503769033554342, -4.268003910456493522, -9.025037683630598551 ) ) ;
#13860=CARTESIAN_POINT ( 'NONE',  ( 10.83668192271000130, -4.288535286065000562, 9.448729895547000268 ) ) ;
#13862=DIRECTION ( 'NONE',  ( 0.000000000000000000, -1.000000000000000000, 0.000000000000000000 ) ) ;
#13865=DIRECTION ( 'NONE',  ( -0.7071067811865474617, -0.7071067811865474617, -9.650793108809640698E-10 ) ) ;
#13868=CARTESIAN_POINT ( 'NONE',  ( 10.91620964606000044, -2.818413279081999789, -6.814156272943999504 ) ) ;
#13872=AXIS2_PLACEMENT_3D ( 'NONE', #18648, #35083, #24580 ) ;
#13883=CARTESIAN_POINT ( 'NONE',  ( 10.91623602276999883, -5.459825388708999583, -8.642870457474998602 ) ) ;
#13885=CARTESIAN_POINT ( 'NONE',  ( 9.618481599739016730, -2.362941927002724096, -6.884006425641727489 ) ) ;
#13887=EDGE_CURVE ( 'NONE', #17344, #32816, #57985, .T. ) ;
#13893=CARTESIAN_POINT ( 'NONE',  ( 8.014941940377999785, -2.280579276705999803, 6.510290672242000198 ) ) ;
#13905=CARTESIAN_POINT ( 'NONE',  ( 7.037120559622001004, -4.623636604834999275, 8.651469651195000665 ) ) ;
#13921=LINE ( 'NONE', #4094, #23186 ) ;
#13922=ORIENTED_EDGE ( 'NONE', *, *, #33931, .T. ) ;
#13924=CARTESIAN_POINT ( 'NONE',  ( 11.37167944038000122, -2.803484087760999888, -6.967877228197000505 ) ) ;
#13926=CARTESIAN_POINT ( 'NONE',  ( 8.069163351475221901, -3.878260955912923080, 5.763835643759676941 ) ) ;
#13930=CARTESIAN_POINT ( 'NONE',  ( 10.39968959185000053, -4.894615431365999747, -4.742639820717000632 ) ) ;
#13932=ORIENTED_EDGE ( 'NONE', *, *, #6857, .T. ) ;
#13933=ADVANCED_FACE ( 'NONE', ( #38158 ), #43426, .T. ) ;
#13936=CARTESIAN_POINT ( 'NONE',  ( 9.353137413980999071, -5.679455740088000582, -8.329752476417999318 ) ) ;
#13947=CARTESIAN_POINT ( 'NONE',  ( 8.983793146794999629, -3.979464503892999439, 9.134080454305001595 ) ) ;
#13953=CARTESIAN_POINT ( 'NONE',  ( 10.39539435320999949, -5.667179153637999178, -7.250689665673000661 ) ) ;
#13960=CARTESIAN_POINT ( 'NONE',  ( 8.550568453843245820, -5.068330482988463004, 6.313212389168451288 ) ) ;
#13970=ADVANCED_FACE ( 'NONE', ( #27690 ), #15810, .T. ) ;
#13973=CARTESIAN_POINT ( 'NONE',  ( 10.21921441925097973, -4.353287638977898055, -8.814644987550590116 ) ) ;
#13992=CARTESIAN_POINT ( 'NONE',  ( 9.202754440379999679, -2.542850487891999745, 7.419808283050000064 ) ) ;
#14001=FACE_OUTER_BOUND ( 'NONE', #26776, .T. ) ;
#14005=CARTESIAN_POINT ( 'NONE',  ( 5.700000000000000178, 0.000000000000000000, 0.000000000000000000 ) ) ;
#14006=CARTESIAN_POINT ( 'NONE',  ( 9.170316940378999249, -5.558929022707999046, 6.272984818914999927 ) ) ;
#14007=ORIENTED_EDGE ( 'NONE', *, *, #68985, .F. ) ;
#14010=CARTESIAN_POINT ( 'NONE',  ( 7.450458831010640992, -2.261073438131606217, 7.470018516072758352 ) ) ;
#14016=CARTESIAN_POINT ( 'NONE',  ( 10.27427156480999848, -4.600000212792999754, 4.944156960788000710 ) ) ;
#14021=CARTESIAN_POINT ( 'NONE',  ( 8.682949004128220238, -5.079917234190865827, 6.251799941949381711 ) ) ;
#14023=EDGE_CURVE ( 'NONE', #46365, #46842, #46602, .T. ) ;
#14039=CARTESIAN_POINT ( 'NONE',  ( 10.57223537388000167, -4.020426196685999543, 8.920680607665000039 ) ) ;
#14070=CARTESIAN_POINT ( 'NONE',  ( 9.311892889969000109, -5.494586520014999920, -6.370782351137999733 ) ) ;
#14081=CARTESIAN_POINT ( 'NONE',  ( 9.228135700785001561, -2.875364528161000077, 8.669943154892999715 ) ) ;
#14085=CYLINDRICAL_SURFACE ( 'NONE', #65392, 1.350000000000000089 ) ;
#14087=ORIENTED_EDGE ( 'NONE', *, *, #56664, .F. ) ;
#14097=CARTESIAN_POINT ( 'NONE',  ( 9.866664898013999263, -4.626219091573998909, -9.027249334595000008 ) ) ;
#14112=ORIENTED_EDGE ( 'NONE', *, *, #956, .F. ) ;
#14138=CARTESIAN_POINT ( 'NONE',  ( 7.997739111735391759, -4.828320830117715623, 8.578514095141958506 ) ) ;
#14145=CARTESIAN_POINT ( 'NONE',  ( 10.80160188108999897, -2.805072368922999715, -8.157282064671999677 ) ) ;
#14158=CARTESIAN_POINT ( 'NONE',  ( 8.755016320410998532, -4.513710855956997392, -6.314259950256001730 ) ) ;
#14163=CARTESIAN_POINT ( 'NONE',  ( 11.07605693148000015, -2.665626082328999669, -4.951852240693000340 ) ) ;
#14164=CARTESIAN_POINT ( 'NONE',  ( 9.485142521132999605, -3.025808284870999731, -9.100010361367001366 ) ) ;
#14183=LINE ( 'NONE', #30950, #33217 ) ;
#14188=CARTESIAN_POINT ( 'NONE',  ( 10.68361719090999884, -2.603550124652000086, 7.762065570229999878 ) ) ;
#14191=CARTESIAN_POINT ( 'NONE',  ( 7.828418146791999099, -5.524126964933000927, 6.910359834012999691 ) ) ;
#14200=CIRCLE ( 'NONE', #9685, 1.449999999999999956 ) ;
#14201=CARTESIAN_POINT ( 'NONE',  ( 10.90454231406000041, -5.099691312770999296, -5.130383474399000221 ) ) ;
#14203=EDGE_LOOP ( 'NONE', ( #63737, #38614, #47062, #33196 ) ) ;
#14204=CARTESIAN_POINT ( 'NONE',  ( 9.347248564704999652, -4.028326926800000152, 9.469437404464001062 ) ) ;
#14207=CARTESIAN_POINT ( 'NONE',  ( 10.01597818573999987, -4.792673671522000411, -6.390249203106999509 ) ) ;
#14211=DIRECTION ( 'NONE',  ( 0.000000000000000000, 0.000000000000000000, -1.000000000000000000 ) ) ;
#14217=ORIENTED_EDGE ( 'NONE', *, *, #58349, .F. ) ;
#14220=EDGE_CURVE ( 'NONE', #64705, #13225, #41269, .T. ) ;
#14227=CARTESIAN_POINT ( 'NONE',  ( 10.71983009893999927, -3.571743996388999864, -5.696159701115999674 ) ) ;
#14229=CARTESIAN_POINT ( 'NONE',  ( 8.991740795306689904, -5.328224142454163648, 7.781282113468042994 ) ) ;
#14248=CARTESIAN_POINT ( 'NONE',  ( 9.181706853207000307, -3.734278838175999482, 8.942129638874000364 ) ) ;
#14261=PLANE ( 'NONE',  #58808 ) ;
#14263=CARTESIAN_POINT ( 'NONE',  ( 11.00589466765999802, -3.012766713855000056, 5.961506477028999385 ) ) ;
#14268=CARTESIAN_POINT ( 'NONE',  ( 8.254953780971833410, -5.339409724223009412, 8.610099718891319753 ) ) ;
#14272=CARTESIAN_POINT ( 'NONE',  ( 11.03280546629000014, -5.245089378378999356, -5.027159640631999160 ) ) ;
#14280=CARTESIAN_POINT ( 'NONE',  ( 9.925159544971000614, -4.365624317997999881, -9.242254741729000855 ) ) ;
#14290=CARTESIAN_POINT ( 'NONE',  ( 9.587879440377001572, -3.762710033898000184, 8.787827024292999667 ) ) ;
#14296=CARTESIAN_POINT ( 'NONE',  ( 11.28109314679000086, -2.660122028910999692, -6.904120269057000492 ) ) ;
#14314=CARTESIAN_POINT ( 'NONE',  ( 8.828674827949001269, -4.601003974012999542, -6.242416087727000296 ) ) ;
#14318=CARTESIAN_POINT ( 'NONE',  ( 10.34423739839155409, -2.685214518266378469, -7.853261023685102593 ) ) ;
#14345=VECTOR ( 'NONE', #29043, 1000.000000000000000 ) ;
#14348=DIRECTION ( 'NONE',  ( 1.000000000000000000, 3.552713678802000396E-14, 5.329070518202999332E-14 ) ) ;
#14349=CARTESIAN_POINT ( 'NONE',  ( 8.694605646795000808, -5.290204991635000020, 8.768102264518001121 ) ) ;
#14353=CARTESIAN_POINT ( 'NONE',  ( 10.22908305962000064, -4.838492992840000007, -5.852445959518000507 ) ) ;
#14354=CARTESIAN_POINT ( 'NONE',  ( 7.641402119058184894, -5.301423981906861371, 6.346217268197262840 ) ) ;
#14362=CARTESIAN_POINT ( 'NONE',  ( 11.00350689643929947, -3.174004326299003420, -9.060806138410798738 ) ) ;
#14369=EDGE_CURVE ( 'NONE', #22433, #25113, #28749, .T. ) ;
#14379=CARTESIAN_POINT ( 'NONE',  ( 10.67905590578999941, -2.899999999999999911, 6.571291218949999902 ) ) ;
#14385=CARTESIAN_POINT ( 'NONE',  ( 9.442085454646999665, -4.742494605615999781, 8.809986937145000141 ) ) ;
#14387=CARTESIAN_POINT ( 'NONE',  ( 10.83767365324000131, -5.758089526411000136, -6.911472812823999945 ) ) ;
#14389=DIRECTION ( 'NONE',  ( 0.000000000000000000, 1.000000000000000000, 0.000000000000000000 ) ) ;
#14390=B_SPLINE_CURVE_WITH_KNOTS ( 'NONE', 3,
 ( #13774, #36121, #2927, #41713 ),
 .UNSPECIFIED., .F., .F.,
 ( 4, 4 ),
 ( 0.000000000000000000, 1.000000000000000000 ),
 .UNSPECIFIED. ) ;
#14391=ORIENTED_EDGE ( 'NONE', *, *, #21765, .F. ) ;
#14392=CARTESIAN_POINT ( 'NONE',  ( 11.01665874711000015, -6.699714419246999952, -5.516646458005999953 ) ) ;
#14416=CARTESIAN_POINT ( 'NONE',  ( 9.707908211423999845, -3.300107492866999781, -5.762405935562999737 ) ) ;
#14431=CARTESIAN_POINT ( 'NONE',  ( 10.12947109217999930, -5.100000000000000533, 6.152188490330000370 ) ) ;
#14434=B_SPLINE_CURVE_WITH_KNOTS ( 'NONE', 3,
 ( #64464, #42817, #37563, #15564, #27783 ),
 .UNSPECIFIED., .F., .F.,
 ( 4, 1, 4 ),
 ( 0.000000000000000000, 0.5000000000000000000, 1.000000000000000000 ),
 .UNSPECIFIED. ) ;
#14435=LINE ( 'NONE', #36093, #47722 ) ;
#14438=CARTESIAN_POINT ( 'NONE',  ( 8.848090123393001605, -2.900413175355999851, -6.422155424834999238 ) ) ;
#14444=CARTESIAN_POINT ( 'NONE',  ( 9.683745612763230426, -2.796157461453096182, 8.204744624355374327 ) ) ;
#14450=CARTESIAN_POINT ( 'NONE',  ( 10.91620964606000044, -2.818413279081999789, -6.814156272943999504 ) ) ;
#14454=CARTESIAN_POINT ( 'NONE',  ( 8.528661480133219897, -4.352698949119082172, 8.815590613233990069 ) ) ;
#14466=DIRECTION ( 'NONE',  ( 0.7071067811866525998, 0.000000000000000000, -0.7071067811864425456 ) ) ;
#14470=EDGE_CURVE ( 'NONE', #21511, #67420, #2151, .T. ) ;
#14471=B_SPLINE_CURVE_WITH_KNOTS ( 'NONE', 3,
 ( #34855, #60034, #49893, #50239, #56170 ),
 .UNSPECIFIED., .F., .F.,
 ( 4, 1, 4 ),
 ( 0.000000000000000000, 0.5000000000000000000, 1.000000000000000000 ),
 .UNSPECIFIED. ) ;
#14480=CARTESIAN_POINT ( 'NONE',  ( 10.48632761434999949, -8.229716073962000777, -6.713145785397999887 ) ) ;
#14488=CARTESIAN_POINT ( 'NONE',  ( 10.47094409420000005, -5.100000000000000533, 6.571291218949999902 ) ) ;
#14500=CARTESIAN_POINT ( 'NONE',  ( 8.468724635341004614, -4.797383707087001348, -6.431807026291995300 ) ) ;
#14504=CARTESIAN_POINT ( 'NONE',  ( 9.221132306829000314, -4.645169647889000331, -5.840816811670999975 ) ) ;
#14506=CARTESIAN_POINT ( 'NONE',  ( 11.04384236319999957, -7.396937235950000300, 6.274987567768999241 ) ) ;
#14509=B_SPLINE_CURVE_WITH_KNOTS ( 'NONE', 3,
 ( #55828, #60719, #12835, #34162, #1997 ),
 .UNSPECIFIED., .F., .F.,
 ( 4, 1, 4 ),
 ( 0.000000000000000000, 0.002767885366475097975, 0.1253844953241992632 ),
 .UNSPECIFIED. ) ;
#14513=B_SPLINE_CURVE_WITH_KNOTS ( 'NONE', 3,
 ( #33496, #8976, #30651, #62455 ),
 .UNSPECIFIED., .F., .F.,
 ( 4, 4 ),
 ( 0.000000000000000000, 1.000000000000000000 ),
 .UNSPECIFIED. ) ;
#14523=CARTESIAN_POINT ( 'NONE',  ( 7.225322421146570306, -2.650264760010439868, 7.500018091723870128 ) ) ;
#14524=EDGE_LOOP ( 'NONE', ( #50174, #56739, #4696, #6432, #21543 ) ) ;
#14528=ADVANCED_FACE ( 'NONE', ( #52283 ), #6187, .T. ) ;
#14534=CARTESIAN_POINT ( 'NONE',  ( 10.25888544622000076, -4.512389816463000081, 5.993697694029000544 ) ) ;
#14543=DIRECTION ( 'NONE',  ( -0.7071067811866525998, 0.000000000000000000, -0.7071067811864425456 ) ) ;
#14546=CARTESIAN_POINT ( 'NONE',  ( 9.194602547868999665, -5.157768569202000108, 8.637845986715998237 ) ) ;
#14550=EDGE_CURVE ( 'NONE', #53746, #21776, #1937, .T. ) ;
#14552=CARTESIAN_POINT ( 'NONE',  ( 9.299999999999998934, -4.537600397704999899, 9.154563893594000135 ) ) ;
#14562=CARTESIAN_POINT ( 'NONE',  ( 8.354417780085995560, -5.125509315120996057, 6.367236178909004174 ) ) ;
#14572=CARTESIAN_POINT ( 'NONE',  ( 9.038117261819090587, -4.950750304293762838, 8.458219317142523508 ) ) ;
#14573=ORIENTED_EDGE ( 'NONE', *, *, #42168, .F. ) ;
#14588=CARTESIAN_POINT ( 'NONE',  ( 8.128308059623998716, -3.117370956513999758, 8.662188901935000018 ) ) ;
#14610=CARTESIAN_POINT ( 'NONE',  ( 8.284908184216730476, -4.822684648958374787, 9.032360259545255232 ) ) ;
#14613=CARTESIAN_POINT ( 'NONE',  ( 10.92233852386999970, -5.248250142883000180, -4.977516224977000192 ) ) ;
#14618=CARTESIAN_POINT ( 'NONE',  ( 10.02091161619000026, -4.911674715448000050, -6.466751564808000730 ) ) ;
#14627=CARTESIAN_POINT ( 'NONE',  ( 8.032370559622998840, -3.524751762020000179, 5.573845465339999805 ) ) ;
#14633=CARTESIAN_POINT ( 'NONE',  ( 10.22094314679000071, -2.563075248996000255, -8.004105227364998854 ) ) ;
#14640=CONICAL_SURFACE ( 'NONE', #53710, 1.449999999965999375, 0.7853981633972997312 ) ;
#14642=VERTEX_POINT ( 'NONE', #8868 ) ;
#14644=VERTEX_POINT ( 'NONE', #50484 ) ;
#14656=ORIENTED_EDGE ( 'NONE', *, *, #57050, .F. ) ;
#14665=EDGE_CURVE ( 'NONE', #7917, #28326, #57101, .T. ) ;
#14668=B_SPLINE_CURVE_WITH_KNOTS ( 'NONE', 3,
 ( #49353, #16505, #37833, #33290 ),
 .UNSPECIFIED., .F., .F.,
 ( 4, 4 ),
 ( 0.000000000000000000, 1.000000000000000000 ),
 .UNSPECIFIED. ) ;
#14683=DIRECTION ( 'NONE',  ( 0.000000000000000000, 1.000000000000000000, 0.000000000000000000 ) ) ;
#14687=DIRECTION ( 'NONE',  ( 0.000000000000000000, -0.8648648648648717963, 0.5020047465136829867 ) ) ;
#14688=CARTESIAN_POINT ( 'NONE',  ( 8.014941940377999785, -2.280579276705999803, 6.510290672242000198 ) ) ;
#14694=CARTESIAN_POINT ( 'NONE',  ( 7.637790262712637279, -5.247290350387737945, 6.287244541376254325 ) ) ;
#14695=CARTESIAN_POINT ( 'NONE',  ( 7.932045726517200634, -5.134137217805110787, 6.756605349134713556 ) ) ;
#14707=CARTESIAN_POINT ( 'NONE',  ( 10.98358762163081259, -5.203662202021275718, 6.699115767914069153 ) ) ;
#14712=CARTESIAN_POINT ( 'NONE',  ( 8.647350449577999143, -5.160012848592001156, -6.809278868592000933 ) ) ;
#14713=CARTESIAN_POINT ( 'NONE',  ( 10.63706886433642573, -2.899999999999999911, 6.444141223494331605 ) ) ;
#14722=CARTESIAN_POINT ( 'NONE',  ( 10.79499900793999956, -3.503951165873000040, 6.168577387731000172 ) ) ;
#14724=CARTESIAN_POINT ( 'NONE',  ( 5.700000001242999659, 1.249999998757000075, -1.883720587326999896E-09 ) ) ;
#14729=CARTESIAN_POINT ( 'NONE',  ( 11.07127482541000063, -6.556071284744000138, -5.494407061017000160 ) ) ;
#14747=EDGE_CURVE ( 'NONE', #67420, #44775, #51292, .T. ) ;
#14751=CARTESIAN_POINT ( 'NONE',  ( 9.839913318575998602, -5.792391408692000532, -6.955579396894000510 ) ) ;
#14759=CARTESIAN_POINT ( 'NONE',  ( 10.33253786428999987, -2.899999999999999911, 6.571291218949999902 ) ) ;
#14763=LINE ( 'NONE', #7794, #4298 ) ;
#14768=FACE_BOUND ( 'NONE', #2294, .T. ) ;
#14775=CARTESIAN_POINT ( 'NONE',  ( 10.61815932168150312, -5.019094019303483201, -5.036897186739046184 ) ) ;
#14778=CARTESIAN_POINT ( 'NONE',  ( 8.894507664004006386, -3.102842363045003271, -6.153768356943001727 ) ) ;
#14781=CARTESIAN_POINT ( 'NONE',  ( 9.575903104272999400, -2.330665094450000030, -8.349943402163999551 ) ) ;
#14782=CARTESIAN_POINT ( 'NONE',  ( 10.91060805961999947, -4.702347118766000200, -9.210032991522000501 ) ) ;
#14783=CARTESIAN_POINT ( 'NONE',  ( 9.558834163536323203, -4.704973616088924615, 8.704082162066264061 ) ) ;
#14792=CARTESIAN_POINT ( 'NONE',  ( 8.424688440789097399, -5.350083765069893360, 7.500019236172019710 ) ) ;
#14819=CARTESIAN_POINT ( 'NONE',  ( 8.154130060498479438, -2.684642961096272096, 7.853228170896902505 ) ) ;
#14824=CARTESIAN_POINT ( 'NONE',  ( 11.02205565301999890, -2.309485172892000282, -7.515673712097999726 ) ) ;
#14838=CARTESIAN_POINT ( 'NONE',  ( 8.205380712518003605, -3.106081630192000009, 6.107045428706002532 ) ) ;
#14841=CARTESIAN_POINT ( 'NONE',  ( 10.37169758536000153, -3.424645824523000037, -5.010422874381999847 ) ) ;
#14842=CARTESIAN_POINT ( 'NONE',  ( 9.580894592352999339, -5.371875912611999482, -7.370590366721999409 ) ) ;
#14844=DIRECTION ( 'NONE',  ( 0.000000000000000000, -0.7071067811865475727, 0.7071067811865475727 ) ) ;
#14845=CARTESIAN_POINT ( 'NONE',  ( 10.99827931143999926, -5.289657308675000280, -4.962166337294999785 ) ) ;
#14849=CARTESIAN_POINT ( 'NONE',  ( 7.935252636294002571, -4.895109672515001620, 6.296391117214003685 ) ) ;
#14850=VECTOR ( 'NONE', #56581, 1000.000000000000000 ) ;
#14862=DIRECTION ( 'NONE',  ( 1.000000000000000000, 1.776356839496000193E-14, -1.776356839496000193E-14 ) ) ;
#14868=CARTESIAN_POINT ( 'NONE',  ( 10.92717634842000152, -5.023656093247000243, 8.718039182945998888 ) ) ;
#14871=CARTESIAN_POINT ( 'NONE',  ( 7.352706853207999771, -4.773080213113000347, 8.927399220053999329 ) ) ;
#14878=ADVANCED_FACE ( 'NONE', ( #20387 ), #38096, .F. ) ;
#14882=CARTESIAN_POINT ( 'NONE',  ( 9.905786073958001481, -2.698967003257000119, 8.979227319929000473 ) ) ;
#14883=AXIS2_PLACEMENT_3D ( 'NONE', #38786, #40096, #56158 ) ;
#14887=CARTESIAN_POINT ( 'NONE',  ( 9.937415816209998809, -3.510658118802999716, -6.227041669085999764 ) ) ;
#14889=CARTESIAN_POINT ( 'NONE',  ( 10.90000000016000037, -5.167567554889999748, 6.822293570050000255 ) ) ;
#14896=CARTESIAN_POINT ( 'NONE',  ( 7.936333720142999759, -5.123034382927999175, 6.721303993095999907 ) ) ;
#14907=CARTESIAN_POINT ( 'NONE',  ( 10.15786958814999963, -4.213496663054999480, -5.822956951053000374 ) ) ;
#14926=CARTESIAN_POINT ( 'NONE',  ( 7.641206853206999661, -4.524489047957000132, 9.047757046927999980 ) ) ;
#14940=LINE ( 'NONE', #53722, #20050 ) ;
#14944=CARTESIAN_POINT ( 'NONE',  ( 8.279953265935446893, -4.917462069712163597, 8.978228541670741691 ) ) ;
#14969=CARTESIAN_POINT ( 'NONE',  ( 10.35753185321000025, -5.367809014988999650, -6.514738374536999999 ) ) ;
#14978=ORIENTED_EDGE ( 'NONE', *, *, #45151, .T. ) ;
#14979=CYLINDRICAL_SURFACE ( 'NONE', #28331, 10.75000000000000000 ) ;
#14989=CARTESIAN_POINT ( 'NONE',  ( 10.97462572286999993, -5.299102401333000145, -4.938840653320999863 ) ) ;
#14991=VERTEX_POINT ( 'NONE', #49199 ) ;
#15022=EDGE_LOOP ( 'NONE', ( #56827, #36196, #19110, #22253, #26765, #22266, #24431, #59334 ) ) ;
#15026=CYLINDRICAL_SURFACE ( 'NONE', #26571, 0.5000000000000002220 ) ;
#15027=CARTESIAN_POINT ( 'NONE',  ( 9.106129440379998385, -4.192917962110999319, 5.525484568403999930 ) ) ;
#15030=CARTESIAN_POINT ( 'NONE',  ( 10.01721296880960033, -5.205658458020572255, 8.206277775804004193 ) ) ;
#15031=CARTESIAN_POINT ( 'NONE',  ( 10.83488305961999920, -5.800181157098999840, -7.920538492179999501 ) ) ;
#15032=CARTESIAN_POINT ( 'NONE',  ( 7.595706369369626287, -4.453886063348286406, 5.820683931063973304 ) ) ;
#15050=CARTESIAN_POINT ( 'NONE',  ( 10.52052890781999928, -2.899999999999999911, 6.152188490330000370 ) ) ;
#15052=CARTESIAN_POINT ( 'NONE',  ( 10.42702345793999896, -5.047055844931000124, 4.671718569916000874 ) ) ;
#15060=CARTESIAN_POINT ( 'NONE',  ( 9.854949224988001077, -2.800315695760000168, 9.013807298610000629 ) ) ;
#15067=DIRECTION ( 'NONE',  ( 0.000000000000000000, 1.000000000000000000, 0.000000000000000000 ) ) ;
#15072=CARTESIAN_POINT ( 'NONE',  ( 11.11504459742000073, -3.456612073675000119, 5.970342812640000218 ) ) ;
#15075=EDGE_CURVE ( 'NONE', #53746, #40911, #14471, .T. ) ;
#15080=CARTESIAN_POINT ( 'NONE',  ( 9.662553763536999796, -4.094830574823999925, 9.119950378356000087 ) ) ;
#15091=CARTESIAN_POINT ( 'NONE',  ( 9.619904806657000762, -2.133039813254999917, -7.346564890486999566 ) ) ;
#15110=VERTEX_POINT ( 'NONE', #18083 ) ;
#15115=DIRECTION ( 'NONE',  ( 0.4682208595141937879, -0.4682208595141937879, 0.7493586947727897130 ) ) ;
#15117=B_SPLINE_CURVE_WITH_KNOTS ( 'NONE', 3,
 ( #66865, #61624, #51476, #29834 ),
 .UNSPECIFIED., .F., .F.,
 ( 4, 4 ),
 ( 0.000000000000000000, 1.000000000000000000 ),
 .UNSPECIFIED. ) ;
#15122=CARTESIAN_POINT ( 'NONE',  ( 11.13491264576000006, -2.665455753003000527, -5.170164771427000261 ) ) ;
#15123=CARTESIAN_POINT ( 'NONE',  ( 9.970944094204998720, -5.100000000000000533, 6.571291218949999902 ) ) ;
#15129=CARTESIAN_POINT ( 'NONE',  ( 9.074999999999999289, -4.417172942406000224, 8.783926296998000538 ) ) ;
#15130=VERTEX_POINT ( 'NONE', #60725 ) ;
#15134=FACE_OUTER_BOUND ( 'NONE', #31248, .T. ) ;
#15142=CARTESIAN_POINT ( 'NONE',  ( 9.378359312499400247, -5.126777126185184663, 6.752018918871678821 ) ) ;
#15144=CARTESIAN_POINT ( 'NONE',  ( 10.99999999997000089, -4.000000000000000000, -7.500000000000000000 ) ) ;
#15148=ORIENTED_EDGE ( 'NONE', *, *, #27354, .T. ) ;
#15160=CARTESIAN_POINT ( 'NONE',  ( 7.935182732229959512, -5.348502701843340645, 7.676951299079880719 ) ) ;
#15162=EDGE_CURVE ( 'NONE', #51247, #23850, #56689, .T. ) ;
#15165=CARTESIAN_POINT ( 'NONE',  ( 9.988720925027999797, -2.842024021884000273, -6.504330542082999322 ) ) ;
#15166=EDGE_LOOP ( 'NONE', ( #35586, #53992, #2975, #36225, #49061, #54756 ) ) ;
#15169=CARTESIAN_POINT ( 'NONE',  ( 10.92799928938507925, -5.127999289385079429, -6.526892970155856233 ) ) ;
#15177=ORIENTED_EDGE ( 'NONE', *, *, #7679, .T. ) ;
#15179=EDGE_CURVE ( 'NONE', #4537, #59620, #20276, .T. ) ;
#15181=CARTESIAN_POINT ( 'NONE',  ( 8.046990059540997109, -3.146252403201002856, 6.173090499042001689 ) ) ;
#15183=CARTESIAN_POINT ( 'NONE',  ( 11.09999999999999964, -2.649999999999999911, -7.500000000000000000 ) ) ;
#15184=CARTESIAN_POINT ( 'NONE',  ( 9.815199780373001559, -2.813634733202999616, 8.848854270764999086 ) ) ;
#15201=VERTEX_POINT ( 'NONE', #40103 ) ;
#15209=CARTESIAN_POINT ( 'NONE',  ( 10.27968096967000022, -5.739708848514999850, 7.774962785835000112 ) ) ;
#15212=CARTESIAN_POINT ( 'NONE',  ( 7.930394353207000258, -3.164807285701999984, 9.104732190648000767 ) ) ;
#15213=DIRECTION ( 'NONE',  ( 0.000000000000000000, -1.000000000000000000, 0.000000000000000000 ) ) ;
#15220=DIRECTION ( 'NONE',  ( 1.000000000000000000, 0.000000000000000000, 0.000000000000000000 ) ) ;
#15224=CARTESIAN_POINT ( 'NONE',  ( 9.629020610622001541, -5.794331084664000819, 7.414872097535999629 ) ) ;
#15230=CARTESIAN_POINT ( 'NONE',  ( 10.98956486188259341, -5.568313880529865756, -4.946129200245233726 ) ) ;
#15242=CARTESIAN_POINT ( 'NONE',  ( 7.696680409794002919, -4.865376733307997803, 6.399695646141002392 ) ) ;
#15243=B_SPLINE_CURVE_WITH_KNOTS ( 'NONE', 3,
 ( #45986, #61718, #56135, #13837 ),
 .UNSPECIFIED., .F., .F.,
 ( 4, 4 ),
 ( 0.000000000000000000, 1.000000000000000000 ),
 .UNSPECIFIED. ) ;
#15247=EDGE_CURVE ( 'NONE', #11010, #15130, #47751, .T. ) ;
#15254=LINE ( 'NONE', #550, #46205 ) ;
#15260=CARTESIAN_POINT ( 'NONE',  ( 9.234504440379000201, -5.964711531933999389, 7.776478361891000723 ) ) ;
#15264=DIRECTION ( 'NONE',  ( 0.000000000000000000, 0.000000000000000000, -1.000000000000000000 ) ) ;
#15273=CARTESIAN_POINT ( 'NONE',  ( 8.636456853209999451, -3.869396851328000153, 5.695656592546999519 ) ) ;
#15274=CARTESIAN_POINT ( 'NONE',  ( 8.475644353210000759, -5.095088356574999366, 6.286978111459999852 ) ) ;
#15280=VECTOR ( 'NONE', #55218, 1000.000000000000000 ) ;
#15290=ORIENTED_EDGE ( 'NONE', *, *, #3351, .T. ) ;
#15291=CARTESIAN_POINT ( 'NONE',  ( 11.09999999999999964, -5.449702618175999547, 5.124965750789000296 ) ) ;
#15293=CARTESIAN_POINT ( 'NONE',  ( 8.288447824096289551, -4.754611573949904191, 9.066990413095210144 ) ) ;
#15303=CARTESIAN_POINT ( 'NONE',  ( 7.726789014911999764, -2.853537667309000270, 6.781794374791000557 ) ) ;
#15313=ORIENTED_EDGE ( 'NONE', *, *, #69149, .F. ) ;
#15333=CARTESIAN_POINT ( 'NONE',  ( 10.64447714202000128, -5.073836261934999925, -8.340686666652999293 ) ) ;
#15338=B_SPLINE_CURVE_WITH_KNOTS ( 'NONE', 3,
 ( #68945, #42040, #63346, #47634 ),
 .UNSPECIFIED., .F., .F.,
 ( 4, 4 ),
 ( 0.8745081996710677430, 1.000000000000000000 ),
 .UNSPECIFIED. ) ;
#15355=EDGE_CURVE ( 'NONE', #8263, #39811, #48635, .T. ) ;
#15373=CARTESIAN_POINT ( 'NONE',  ( 11.09392659058396724, -2.706073409412732111, 6.603326177236545469 ) ) ;
#15374=CARTESIAN_POINT ( 'NONE',  ( 8.796581853210000190, -2.368260286481999710, 7.410200011629000549 ) ) ;
#15379=CARTESIAN_POINT ( 'NONE',  ( 10.20448674122262211, -2.648429362731085757, 7.853061647121137412 ) ) ;
#15381=CARTESIAN_POINT ( 'NONE',  ( 7.485254293485687604, -2.429645980366736957, 6.751440798236062690 ) ) ;
#15385=ORIENTED_EDGE ( 'NONE', *, *, #22188, .F. ) ;
#15402=CARTESIAN_POINT ( 'NONE',  ( 10.37902717885611636, -2.650237472149363338, -7.263327126957014990 ) ) ;
#15411=CARTESIAN_POINT ( 'NONE',  ( 9.889844610056000462, -4.052276314598000084, 9.260527932809999641 ) ) ;
#15424=CARTESIAN_POINT ( 'NONE',  ( 9.353731048338000065, -2.823575173856999410, 9.032043499493001448 ) ) ;
#15431=CARTESIAN_POINT ( 'NONE',  ( 9.414314870535999802, -3.941041813398000304, 5.878346364186999295 ) ) ;
#15448=VECTOR ( 'NONE', #24237, 1000.000000000000114 ) ;
#15451=CARTESIAN_POINT ( 'NONE',  ( 10.25462442569999943, -2.860634389522000109, 6.604605425112000994 ) ) ;
#15469=CARTESIAN_POINT ( 'NONE',  ( 9.663906509039998483, -2.491831134779999957, -6.388915175267000812 ) ) ;
#15470=CARTESIAN_POINT ( 'NONE',  ( 10.60770805961999841, -2.392337812398999564, -6.587351599745000286 ) ) ;
#15482=DIRECTION ( 'NONE',  ( 0.000000000000000000, -0.8648648648648717963, 0.5020047465136829867 ) ) ;
#15501=EDGE_CURVE ( 'NONE', #4646, #12348, #37588, .T. ) ;
#15514=CARTESIAN_POINT ( 'NONE',  ( 10.05525937050999907, -5.223866772223000332, -6.898311956607000361 ) ) ;
#15528=CARTESIAN_POINT ( 'NONE',  ( 10.35303240674999969, -3.419511749372000420, -4.861886959447999423 ) ) ;
#15529=EDGE_CURVE ( 'NONE', #64582, #52126, #33225, .T. ) ;
#15534=CARTESIAN_POINT ( 'NONE',  ( 9.566960887370999700, -5.215923019114000247, 6.177729435798999802 ) ) ;
#15543=CARTESIAN_POINT ( 'NONE',  ( 7.744301838472999577, -3.130384865731000055, 6.467396727560999814 ) ) ;
#15549=CARTESIAN_POINT ( 'NONE',  ( 11.09999999999999964, -2.649999999999999911, 7.500000000000000000 ) ) ;
#15550=ORIENTED_EDGE ( 'NONE', *, *, #8958, .T. ) ;
#15562=CARTESIAN_POINT ( 'NONE',  ( 10.11260824411999870, -3.359889198679999911, 5.859131457670000209 ) ) ;
#15564=CARTESIAN_POINT ( 'NONE',  ( 11.03879883359000047, -2.753595124514999881, 5.027017047203000466 ) ) ;
#15565=CARTESIAN_POINT ( 'NONE',  ( 7.839808059622000336, -3.084082018960999871, 9.259837032825000591 ) ) ;
#15572=ORIENTED_EDGE ( 'NONE', *, *, #7426, .F. ) ;
#15573=CARTESIAN_POINT ( 'NONE',  ( 9.815199780373001559, -2.813634733202999616, 8.848854270764999086 ) ) ;
#15576=ORIENTED_EDGE ( 'NONE', *, *, #21563, .F. ) ;
#15577=CARTESIAN_POINT ( 'NONE',  ( 10.98768472633000037, -6.720753151621999599, -5.471698430863999540 ) ) ;
#15581=DIRECTION ( 'NONE',  ( -1.000000000000000000, 0.000000000000000000, 0.000000000000000000 ) ) ;
#15583=DIRECTION ( 'NONE',  ( 0.000000000000000000, -1.000000000000000000, 0.000000000000000000 ) ) ;
#15594=DIRECTION ( 'NONE',  ( -0.1218403629891999795, -1.031102291695999760E-07, 0.9925497095595008368 ) ) ;
#15603=CARTESIAN_POINT ( 'NONE',  ( 8.052730646792999991, -4.968144979409999884, 5.971795951526999602 ) ) ;
#15616=CARTESIAN_POINT ( 'NONE',  ( 7.583058059622000080, -4.763531818439999732, 5.668890958491999754 ) ) ;
#15620=LINE ( 'NONE', #21886, #36750 ) ;
#15625=VERTEX_POINT ( 'NONE', #18906 ) ;
#15629=CARTESIAN_POINT ( 'NONE',  ( 7.152687255306670266, -3.171513860283114994, 8.579150755730465150 ) ) ;
#15631=ORIENTED_EDGE ( 'NONE', *, *, #23684, .T. ) ;
#15634=CARTESIAN_POINT ( 'NONE',  ( 8.229919888127584571, -5.613417466181594762, 8.151383774938032900 ) ) ;
#15643=CARTESIAN_POINT ( 'NONE',  ( 7.744883055160999952, -2.855944972365000112, 6.776570926616000357 ) ) ;
#15644=CARTESIAN_POINT ( 'NONE',  ( 8.470944094208999076, -5.100000000000000533, 6.571291218949999902 ) ) ;
#15647=CARTESIAN_POINT ( 'NONE',  ( 8.801828814214612606, -4.497542371825409724, 9.205821706225451706 ) ) ;
#15654=CARTESIAN_POINT ( 'NONE',  ( 9.085769353209000698, -2.821866379289000193, 6.127148604720000336 ) ) ;
#15659=ADVANCED_FACE ( 'NONE', ( #40231 ), #30708, .T. ) ;
#15680=CARTESIAN_POINT ( 'NONE',  ( 10.39191562140000080, -4.919949601728999866, -4.654593006246000364 ) ) ;
#15687=B_SPLINE_CURVE_WITH_KNOTS ( 'NONE', 3,
 ( #32154, #20620, #15030, #53123, #5224, #4526, #25862, #68497, #15379, #58027 ),
 .UNSPECIFIED., .F., .F.,
 ( 4, 2, 2, 2, 4 ),
 ( 0.1254469995254103021, 0.3127557518398033087, 0.5000645041541962321, 0.6873732564685889335, 0.8746820087829817458 ),
 .UNSPECIFIED. ) ;
#15706=CARTESIAN_POINT ( 'NONE',  ( 9.332537864288001472, -2.899999999999999911, 6.571291218949999902 ) ) ;
#15716=CARTESIAN_POINT ( 'NONE',  ( 7.422245559621999611, -5.361050935357000391, 6.973449182446000094 ) ) ;
#15723=CARTESIAN_POINT ( 'NONE',  ( 7.482900004268410399, -2.407370889025786997, 6.799601156578478189 ) ) ;
#15741=CARTESIAN_POINT ( 'NONE',  ( 8.803927344482000095, -5.129996464381000543, -6.743586268849999676 ) ) ;
#15750=CARTESIAN_POINT ( 'NONE',  ( 9.743567407955000093, -5.287392049455999832, 8.939957179821000466 ) ) ;
#15756=ORIENTED_EDGE ( 'NONE', *, *, #28063, .T. ) ;
#15760=DIRECTION ( 'NONE',  ( -0.7071067718169923300, -0.7071067905560921574, -1.210975589615986548E-07 ) ) ;
#15766=VERTEX_POINT ( 'NONE', #45391 ) ;
#15770=CARTESIAN_POINT ( 'NONE',  ( 10.62698276521000196, -3.142914536759000121, 8.668455626664998803 ) ) ;
#15774=CARTESIAN_POINT ( 'NONE',  ( 7.739033623444901089, -2.652152912377775174, 7.263328590673341800 ) ) ;
#15795=ORIENTED_EDGE ( 'NONE', *, *, #12892, .F. ) ;
#15799=CARTESIAN_POINT ( 'NONE',  ( 9.679514975094384965, -4.176630006209533619, -8.850146613061715684 ) ) ;
#15801=EDGE_CURVE ( 'NONE', #53841, #11010, #13921, .T. ) ;
#15805=CARTESIAN_POINT ( 'NONE',  ( 10.86330120046000047, -2.934641216426999932, -5.167266016126999872 ) ) ;
#15806=CARTESIAN_POINT ( 'NONE',  ( 10.49412055961999890, -2.866949708568999888, -8.960719633954001395 ) ) ;
#15810=CYLINDRICAL_SURFACE ( 'NONE', #10854, 0.4999999999999998335 ) ;
#15825=CARTESIAN_POINT ( 'NONE',  ( 7.000000000000000000, -7.526486366024999874, -3.526486366024999874 ) ) ;
#15847=CARTESIAN_POINT ( 'NONE',  ( 10.53865751177000121, -3.647233463439000012, -6.014125921456000334 ) ) ;
#15851=CARTESIAN_POINT ( 'NONE',  ( 5.700000000000000178, -1.300000000000000044, -9.662944685757000940 ) ) ;
#15860=CARTESIAN_POINT ( 'NONE',  ( 8.500486250726996929, -2.902641158998001458, 6.605591905707999700 ) ) ;
#15863=CARTESIAN_POINT ( 'NONE',  ( 7.790168786842999182, -2.923571394339999685, 6.474157094959999803 ) ) ;
#15865=DIRECTION ( 'NONE',  ( 0.000000000000000000, 0.000000000000000000, -1.000000000000000000 ) ) ;
#15866=CARTESIAN_POINT ( 'NONE',  ( 9.285188841453999586, -5.269672295101000437, 8.747824102203999530 ) ) ;
#15883=EDGE_LOOP ( 'NONE', ( #22172, #2589, #7008, #68335, #8947 ) ) ;
#15887=DIRECTION ( 'NONE',  ( -0.7071067783004970631, -0.7071067840725973053, 3.040673725924991281E-08 ) ) ;
#15893=CARTESIAN_POINT ( 'NONE',  ( 10.46754921866999943, -2.318350880468999620, 6.549783596838000044 ) ) ;
#15897=CARTESIAN_POINT ( 'NONE',  ( 9.214144353209000826, -5.421531391267000011, 6.381128921159999301 ) ) ;
#15902=DIRECTION ( 'NONE',  ( 1.000000000000000000, 0.000000000000000000, 0.000000000000000000 ) ) ;
#15904=VERTEX_POINT ( 'NONE', #56562 ) ;
#15905=CARTESIAN_POINT ( 'NONE',  ( 9.352255147285999826, -2.817754448466000206, 6.388456890282999900 ) ) ;
#15909=CARTESIAN_POINT ( 'NONE',  ( 7.307500000000000107, -0.2999999999999999889, -3.149999999999999911 ) ) ;
#15910=ORIENTED_EDGE ( 'NONE', *, *, #40021, .F. ) ;
#15922=CARTESIAN_POINT ( 'NONE',  ( 8.361422056298998484, -5.126342729456004221, 6.365321850284000327 ) ) ;
#15932=CARTESIAN_POINT ( 'NONE',  ( 8.938868730821853958, -3.795034549399585178, -6.149945561018825835 ) ) ;
#15934=CARTESIAN_POINT ( 'NONE',  ( 8.725348536223782148, -2.649439212887072959, 7.500023728975150128 ) ) ;
#15939=EDGE_CURVE ( 'NONE', #67742, #2068, #1825, .T. ) ;
#15941=CARTESIAN_POINT ( 'NONE',  ( 8.694605646795000808, -5.290204991635000020, 8.768102264518001121 ) ) ;
#15944=COLOUR_RGB ( '', 0.08235294, 0.09019608, 0.10196078) ;
#15947=CARTESIAN_POINT ( 'NONE',  ( 10.61094409420999973, -5.100000000000000533, -6.571291218949999902 ) ) ;
#15953=CARTESIAN_POINT ( 'NONE',  ( 9.176355646795000709, -2.935738482289000029, 6.259841087764999479 ) ) ;
#15955=PLANE ( 'NONE',  #309 ) ;
#15956=CARTESIAN_POINT ( 'NONE',  ( 9.123929153134323400, -5.099761357576727328, 6.165062780802330167 ) ) ;
#15959=EDGE_CURVE ( 'NONE', #15130, #62127, #14940, .T. ) ;
#15969=CARTESIAN_POINT ( 'NONE',  ( 7.835751895984281568, -4.956109399768123147, 6.487758672992816500 ) ) ;
#15972=CARTESIAN_POINT ( 'NONE',  ( 8.493055160192083619, -2.517084544257638612, 6.576072328180241122 ) ) ;
#15975=AXIS2_PLACEMENT_3D ( 'NONE', #16809, #26972, #31528 ) ;
#15988=ORIENTED_EDGE ( 'NONE', *, *, #9398, .F. ) ;
#15992=CARTESIAN_POINT ( 'NONE',  ( 9.214144353209000826, -5.421531391267000011, 6.381128921159999301 ) ) ;
#16012=LINE ( 'NONE', #58318, #21582 ) ;
#16031=VERTEX_POINT ( 'NONE', #44969 ) ;
#16038=ORIENTED_EDGE ( 'NONE', *, *, #56664, .T. ) ;
#16044=CARTESIAN_POINT ( 'NONE',  ( 9.771640687501500722, -2.873222873813889411, 6.752018918873273989 ) ) ;
#16050=CARTESIAN_POINT ( 'NONE',  ( 10.34947173981000113, -4.457565973839000328, 6.154866550070000386 ) ) ;
#16051=CARTESIAN_POINT ( 'NONE',  ( 8.887168146795000112, -2.193670085072000120, 7.400591740205000768 ) ) ;
#16056=CARTESIAN_POINT ( 'NONE',  ( 10.48598064679000075, -5.506038521567000465, -7.274786670944999756 ) ) ;
#16057=CARTESIAN_POINT ( 'NONE',  ( 7.759089400014850035, -5.269491846164327420, 8.691428595288718029 ) ) ;
#16064=EDGE_LOOP ( 'NONE', ( #57785, #25209, #14007, #33744 ) ) ;
#16074=B_SPLINE_CURVE_WITH_KNOTS ( 'NONE', 3,
 ( #17496, #38820, #65724, #17848, #23771 ),
 .UNSPECIFIED., .F., .F.,
 ( 4, 1, 4 ),
 ( 0.000000000000000000, 0.5000000000000000000, 1.000000000000000000 ),
 .UNSPECIFIED. ) ;
#16083=CARTESIAN_POINT ( 'NONE',  ( 10.61382642076999971, -3.385081736013999976, 5.849525238167000651 ) ) ;
#16084=EDGE_CURVE ( 'NONE', #16031, #15625, #17683, .T. ) ;
#16096=DIRECTION ( 'NONE',  ( 8.759270281372000635E-11, -8.759291270753999297E-11, 1.000000000000000000 ) ) ;
#16101=CARTESIAN_POINT ( 'NONE',  ( 9.241224735070849405, -2.676616289842693952, 7.234190499188664525 ) ) ;
#16103=EDGE_LOOP ( 'NONE', ( #49521, #51974, #47827, #9970, #44310 ) ) ;
#16108=ADVANCED_FACE ( 'NONE', ( #37213 ), #25343, .T. ) ;
#16109=CARTESIAN_POINT ( 'NONE',  ( 10.19256470245000123, -2.560274838243000062, 7.664550593243999899 ) ) ;
#16128=FACE_OUTER_BOUND ( 'NONE', #19614, .T. ) ;
#16130=EDGE_CURVE ( 'NONE', #46269, #48331, #27712, .T. ) ;
#16148=CARTESIAN_POINT ( 'NONE',  ( 10.50898185320999900, -4.485028460808000439, -9.114431591966999591 ) ) ;
#16152=CARTESIAN_POINT ( 'NONE',  ( 9.050000000000000711, 0.000000000000000000, 4.000000000000000000 ) ) ;
#16167=CARTESIAN_POINT ( 'NONE',  ( 7.000000000000000000, -6.495985883990673670, -3.000000000000000000 ) ) ;
#16170=EDGE_CURVE ( 'NONE', #33857, #23094, #47949, .T. ) ;
#16173=EDGE_LOOP ( 'NONE', ( #5504, #52610, #28554 ) ) ;
#16178=( GEOMETRIC_REPRESENTATION_CONTEXT ( 3 ) GLOBAL_UNCERTAINTY_ASSIGNED_CONTEXT ( ( #60254 ) ) GLOBAL_UNIT_ASSIGNED_CONTEXT ( ( #45434, #61508, #8373 ) ) REPRESENTATION_CONTEXT ( 'NONE', 'WORKASPACE' ) );
#16179=CARTESIAN_POINT ( 'NONE',  ( 10.58522900337914052, -2.975308710305338167, 5.037100615727592157 ) ) ;
#16193=CARTESIAN_POINT ( 'NONE',  ( 10.14584566409999944, -5.370505908760000224, -6.826219946961000318 ) ) ;
#16207=CARTESIAN_POINT ( 'NONE',  ( 9.719606904206999687, -5.967761543230999166, 7.406644089178000101 ) ) ;
#16210=CARTESIAN_POINT ( 'NONE',  ( 9.753140057121997941, -4.104977100659999323, 9.293279163877999238 ) ) ;
#16213=CARTESIAN_POINT ( 'NONE',  ( 9.731876262297951996, -2.899999999999999911, -6.324732395500358706 ) ) ;
#16218=B_SPLINE_SURFACE_WITH_KNOTS ( 'NONE', 3, 3, ( 
 ( #57078, #41350, #3926, #47285 ),
 ( #62661, #30518, #36100, #9520 ),
 ( #21055, #62994, #30862, #63690 ),
 ( #15122, #36443, #9871, #15805 ),
 ( #57760, #31215, #20709, #38153 ) ),
 .UNSPECIFIED., .F., .F., .F.,
 ( 4, 1, 4 ),
 ( 4, 4 ),
 ( 0.9643675639056999982, 1.000000000000000000, 1.004735132284999999 ),
 ( -0.1730180444169999998, 1.173018043257999965 ),
 .UNSPECIFIED. ) ;
#16225=CARTESIAN_POINT ( 'NONE',  ( 10.26811392801000089, -4.000000000000000000, 4.767677575776000154 ) ) ;
#16236=CARTESIAN_POINT ( 'NONE',  ( 9.632185590920999019, -5.638162562978999759, 6.476633609657000079 ) ) ;
#16239=CARTESIAN_POINT ( 'NONE',  ( 6.992194708760999688, -9.194551129401000722, 5.189166568983999639 ) ) ;
#16240=CARTESIAN_POINT ( 'NONE',  ( 7.775620559622000272, -4.636725880537000855, 9.378965771357000492 ) ) ;
#16247=CARTESIAN_POINT ( 'NONE',  ( 8.154750263806279875, -3.054975986857539016, 6.324465894181788173 ) ) ;
#16249=CARTESIAN_POINT ( 'NONE',  ( 9.166075977534999808, -4.023333687735000552, 9.122281080215000060 ) ) ;
#16256=CARTESIAN_POINT ( 'NONE',  ( 10.61442944038000036, -5.287639274524000399, -7.937245019889999753 ) ) ;
#16257=ORIENTED_EDGE ( 'NONE', *, *, #25874, .T. ) ;
#16267=CARTESIAN_POINT ( 'NONE',  ( 9.629471092178999214, -5.100000000000000533, 6.152188490330000370 ) ) ;
#16275=EDGE_CURVE ( 'NONE', #29023, #42061, #21136, .T. ) ;
#16279=CARTESIAN_POINT ( 'NONE',  ( 9.291454852466372927, -5.435482730291879783, -6.499550932516991786 ) ) ;
#16284=CARTESIAN_POINT ( 'NONE',  ( 7.539230646792000279, -4.696237245142999228, 5.830277424166999900 ) ) ;
#16296=CARTESIAN_POINT ( 'NONE',  ( 9.149956853208999874, -4.175914961544999748, 5.699510287082000026 ) ) ;
#16297=CARTESIAN_POINT ( 'NONE',  ( 8.513433059625000965, -5.040796345420999636, 8.522966281393001609 ) ) ;
#16298=CARTESIAN_POINT ( 'NONE',  ( 7.716851002542999716, -2.832432432432000269, 6.822293592207000934 ) ) ;
#16310=CARTESIAN_POINT ( 'NONE',  ( 7.955097046864369581, -4.953350247991573418, 6.431944445602010063 ) ) ;
#16315=CARTESIAN_POINT ( 'NONE',  ( 8.554703854670005825, -3.570844187153873417, 5.814174462132309706 ) ) ;
#16317=EDGE_LOOP ( 'NONE', ( #24858, #36537, #60978, #31920, #24563 ) ) ;
#16320=ORIENTED_EDGE ( 'NONE', *, *, #55932, .T. ) ;
#16322=CARTESIAN_POINT ( 'NONE',  ( 7.721047324851166849, -2.916517839021724789, 6.666908917546550128 ) ) ;
#16325=VERTEX_POINT ( 'NONE', #37897 ) ;
#16327=CARTESIAN_POINT ( 'NONE',  ( 9.715118312915786092, -4.417515367316165786, -8.786662241963096420 ) ) ;
#16356=ADVANCED_FACE ( 'NONE', ( #43145 ), #64446, .T. ) ;
#16357=CARTESIAN_POINT ( 'NONE',  ( 10.56591477248000110, -5.293237054095000005, -7.067083954277999958 ) ) ;
#16362=CARTESIAN_POINT ( 'NONE',  ( 10.98768472639999949, -0.3876847264043000174, -4.945212061661000469 ) ) ;
#16365=B_SPLINE_CURVE_WITH_KNOTS ( 'NONE', 3,
 ( #63345, #57762, #4972, #9873, #47633, #41690, #31217, #51833, #25266, #19331 ),
 .UNSPECIFIED., .F., .F.,
 ( 4, 2, 2, 2, 4 ),
 ( 0.1254223444949154886, 0.3127174981214190796, 0.5000126517479226429, 0.6873078053744264837, 0.8746029590009303245 ),
 .UNSPECIFIED. ) ;
#16367=CARTESIAN_POINT ( 'NONE',  ( 10.83253786428999987, -2.899999999999999911, 6.571291218949999902 ) ) ;
#16369=VECTOR ( 'NONE', #68006, 1000.000000000000114 ) ;
#16390=ADVANCED_FACE ( 'NONE', ( #6767 ), #20094, .F. ) ;
#16395=CARTESIAN_POINT ( 'NONE',  ( 10.76010362286999822, -4.535387425205000156, 6.001717576299999024 ) ) ;
#16396=CARTESIAN_POINT ( 'NONE',  ( 7.101308059622001068, -3.554853390786000045, 8.889491623367000273 ) ) ;
#16397=ORIENTED_EDGE ( 'NONE', *, *, #35075, .T. ) ;
#16400=CARTESIAN_POINT ( 'NONE',  ( 10.20608185320999972, -2.622355301673999772, -6.528538675937999969 ) ) ;
#16401=CARTESIAN_POINT ( 'NONE',  ( 7.754742686019933551, -5.333685489479075947, 8.616430321029321604 ) ) ;
#16402=CARTESIAN_POINT ( 'NONE',  ( 9.657547180956999711, -5.333447643521000536, 6.049925825719999928 ) ) ;
#16419=CARTESIAN_POINT ( 'NONE',  ( 8.304129440378000382, -3.650411072918999800, 6.083135626079000602 ) ) ;
#16427=CARTESIAN_POINT ( 'NONE',  ( 10.72520823780999955, -5.521647200017000934, 6.612992938078999572 ) ) ;
#16435=DIRECTION ( 'NONE',  ( 1.000000000000000000, 0.000000000000000000, 0.000000000000000000 ) ) ;
#16448=CARTESIAN_POINT ( 'NONE',  ( 9.449618669012016525, -4.457228036536642790, 8.907268959278543008 ) ) ;
#16479=ADVANCED_FACE ( 'NONE', ( #25953 ), #58452, .F. ) ;
#16481=CARTESIAN_POINT ( 'NONE',  ( 9.674960421382822418, -2.650268802167429438, 7.499999178247414910 ) ) ;
#16490=CARTESIAN_POINT ( 'NONE',  ( 10.35753185321000025, -5.367809014988999650, -6.514738374536999999 ) ) ;
#16505=CARTESIAN_POINT ( 'NONE',  ( 10.34920446231350155, -2.899999999999999911, -6.662590550579927218 ) ) ;
#16510=CARTESIAN_POINT ( 'NONE',  ( 10.56591477248000110, -5.293237054095000005, -7.067083954277999958 ) ) ;
#16524=CARTESIAN_POINT ( 'NONE',  ( 9.903944471677000649, -5.205019707614999547, 6.747219600580999455 ) ) ;
#16525=ADVANCED_FACE ( 'NONE', ( #26653 ), #16218, .F. ) ;
#16529=ORIENTED_EDGE ( 'NONE', *, *, #956, .T. ) ;
#16537=CARTESIAN_POINT ( 'NONE',  ( 10.16989351219999982, -2.594225604561000154, -6.291264536816999708 ) ) ;
#16543=CARTESIAN_POINT ( 'NONE',  ( 8.587675602096970451, -2.935917077764118144, 6.277144180784712368 ) ) ;
#16549=CARTESIAN_POINT ( 'NONE',  ( 8.164796825344000197, -3.457406484157000026, 6.165651553258999940 ) ) ;
#16552=LINE ( 'NONE', #9666, #64576 ) ;
#16553=CARTESIAN_POINT ( 'NONE',  ( 7.491953176340000908, -3.528027000165000704, 6.607934030033999484 ) ) ;
#16557=CARTESIAN_POINT ( 'NONE',  ( 9.691080333872001518, -5.335644368206000188, 8.701217921043999937 ) ) ;
#16560=EDGE_CURVE ( 'NONE', #22542, #51145, #44119, .T. ) ;
#16568=CARTESIAN_POINT ( 'NONE',  ( 11.09999999999999964, -2.700000000000000178, 5.160242730440000258 ) ) ;
#16583=EDGE_LOOP ( 'NONE', ( #41695, #10802, #60446, #31797, #53479, #6258 ) ) ;
#16584=CARTESIAN_POINT ( 'NONE',  ( 10.05691733561000056, -2.453480799114999833, 6.657106310117000270 ) ) ;
#16597=CARTESIAN_POINT ( 'NONE',  ( 10.80815535238000002, -2.937528991339000140, 8.948455587554001056 ) ) ;
#16613=ORIENTED_EDGE ( 'NONE', *, *, #63198, .F. ) ;
#16616=DIRECTION ( 'NONE',  ( 1.000000000000000000, 0.000000000000000000, 0.000000000000000000 ) ) ;
#16619=CARTESIAN_POINT ( 'NONE',  ( 9.781666627457001439, -5.464740618746000145, 8.817321229216000589 ) ) ;
#16623=VERTEX_POINT ( 'NONE', #11935 ) ;
#16627=CARTESIAN_POINT ( 'NONE',  ( 7.225322421146570306, -2.650264760010439868, 7.500018091723870128 ) ) ;
#16629=CARTESIAN_POINT ( 'NONE',  ( 7.603418146792000343, -5.687202994508999687, 6.847270485579000088 ) ) ;
#16633=DIRECTION ( 'NONE',  ( 0.000000000000000000, -0.8648648648648717963, 0.5020047465136829867 ) ) ;
#16634=DIRECTION ( 'NONE',  ( -1.000000000000000000, 0.000000000000000000, 0.000000000000000000 ) ) ;
#16640=CARTESIAN_POINT ( 'NONE',  ( 8.727043146794999373, -3.882020254083999866, 5.870054788755000530 ) ) ;
#16659=CARTESIAN_POINT ( 'NONE',  ( 8.304386322453103375, -4.439452195556469860, 9.191388126121186275 ) ) ;
#16661=VERTEX_POINT ( 'NONE', #32247 ) ;
#16664=VERTEX_POINT ( 'NONE', #33622 ) ;
#16665=EDGE_CURVE ( 'NONE', #51145, #12348, #42722, .T. ) ;
#16667=CARTESIAN_POINT ( 'NONE',  ( 7.744301838472999577, -3.130384865731000055, 6.467396727560999814 ) ) ;
#16684=DIRECTION ( 'NONE',  ( 0.000000000000000000, 1.000000000000000000, 0.000000000000000000 ) ) ;
#16698=PRODUCT_DEFINITION ( 'UNKNOWN', '', #24024, #35999 ) ;
#16712=CARTESIAN_POINT ( 'NONE',  ( 7.000000000000000000, 0.5292307692307999245, 2.083846153846000249 ) ) ;
#16713=VERTEX_POINT ( 'NONE', #10902 ) ;
#16715=CARTESIAN_POINT ( 'NONE',  ( 7.550000000000000711, -4.000000000000000000, 8.849999999999999645 ) ) ;
#16733=CARTESIAN_POINT ( 'NONE',  ( 10.01532628870999986, -4.946995631616999844, 8.559221361189001342 ) ) ;
#16738=CARTESIAN_POINT ( 'NONE',  ( 10.84974435320999930, -5.265000209383999596, -6.385811305909999902 ) ) ;
#16740=CARTESIAN_POINT ( 'NONE',  ( 7.807002133442725089, -4.386469107892202679, 9.196132381460992988 ) ) ;
#16741=CARTESIAN_POINT ( 'NONE',  ( 9.305875415870998424, -4.945293979885000191, 9.077881967919999795 ) ) ;
#16743=VERTEX_POINT ( 'NONE', #59480 ) ;
#16756=FACE_OUTER_BOUND ( 'NONE', #33145, .T. ) ;
#16764=CARTESIAN_POINT ( 'NONE',  ( 7.986083034292184912, -5.349307872168665767, 7.676713696079082716 ) ) ;
#16774=LINE ( 'NONE', #49638, #53771 ) ;
#16775=AXIS2_PLACEMENT_3D ( 'NONE', #67941, #9210, #3622 ) ;
#16777=EDGE_CURVE ( 'NONE', #52199, #33729, #47776, .T. ) ;
#16779=EDGE_CURVE ( 'NONE', #28326, #23313, #43506, .T. ) ;
#16800=EDGE_CURVE ( 'NONE', #61758, #26679, #41075, .T. ) ;
#16808=B_SPLINE_CURVE_WITH_KNOTS ( 'NONE', 3,
 ( #3242, #8145, #51477, #39971 ),
 .UNSPECIFIED., .F., .F.,
 ( 4, 4 ),
 ( 0.6941835283959838510, 1.000000000000000000 ),
 .UNSPECIFIED. ) ;
#16809=CARTESIAN_POINT ( 'NONE',  ( 11.09999999999999964, -4.000000000000000000, 7.500000000000000000 ) ) ;
#16814=CARTESIAN_POINT ( 'NONE',  ( 9.470944094206000585, -5.100000000000000533, 6.571291218949999902 ) ) ;
#16818=B_SPLINE_CURVE_WITH_KNOTS ( 'NONE', 3,
 ( #59609, #55409, #54712, #7501, #2267, #22202, #18351, #28148, #39674, #16951, #60993, #13113 ),
 .UNSPECIFIED., .F., .F.,
 ( 4, 2, 2, 2, 2, 4 ),
 ( 0.000000000000000000, 0.2499999999999970579, 0.3749999999999958922, 0.4999999999999947820, 0.7499999999999973355, 1.000000000000000000 ),
 .UNSPECIFIED. ) ;
#16820=DIRECTION ( 'NONE',  ( 0.000000000000000000, 1.000000000000000000, 0.000000000000000000 ) ) ;
#16823=EDGE_CURVE ( 'NONE', #29320, #15110, #50246, .T. ) ;
#16828=AXIS2_PLACEMENT_3D ( 'NONE', #33419, #54036, #16633 ) ;
#16830=CARTESIAN_POINT ( 'NONE',  ( 10.44811814679000150, -5.235603901491000300, -6.609968500665999613 ) ) ;
#16852=CARTESIAN_POINT ( 'NONE',  ( 9.870877370727999534, -2.904359058094999835, -8.563874348197000330 ) ) ;
#16878=CARTESIAN_POINT ( 'NONE',  ( 10.48414299032999963, -4.098653366703000067, -9.351353705206001621 ) ) ;
#16893=CARTESIAN_POINT ( 'NONE',  ( 7.559219638201004621, -3.224407481241000628, 6.403792276147000528 ) ) ;
#16896=CARTESIAN_POINT ( 'NONE',  ( 10.06844525594999951, -4.148609764890999863, 8.941457795715999524 ) ) ;
#16907=CARTESIAN_POINT ( 'NONE',  ( 8.199995110659001440, -2.894508759333000114, 6.645190873281999089 ) ) ;
#16922=CARTESIAN_POINT ( 'NONE',  ( 9.251933059621999078, -5.159251056493999954, 9.109488373271000583 ) ) ;
#16932=CARTESIAN_POINT ( 'NONE',  ( 9.261668853699999815, -2.944250413017999612, 6.507387951280999339 ) ) ;
#16937=CARTESIAN_POINT ( 'NONE',  ( 10.19794194037999979, -4.262172867567000090, -8.834326937932999613 ) ) ;
#16949=CARTESIAN_POINT ( 'NONE',  ( 9.334238628924479642, -3.792635205665601195, 9.233780771583109725 ) ) ;
#16951=CARTESIAN_POINT ( 'NONE',  ( 8.307734559752500303, -5.093561253831357938, 6.540208455084596473 ) ) ;
#16955=CARTESIAN_POINT ( 'NONE',  ( 9.194602547868999665, -5.157768569202000108, 8.637845986715998237 ) ) ;
#16963=CARTESIAN_POINT ( 'NONE',  ( 10.81316193496000011, -3.756072284922999938, 6.071597915422999314 ) ) ;
#16967=CARTESIAN_POINT ( 'NONE',  ( 8.154706853209001238, -4.255646685191999623, 9.114089645792999406 ) ) ;
#16986=ADVANCED_FACE ( 'NONE', ( #21228 ), #68418, .F. ) ;
#17001=CARTESIAN_POINT ( 'NONE',  ( 8.390259216738563453, -2.723240919514677838, 8.682674612182450957 ) ) ;
#17007=VERTEX_POINT ( 'NONE', #10733 ) ;
#17012=CARTESIAN_POINT ( 'NONE',  ( 10.48121855676791903, -3.643715756357204683, -9.239801132892552005 ) ) ;
#17034=EDGE_CURVE ( 'NONE', #65121, #69025, #64327, .T. ) ;
#17042=CARTESIAN_POINT ( 'NONE',  ( 10.73506343560000076, -5.202499304193000107, -8.441414596927000247 ) ) ;
#17044=CARTESIAN_POINT ( 'NONE',  ( 8.883148997460001084, -5.167567567567999731, 6.822293592207000934 ) ) ;
#17045=CARTESIAN_POINT ( 'NONE',  ( 10.26947109217999810, -5.100000000000000533, -6.152188490330000370 ) ) ;
#17058=LINE ( 'NONE', #48890, #55619 ) ;
#17059=B_SPLINE_SURFACE_WITH_KNOTS ( 'NONE', 3, 3, ( 
 ( #55688, #50785, #7785, #29125, #39955, #7432, #28783, #13725, #17937, #39601, #39256, #60581, #33673, #60237, #8476, #18282, #23514, #28429, #24203 ),
 ( #50094, #35054, #12340, #18625, #2203, #1852, #60925, #12686, #18965, #40291, #44856, #19300, #23170, #51125, #13039, #3227, #44519, #34369, #2880 ),
 ( #2534, #65812, #34021, #23862, #55336, #66163, #66504, #13389, #34711, #45545, #56023, #66851, #10188, #68212, #67877, #9489, #68557, #41659, #46568 ),
 ( #62963, #3899, #31518, #62626, #14751, #4586, #57049, #14416, #9150, #15091, #47600, #52490, #20331, #36764, #58085, #46910, #14070, #35394, #36415 ) ),
 .UNSPECIFIED., .F., .F., .F.,
 ( 4, 4 ),
 ( 4, 1, 1, 1, 1, 1, 1, 1, 1, 1, 1, 1, 1, 1, 1, 1, 4 ),
 ( -0.1039086239011999951, 1.103908623900999864 ),
 ( -0.008849010032007000384, 0.01991027257200999809, 0.04866955517603999831, 0.07742883778006000306, 0.1061881203840999988, 0.1349474029881000126, 0.1637066855920999986, 0.1924659681960999846, 0.2212252508002000018, 0.2499845334042000156, 0.2787438160081999738, 0.3075030986121999876, 0.3362623812162000014, 0.3650216638202999908, 0.3937809464243000046, 0.4225402290282999629, 0.4512995116322999767 ),
 .UNSPECIFIED. ) ;
#17068=CARTESIAN_POINT ( 'NONE',  ( 10.64831157502426429, -4.679757719901565416, -8.679446014678198651 ) ) ;
#17073=ORIENTED_EDGE ( 'NONE', *, *, #37169, .T. ) ;
#17078=CARTESIAN_POINT ( 'NONE',  ( 9.442085454646999665, -4.742494605615999781, 8.809986937145000141 ) ) ;
#17083=CARTESIAN_POINT ( 'NONE',  ( 10.78888064679000003, -2.675723359162999859, -6.748225798259000818 ) ) ;
#17084=CARTESIAN_POINT ( 'NONE',  ( 7.898220110652619752, -2.603757854786413972, 8.536907500157953521 ) ) ;
#17086=CARTESIAN_POINT ( 'NONE',  ( 9.691080333872001518, -5.335644368206000188, 8.701217921043999937 ) ) ;
#17087=CYLINDRICAL_SURFACE ( 'NONE', #38785, 1.350000000000000089 ) ;
#17100=ORIENTED_EDGE ( 'NONE', *, *, #7679, .F. ) ;
#17104=CARTESIAN_POINT ( 'NONE',  ( 9.566483607044000692, -4.108965473266000146, 8.851626696081998702 ) ) ;
#17131=CARTESIAN_POINT ( 'NONE',  ( 9.957462135714001406, -5.100000000000000533, -6.571291218949999902 ) ) ;
#17137=CARTESIAN_POINT ( 'NONE',  ( 9.447848023450999833, -5.447470167531999863, 7.431328114251999573 ) ) ;
#17146=DIRECTION ( 'NONE',  ( -1.000000000000000000, 0.000000000000000000, 0.000000000000000000 ) ) ;
#17149=CARTESIAN_POINT ( 'NONE',  ( 11.09999999999999964, -5.299999999999999822, 5.160242713806000303 ) ) ;
#17154=VERTEX_POINT ( 'NONE', #34146 ) ;
#17166=CYLINDRICAL_SURFACE ( 'NONE', #24090, 1.350000000000000089 ) ;
#17176=B_SPLINE_CURVE_WITH_KNOTS ( 'NONE', 3,
 ( #35698, #3860, #34329, #18588, #51087, #18242, #39563, #13003, #55648, #50399 ),
 .UNSPECIFIED., .F., .F.,
 ( 4, 2, 2, 2, 4 ),
 ( 0.000000000000000000, 0.1477786706793876581, 0.2216680060190820700, 0.2586126736889285960, 0.2955573413587750942 ),
 .UNSPECIFIED. ) ;
#17178=CARTESIAN_POINT ( 'NONE',  ( 10.43325685320999874, -5.596199512734999715, -8.042023143828998855 ) ) ;
#17180=CARTESIAN_POINT ( 'NONE',  ( 9.617147628285000138, -2.491831134779999957, -6.388915175267000812 ) ) ;
#17185=CARTESIAN_POINT ( 'NONE',  ( 11.09999999999999964, -5.299999999999999822, 5.160242713806000303 ) ) ;
#17189=ORIENTED_EDGE ( 'NONE', *, *, #20354, .F. ) ;
#17194=CARTESIAN_POINT ( 'NONE',  ( 8.621524209948782769, -3.647212272540656830, 8.851469415033186294 ) ) ;
#17195=CARTESIAN_POINT ( 'NONE',  ( 7.307500000000000107, -0.2999999999999999889, -3.149999999999999911 ) ) ;
#17199=CARTESIAN_POINT ( 'NONE',  ( 10.39355669675000016, -4.089958462238000081, -9.188182957628999503 ) ) ;
#17218=CARTESIAN_POINT ( 'NONE',  ( 9.514108112060000622, -4.887639888682999256, 8.462756667353000140 ) ) ;
#17221=ORIENTED_EDGE ( 'NONE', *, *, #54974, .T. ) ;
#17231=CARTESIAN_POINT ( 'NONE',  ( 9.843620110012999191, -5.021680390140000227, -8.761463725090999688 ) ) ;
#17233=CARTESIAN_POINT ( 'NONE',  ( 9.564964385875493136, -5.350010280223940207, -7.500002129152480101 ) ) ;
#17234=CARTESIAN_POINT ( 'NONE',  ( 8.199995110659001440, -2.894508759333000114, 6.645190873281999089 ) ) ;
#17235=DIRECTION ( 'NONE',  ( 1.000000000000000000, -9.560371307181999538E-10, -1.449016008921000004E-09 ) ) ;
#17236=CARTESIAN_POINT ( 'NONE',  ( 8.629140486159279533, -3.010722422556198818, -6.580811551485690636 ) ) ;
#17243=CIRCLE ( 'NONE', #2723, 2.149999999999999911 ) ;
#17244=CARTESIAN_POINT ( 'NONE',  ( 9.406851002546000373, -2.832432432432000269, -6.822293592207000934 ) ) ;
#17247=CARTESIAN_POINT ( 'NONE',  ( 7.575821720216998401, -3.529668843644999221, 6.549222992663997545 ) ) ;
#17250=CARTESIAN_POINT ( 'NONE',  ( 11.11845396862999991, -5.767021056207999763, 7.178419201465000121 ) ) ;
#17258=FACE_OUTER_BOUND ( 'NONE', #25732, .T. ) ;
#17259=ADVANCED_FACE ( 'NONE', ( #61730 ), #11209, .T. ) ;
#17267=CARTESIAN_POINT ( 'NONE',  ( 7.725062132959652494, -2.650631715052233162, 7.500008390440855877 ) ) ;
#17278=ORIENTED_EDGE ( 'NONE', *, *, #65815, .F. ) ;
#17279=DIRECTION ( 'NONE',  ( 1.000000000000000000, 0.000000000000000000, 0.000000000000000000 ) ) ;
#17282=CARTESIAN_POINT ( 'NONE',  ( 7.975339216757299177, -5.350090185752664595, 7.499980949462679014 ) ) ;
#17286=CARTESIAN_POINT ( 'NONE',  ( 11.01666666666868188, -3.382745367834177230, 8.852578401490447391 ) ) ;
#17287=ORIENTED_EDGE ( 'NONE', *, *, #65698, .F. ) ;
#17288=CARTESIAN_POINT ( 'NONE',  ( 9.944325809452999820, -5.443013936195000291, 7.367349259341000156 ) ) ;
#17291=ORIENTED_EDGE ( 'NONE', *, *, #36782, .F. ) ;
#17292=LINE ( 'NONE', #15909, #8032 ) ;
#17293=CARTESIAN_POINT ( 'NONE',  ( 10.14521814679000045, -3.576528389491000048, -8.962725485696999783 ) ) ;
#17295=B_SPLINE_CURVE_WITH_KNOTS ( 'NONE', 3,
 ( #19316, #54397, #24909, #51144 ),
 .UNSPECIFIED., .F., .F.,
 ( 4, 4 ),
 ( 0.000000000000000000, 1.000000000000000000 ),
 .UNSPECIFIED. ) ;
#17300=VECTOR ( 'NONE', #2174, 1000.000000000000114 ) ;
#17305=CARTESIAN_POINT ( 'NONE',  ( 8.229954139086000708, -4.681838082657003852, 6.132216288069997745 ) ) ;
#17312=CARTESIAN_POINT ( 'NONE',  ( 9.318721994369999706, -2.755032632138999737, 8.795122807847999269 ) ) ;
#17323=CARTESIAN_POINT ( 'NONE',  ( 7.999933059623999476, -5.198566224659999513, 8.332559954171999905 ) ) ;
#17326=CARTESIAN_POINT ( 'NONE',  ( 11.07128162083999889, -6.555044467076000636, 5.493351806897000422 ) ) ;
#17328=FACE_OUTER_BOUND ( 'NONE', #53257, .T. ) ;
#17335=CARTESIAN_POINT ( 'NONE',  ( 8.930995559624999913, -2.019079883662000086, 7.390983468784999566 ) ) ;
#17344=VERTEX_POINT ( 'NONE', #59233 ) ;
#17352=ORIENTED_EDGE ( 'NONE', *, *, #54974, .F. ) ;
#17360=ORIENTED_EDGE ( 'NONE', *, *, #23607, .T. ) ;
#17362=CARTESIAN_POINT ( 'NONE',  ( 9.514108112060000622, -4.887639888682999256, 8.462756667353000140 ) ) ;
#17371=CARTESIAN_POINT ( 'NONE',  ( 8.953527735834686752, -2.251939686354768710, 7.420637145815573987 ) ) ;
#17377=VECTOR ( 'NONE', #43005, 1000.000000000000000 ) ;
#17394=CARTESIAN_POINT ( 'NONE',  ( 8.739649184022004746, -2.648220570447153310, 7.263719241076167954 ) ) ;
#17396=CARTESIAN_POINT ( 'NONE',  ( 10.97075054419999951, -2.648517896406999750, -6.788869136079999755 ) ) ;
#17399=CARTESIAN_POINT ( 'NONE',  ( 9.140753410162000492, -5.100000000000000533, 6.175944241622000064 ) ) ;
#17408=CARTESIAN_POINT ( 'NONE',  ( 10.06819717210663612, -5.125396288445600135, -6.749639981115930887 ) ) ;
#17418=CARTESIAN_POINT ( 'NONE',  ( 7.565629440376999248, -3.206365290996999740, 5.681739161071000410 ) ) ;
#17419=CARTESIAN_POINT ( 'NONE',  ( 9.355720302797999821, -5.362859773739999447, -6.470306978669999154 ) ) ;
#17421=CARTESIAN_POINT ( 'NONE',  ( 8.933148997457999840, -5.167567567567999731, 6.822293592207000934 ) ) ;
#17423=ORIENTED_EDGE ( 'NONE', *, *, #5762, .F. ) ;
#17434=CARTESIAN_POINT ( 'NONE',  ( 9.959635380193999410, -5.406637819064000539, 7.700301345050000634 ) ) ;
#17436=ORIENTED_EDGE ( 'NONE', *, *, #3608, .T. ) ;
#17438=ADVANCED_FACE ( 'NONE', ( #3601 ), #24937, .F. ) ;
#17441=CARTESIAN_POINT ( 'NONE',  ( 10.98768472639999949, -0.3876847264043000174, -4.945212061661000469 ) ) ;
#17442=CARTESIAN_POINT ( 'NONE',  ( 10.92546935320999957, -5.641520548727999795, -7.883473948564999390 ) ) ;
#17443=CARTESIAN_POINT ( 'NONE',  ( 7.771966698881652924, -5.059393530258413207, 8.879290890679834902 ) ) ;
#17444=CARTESIAN_POINT ( 'NONE',  ( 9.409308287954999628, -2.634700736117999931, 8.920302460802998823 ) ) ;
#17463=CARTESIAN_POINT ( 'NONE',  ( 11.09999999999999964, -5.449702613288000208, -5.124965750789000296 ) ) ;
#17467=VERTEX_POINT ( 'NONE', #40332 ) ;
#17473=CARTESIAN_POINT ( 'NONE',  ( 10.63462194421999918, -5.668721490782999695, 6.527259573254000635 ) ) ;
#17495=DIRECTION ( 'NONE',  ( 1.000000000000000000, 0.000000000000000000, 0.000000000000000000 ) ) ;
#17496=CARTESIAN_POINT ( 'NONE',  ( 8.331682137624000006, -5.101289325373999262, 6.607176193198000647 ) ) ;
#17537=CARTESIAN_POINT ( 'NONE',  ( 10.67529314679000052, -3.066674550532999977, -8.703235919197002346 ) ) ;
#17539=CARTESIAN_POINT ( 'NONE',  ( 10.98768472625999948, -6.720753154780999772, 5.471698433974999887 ) ) ;
#17545=VERTEX_POINT ( 'NONE', #24859 ) ;
#17549=EDGE_LOOP ( 'NONE', ( #18927, #65668, #58683, #8742, #7742, #59073, #1026, #61055 ) ) ;
#17559=CARTESIAN_POINT ( 'NONE',  ( 10.02800210979000184, -3.452027005875999865, -6.074520565702999697 ) ) ;
#17562=CARTESIAN_POINT ( 'NONE',  ( 10.55909255430753824, -3.020528152026101143, -5.017625565365243290 ) ) ;
#17565=ORIENTED_EDGE ( 'NONE', *, *, #9794, .T. ) ;
#17567=CARTESIAN_POINT ( 'NONE',  ( 10.33085896026999961, -4.880781593996999845, 4.717851323696000243 ) ) ;
#17571=CARTESIAN_POINT ( 'NONE',  ( 10.37026726325999881, -5.571557883540000589, 7.748386351620999868 ) ) ;
#17584=CARTESIAN_POINT ( 'NONE',  ( 10.75911128370000114, -4.477561100530000004, -5.708582007447000173 ) ) ;
#17586=DIRECTION ( 'NONE',  ( 0.000000000000000000, 1.000000000000000000, 0.000000000000000000 ) ) ;
#17590=DIRECTION ( 'NONE',  ( 0.000000000000000000, -1.000000000000000000, 0.000000000000000000 ) ) ;
#17591=CARTESIAN_POINT ( 'NONE',  ( 8.558656745902677443, -3.294699824964758772, 5.942504329580781786 ) ) ;
#17596=CARTESIAN_POINT ( 'NONE',  ( 10.27199419957999993, -3.240085154792000210, 4.537815602971000395 ) ) ;
#17597=CARTESIAN_POINT ( 'NONE',  ( 7.575821720216998401, -3.529668843644999221, 6.549222992663997545 ) ) ;
#17602=CARTESIAN_POINT ( 'NONE',  ( 7.428159769834000059, -3.524402284009999331, 6.653317709399996005 ) ) ;
#17605=CARTESIAN_POINT ( 'NONE',  ( 9.323728576950999880, -3.947350124452999598, 6.051857392047999440 ) ) ;
#17606=CARTESIAN_POINT ( 'NONE',  ( 10.01186131679890856, -2.762178309543651178, 6.265253433400348015 ) ) ;
#17624=CARTESIAN_POINT ( 'NONE',  ( 7.579654319238870563, -4.353725718092394281, 8.815991072544541396 ) ) ;
#17639=CARTESIAN_POINT ( 'NONE',  ( 9.123558059623999128, -5.558929022707999046, 6.272984818914999927 ) ) ;
#17641=CARTESIAN_POINT ( 'NONE',  ( 11.10000000000000142, -2.722910913279374068, -8.517131090127774584 ) ) ;
#17646=DIRECTION ( 'NONE',  ( 0.000000000000000000, -0.8646938284590766077, 0.5022992962614868384 ) ) ;
#17647=FACE_OUTER_BOUND ( 'NONE', #21244, .T. ) ;
#17650=AXIS2_PLACEMENT_3D ( 'NONE', #50634, #13244, #25087 ) ;
#17652=CARTESIAN_POINT ( 'NONE',  ( 11.18236694037999968, -4.516641106826999597, -8.757887038823000125 ) ) ;
#17666=CARTESIAN_POINT ( 'NONE',  ( 10.90000000011000125, -2.899999999889000257, -6.571291220762999430 ) ) ;
#17667=CARTESIAN_POINT ( 'NONE',  ( 9.967845797207999681, -2.034786297409000078, 7.636877353231999344 ) ) ;
#17670=EDGE_CURVE ( 'NONE', #36315, #60701, #28449, .T. ) ;
#17679=CARTESIAN_POINT ( 'NONE',  ( 7.037120559622001004, -4.623636604834999275, 8.651469651195000665 ) ) ;
#17683=B_SPLINE_CURVE_WITH_KNOTS ( 'NONE', 3,
 ( #36182, #42119, #42804, #4694 ),
 .UNSPECIFIED., .F., .F.,
 ( 4, 4 ),
 ( 0.000000000000000000, 1.000000000000000000 ),
 .UNSPECIFIED. ) ;
#17684=CARTESIAN_POINT ( 'NONE',  ( 8.629835589027990750, -5.187744040556002467, -6.859988146772001194 ) ) ;
#17692=CARTESIAN_POINT ( 'NONE',  ( 11.08923508776348754, -3.836355263994051690, -9.039235091851082871 ) ) ;
#17695=EDGE_CURVE ( 'NONE', #40162, #68990, #41967, .T. ) ;
#17697=CARTESIAN_POINT ( 'NONE',  ( 10.26328274790922634, -2.909659596545102644, -8.325272347294594866 ) ) ;
#17698=CARTESIAN_POINT ( 'NONE',  ( 8.434756776051003158, -5.098765216145000778, 6.624660916390000764 ) ) ;
#17718=EDGE_LOOP ( 'NONE', ( #68696, #44287, #52643, #53679, #20389 ) ) ;
#17725=CARTESIAN_POINT ( 'NONE',  ( 8.817462135714999150, -5.100000000000000533, 6.571291218949999902 ) ) ;
#17746=ORIENTED_EDGE ( 'NONE', *, *, #43025, .T. ) ;
#17752=CARTESIAN_POINT ( 'NONE',  ( 9.988720925027999797, -2.842024021884000273, -6.504330542082999322 ) ) ;
#17754=DIRECTION ( 'NONE',  ( -0.7071067811865952013, -0.7071067811864951702, -8.251241205416942814E-08 ) ) ;
#17763=CARTESIAN_POINT ( 'NONE',  ( 10.27706886429732158, -2.899999999999999911, -6.444141223373538452 ) ) ;
#17773=CARTESIAN_POINT ( 'NONE',  ( 8.887168146795000112, -2.193670085072000120, 7.400591740205000768 ) ) ;
#17774=CARTESIAN_POINT ( 'NONE',  ( 9.798320215454998205, -2.757678812098000254, -6.584768124342000206 ) ) ;
#17789=CARTESIAN_POINT ( 'NONE',  ( 9.409421956854998825, -2.113407700033000047, 7.914197133433000353 ) ) ;
#17790=CARTESIAN_POINT ( 'NONE',  ( 8.898558059623999483, -5.146736128384000075, 6.597417125647000447 ) ) ;
#17795=CARTESIAN_POINT ( 'NONE',  ( 8.039320795308336542, -3.234825695714153238, 5.919796682457031167 ) ) ;
#17796=CARTESIAN_POINT ( 'NONE',  ( 10.87021507563000000, -2.226042145532000305, 7.782753277595999997 ) ) ;
#17808=EDGE_CURVE ( 'NONE', #31101, #63766, #51388, .T. ) ;
#17816=CARTESIAN_POINT ( 'NONE',  ( 7.919004440377000797, -5.361050935357000391, 6.973449182446000094 ) ) ;
#17822=CARTESIAN_POINT ( 'NONE',  ( 10.41839555962000041, -4.531908721143000029, -9.270473926467998282 ) ) ;
#17825=CARTESIAN_POINT ( 'NONE',  ( 8.079724940884622342, -4.352763894256449717, 8.815588961479031482 ) ) ;
#17839=EDGE_CURVE ( 'NONE', #17921, #33287, #50505, .T. ) ;
#17848=CARTESIAN_POINT ( 'NONE',  ( 8.434600867921000500, -5.100000003633000212, 6.577466067358000323 ) ) ;
#17857=B_SPLINE_CURVE_WITH_KNOTS ( 'NONE', 3,
 ( #61734, #13855, #56496, #8600, #46006, #29950, #56845, #51253, #35523, #8943 ),
 .UNSPECIFIED., .F., .F.,
 ( 4, 2, 2, 2, 4 ),
 ( 0.1324350869623206473, 0.3493263152217405132, 0.5662175434811602681, 0.7831087717405801341, 1.000000000000000000 ),
 .UNSPECIFIED. ) ;
#17858=ADVANCED_FACE ( 'NONE', ( #22004 ), #11175, .T. ) ;
#17864=ORIENTED_EDGE ( 'NONE', *, *, #12080, .T. ) ;
#17873=DIRECTION ( 'NONE',  ( 0.000000000000000000, 1.000000000000000000, 0.000000000000000000 ) ) ;
#17875=EDGE_LOOP ( 'NONE', ( #48059, #27321, #9198, #61713 ) ) ;
#17880=CARTESIAN_POINT ( 'NONE',  ( 10.76537527815838580, -5.100000000000000533, 6.445686799303629755 ) ) ;
#17887=B_SPLINE_CURVE_WITH_KNOTS ( 'NONE', 3,
 ( #1518, #48728, #6753, #60253, #44873 ),
 .UNSPECIFIED., .F., .F.,
 ( 4, 1, 4 ),
 ( 0.000000000000000000, 0.5000000000000000000, 1.000000000000000000 ),
 .UNSPECIFIED. ) ;
#17889=CARTESIAN_POINT ( 'NONE',  ( 10.19794194037999979, -4.262172867567000090, -8.834326937932999613 ) ) ;
#17899=ORIENTED_EDGE ( 'NONE', *, *, #10436, .T. ) ;
#17907=CARTESIAN_POINT ( 'NONE',  ( 10.90421209872000041, -3.863781031729999871, -9.185081053980001187 ) ) ;
#17916=CARTESIAN_POINT ( 'NONE',  ( 10.68674208995000008, -5.041113534315000422, 5.111026935337999788 ) ) ;
#17920=CARTESIAN_POINT ( 'NONE',  ( 10.44675369521999997, -2.885048926231000177, 8.863479194807000638 ) ) ;
#17921=VERTEX_POINT ( 'NONE', #42653 ) ;
#17930=CYLINDRICAL_SURFACE ( 'NONE', #54022, 0.5000000000000002220 ) ;
#17933=CARTESIAN_POINT ( 'NONE',  ( 11.11264194660999927, -2.146089039267000231, -7.517188649391000510 ) ) ;
#17937=CARTESIAN_POINT ( 'NONE',  ( 9.392147628284998717, -2.890602650755999647, -6.682694598879999504 ) ) ;
#17944=CARTESIAN_POINT ( 'NONE',  ( 10.54700110996000006, -2.946846751162999656, 4.944912775081999889 ) ) ;
#17945=CARTESIAN_POINT ( 'NONE',  ( 7.443695762906002322, -3.525420668437998728, 6.642224720921002579 ) ) ;
#17950=CARTESIAN_POINT ( 'NONE',  ( 9.013429960698999821, -4.933961117404000341, 8.417889755737999025 ) ) ;
#17954=CARTESIAN_POINT ( 'NONE',  ( 9.034116535116000435, -4.695350938297000454, 8.660677768253002284 ) ) ;
#17955=LINE ( 'NONE', #12356, #37499 ) ;
#17962=CARTESIAN_POINT ( 'NONE',  ( 9.065585557054992805, -2.892971862670999705, -6.682168649839002939 ) ) ;
#17967=CARTESIAN_POINT ( 'NONE',  ( 9.776078604427999252, -4.565692099013000771, -8.879633571423999783 ) ) ;
#17981=CARTESIAN_POINT ( 'NONE',  ( 10.44079553769483404, -5.100000000000000533, 6.662590550628412878 ) ) ;
#17988=CARTESIAN_POINT ( 'NONE',  ( 11.05833333333536928, -2.548905579444654901, 7.980400043918773889 ) ) ;
#17995=CARTESIAN_POINT ( 'NONE',  ( 11.01267610329000135, -8.059176674844000132, 6.866686629167999101 ) ) ;
#18001=DIRECTION ( 'NONE',  ( 0.7660444348520201174, 3.621652213051094873E-11, 0.6427876195387159930 ) ) ;
#18003=CARTESIAN_POINT ( 'NONE',  ( 10.27427156480999848, -4.600000212792999754, 4.944156960788000710 ) ) ;
#18007=CARTESIAN_POINT ( 'NONE',  ( 9.351982841559774329, -3.410536830733829294, 9.136515536752833455 ) ) ;
#18012=CARTESIAN_POINT ( 'NONE',  ( 11.13214415304999960, -5.330901272402999602, -5.052956475076999077 ) ) ;
#18021=EDGE_LOOP ( 'NONE', ( #31642, #33369, #41905, #2277 ) ) ;
#18025=CARTESIAN_POINT ( 'NONE',  ( 10.50286331871000023, -5.158900740613000302, 8.369962360110999811 ) ) ;
#18026=CARTESIAN_POINT ( 'NONE',  ( 9.135904863751600047, -5.220041948655085307, 6.249571414823495097 ) ) ;
#18027=CARTESIAN_POINT ( 'NONE',  ( 8.513433059625000965, -5.040796345420999636, 8.522966281393001609 ) ) ;
#18050=CARTESIAN_POINT ( 'NONE',  ( 11.04783424078000031, -2.764605797469000148, 5.041477660832000218 ) ) ;
#18060=ORIENTED_EDGE ( 'NONE', *, *, #16800, .F. ) ;
#18069=DIRECTION ( 'NONE',  ( -0.6427876096865049460, 0.000000000000000000, 0.7660444431190069903 ) ) ;
#18073=ORIENTED_EDGE ( 'NONE', *, *, #18254, .F. ) ;
#18083=CARTESIAN_POINT ( 'NONE',  ( 10.38314899745999931, -5.167567567567999731, 6.822293592207000934 ) ) ;
#18097=CARTESIAN_POINT ( 'NONE',  ( 11.01003172897000049, -3.180716007396000133, -6.283809484240999943 ) ) ;
#18098=CARTESIAN_POINT ( 'NONE',  ( 5.700000000000000178, 0.000000000000000000, 0.000000000000000000 ) ) ;
#18102=CARTESIAN_POINT ( 'NONE',  ( 10.14405657264394378, -4.746626309883068551, -8.655951532184957387 ) ) ;
#18105=CARTESIAN_POINT ( 'NONE',  ( 10.22422653164065487, -2.899999999999999911, -6.304440313833538312 ) ) ;
#18117=CARTESIAN_POINT ( 'NONE',  ( 7.282480646792000023, -3.448181789123000218, 9.222458996124998976 ) ) ;
#18131=CARTESIAN_POINT ( 'NONE',  ( 10.27968096967000022, -5.739708848514999850, 7.774962785835000112 ) ) ;
#18136=CARTESIAN_POINT ( 'NONE',  ( 7.933903043726158621, -2.295323260153894651, 7.847068492003852924 ) ) ;
#18137=CARTESIAN_POINT ( 'NONE',  ( 10.99433452212999818, -3.697619272994999928, 5.729306330972000261 ) ) ;
#18138=CARTESIAN_POINT ( 'NONE',  ( 11.09999999999999964, -4.000000000000000000, -7.500000000000000000 ) ) ;
#18147=EDGE_CURVE ( 'NONE', #21661, #22433, #50661, .T. ) ;
#18159=CARTESIAN_POINT ( 'NONE',  ( 8.379706853209000883, -4.282999948634999221, 9.286791354293999490 ) ) ;
#18164=CARTESIAN_POINT ( 'NONE',  ( 10.45625805961999966, -3.661873208228000109, -9.317463915629002003 ) ) ;
#18177=B_SPLINE_CURVE_WITH_KNOTS ( 'NONE', 3,
 ( #49578, #55865, #7973, #39094 ),
 .UNSPECIFIED., .F., .F.,
 ( 4, 4 ),
 ( 0.000000000000000000, 1.000000000000000000 ),
 .UNSPECIFIED. ) ;
#18195=CARTESIAN_POINT ( 'NONE',  ( 8.771640687504598688, -2.873222873814833545, 6.752018918871646846 ) ) ;
#18199=CARTESIAN_POINT ( 'NONE',  ( 10.75620859869496115, -5.323164692320646374, 8.643262214358355067 ) ) ;
#18200=CARTESIAN_POINT ( 'NONE',  ( 7.100000000000000533, -4.000000000000000000, 8.849999999999999645 ) ) ;
#18222=ORIENTED_EDGE ( 'NONE', *, *, #11203, .F. ) ;
#18229=CARTESIAN_POINT ( 'NONE',  ( 9.574741131515299486, -3.579783539280765314, 8.799459768376697966 ) ) ;
#18230=CARTESIAN_POINT ( 'NONE',  ( 11.22022944037999892, -3.883088694641999794, -8.854817792072001481 ) ) ;
#18242=CARTESIAN_POINT ( 'NONE',  ( 8.967233804172259681, -5.342662483617720781, 7.359968207274207863 ) ) ;
#18250=CARTESIAN_POINT ( 'NONE',  ( 10.10656447933000024, -4.887648864398999926, -6.257283015674000026 ) ) ;
#18254=EDGE_CURVE ( 'NONE', #50708, #21446, #35620, .T. ) ;
#18255=CIRCLE ( 'NONE', #23839, 10.75000000000000533 ) ;
#18259=CARTESIAN_POINT ( 'NONE',  ( 11.04322985880000196, -5.244997146226999973, 5.031759926182000520 ) ) ;
#18260=CARTESIAN_POINT ( 'NONE',  ( 10.77332351902758845, -2.820285017511723336, -8.179908095962412418 ) ) ;
#18263=CARTESIAN_POINT ( 'NONE',  ( 9.813358178091998951, -5.349400659402999914, 6.657024270273000255 ) ) ;
#18267=( BOUNDED_SURFACE ( )  B_SPLINE_SURFACE ( 3, 3, ( 
 ( #36855, #20083, #10277, #36504, #63751, #31610, #41412, #52932, #41753, #30924, #3987 ),
 ( #26366, #42440, #47692, #48028, #69004, #132, #15863, #58513, #53275, #10617, #52582 ),
 ( #5377, #62718, #52236, #15181, #31271, #57824, #9933, #16893, #64093, #7102, #65477 ),
 ( #6749, #32307, #11305, #64431, #54301, #38222, #10968, #17247, #16553, #28440, #17602 ) ),
 .UNSPECIFIED., .F., .F., .T. ) 
 B_SPLINE_SURFACE_WITH_KNOTS ( ( 4, 4 ),
 ( 4, 1, 1, 1, 1, 1, 1, 1, 4 ),
 ( 0.000000000000000000, 1.000000000000000000 ),
 ( -0.004668278336391999857, 0.000000000000000000, 0.03269534097185999855, 0.06255479614191999937, 0.08986301827556000821, 0.1148786485006000058, 0.1378153831697999931, 0.1587710662428999941, 0.1687086804768000159 ),
 .UNSPECIFIED. ) 
 GEOMETRIC_REPRESENTATION_ITEM ( )  RATIONAL_B_SPLINE_SURFACE ( (
 ( 1.221011660805000121, 1.221011660805000121, 1.221011660805000121, 1.221011660805000121, 1.221011660805000121, 1.221011660805000121, 1.221011660805000121, 1.221011660805000121, 1.221011660805000121, 1.221011660805000121, 1.221011660805000121),
 ( 0.9263294463983999805, 0.9263294463983999805, 0.9263294463983999805, 0.9263294463983999805, 0.9263294463983999805, 0.9263294463983999805, 0.9263294463983999805, 0.9263294463983999805, 0.9263294463983999805, 0.9263294463983999805, 0.9263294463983999805),
 ( 0.9263294463983999805, 0.9263294463983999805, 0.9263294463983999805, 0.9263294463983999805, 0.9263294463983999805, 0.9263294463983999805, 0.9263294463983999805, 0.9263294463983999805, 0.9263294463983999805, 0.9263294463983999805, 0.9263294463983999805),
 ( 1.221011660805000121, 1.221011660805000121, 1.221011660805000121, 1.221011660805000121, 1.221011660805000121, 1.221011660805000121, 1.221011660805000121, 1.221011660805000121, 1.221011660805000121, 1.221011660805000121, 1.221011660805000121) ) ) 
 REPRESENTATION_ITEM ( '' )  SURFACE ( )  );
#18277=CARTESIAN_POINT ( 'NONE',  ( 10.90000000000000036, -5.599999999999999645, 6.571291218949999902 ) ) ;
#18278=B_SPLINE_CURVE_WITH_KNOTS ( 'NONE', 3,
 ( #60079, #23362, #1690, #22316, #44357, #1004, #17068, #59724, #33166, #18945, #8798, #61936, #65791, #66483, #18260, #18606, #39932, #66142 ),
 .UNSPECIFIED., .F., .F.,
 ( 4, 2, 2, 2, 2, 2, 2, 2, 4 ),
 ( 0.1254144463278223376, 0.2190603764462324965, 0.3127063065646425999, 0.4063522366830527588, 0.4999981668014629177, 0.5936440969198727435, 0.6872900270382826804, 0.7809359571566925062, 0.8745818872751025541 ),
 .UNSPECIFIED. ) ;
#18282=CARTESIAN_POINT ( 'NONE',  ( 9.084135711596999840, -5.371875912611999482, -7.370590366721999409 ) ) ;
#18293=CARTESIAN_POINT ( 'NONE',  ( 9.414314870535999802, -3.941041813398000304, 5.878346364186999295 ) ) ;
#18296=CARTESIAN_POINT ( 'NONE',  ( 11.08992739829000129, -5.210546653347999602, 8.327600405525998895 ) ) ;
#18308=CARTESIAN_POINT ( 'NONE',  ( 9.485316810687001166, -2.477793449086000077, -8.275032865112999403 ) ) ;
#18312=EDGE_CURVE ( 'NONE', #21446, #66731, #23006, .T. ) ;
#18325=DIRECTION ( 'NONE',  ( 1.000000000000000000, 0.000000000000000000, 0.000000000000000000 ) ) ;
#18329=CARTESIAN_POINT ( 'NONE',  ( 9.276366930216616069, -4.996498776711455925, -6.096478446050083377 ) ) ;
#18332=CARTESIAN_POINT ( 'NONE',  ( 10.19256470245000123, -2.560274838243000062, 7.664550593243999899 ) ) ;
#18341=DIRECTION ( 'NONE',  ( 1.000000000000000000, 0.000000000000000000, 0.000000000000000000 ) ) ;
#18349=CARTESIAN_POINT ( 'NONE',  ( 9.382621648424837701, -2.846608892234664623, 8.802369146277571943 ) ) ;
#18351=CARTESIAN_POINT ( 'NONE',  ( 8.250655866767852231, -4.995175266012890525, 6.333805738284204345 ) ) ;
#18357=CARTESIAN_POINT ( 'NONE',  ( 10.77962878203999963, -2.397503436487000261, 7.755423856053000442 ) ) ;
#18362=VERTEX_POINT ( 'NONE', #21579 ) ;
#18365=EDGE_CURVE ( 'NONE', #2080, #29508, #33121, .T. ) ;
#18369=CARTESIAN_POINT ( 'NONE',  ( 9.181706853207000307, -3.734278838175999482, 8.942129638874000364 ) ) ;
#18370=CARTESIAN_POINT ( 'NONE',  ( 8.316694573732000606, -2.898380360490000029, 6.611503418275999522 ) ) ;
#18376=CARTESIAN_POINT ( 'NONE',  ( 10.85500481460000088, -2.931066281534000062, -5.151242807010000035 ) ) ;
#18381=CARTESIAN_POINT ( 'NONE',  ( 9.251933059621999078, -5.159251056493999954, 9.109488373271000583 ) ) ;
#18391=EDGE_LOOP ( 'NONE', ( #20618, #47515, #67588, #21638, #10347, #3486, #28268, #40476, #12564, #41186 ) ) ;
#18393=CARTESIAN_POINT ( 'NONE',  ( 7.800894438721999613, -3.218815632501999868, 6.398977300879999497 ) ) ;
#18401=DIRECTION ( 'NONE',  ( 1.000000000000000000, 0.000000000000000000, 0.000000000000000000 ) ) ;
#18403=AXIS2_PLACEMENT_3D ( 'NONE', #38283, #32369, #21513 ) ;
#18408=CARTESIAN_POINT ( 'NONE',  ( 9.457111106897940545, -5.237397863424940958, 8.039624212520665836 ) ) ;
#18412=ORIENTED_EDGE ( 'NONE', *, *, #57294, .F. ) ;
#18413=CARTESIAN_POINT ( 'NONE',  ( 7.603392156809999136, -9.092031481190000264, 5.808920680900000022 ) ) ;
#18416=CARTESIAN_POINT ( 'NONE',  ( 9.143998948451265818, -2.899999999999999911, 6.465127702479446015 ) ) ;
#18424=CARTESIAN_POINT ( 'NONE',  ( 9.725191424783300675, -2.649754699899359522, 7.500009801425228773 ) ) ;
#18425=EDGE_LOOP ( 'NONE', ( #31781, #29701, #42367, #3956, #42667, #17221, #39495, #21806 ) ) ;
#18427=EDGE_CURVE ( 'NONE', #67391, #21093, #10502, .T. ) ;
#18436=ORIENTED_EDGE ( 'NONE', *, *, #48533, .F. ) ;
#18441=CARTESIAN_POINT ( 'NONE',  ( 9.910158555493998378, -2.531067292016000003, -7.917737669614999696 ) ) ;
#18454=EDGE_CURVE ( 'NONE', #37636, #29023, #46901, .T. ) ;
#18457=CARTESIAN_POINT ( 'NONE',  ( 9.133199450400327990, -5.099761357576727328, 6.159710572180335575 ) ) ;
#18461=CARTESIAN_POINT ( 'NONE',  ( 7.924355646793000751, -2.432121990576000314, 6.597519606637999523 ) ) ;
#18465=ORIENTED_EDGE ( 'NONE', *, *, #33187, .F. ) ;
#18474=CARTESIAN_POINT ( 'NONE',  ( 9.799258316471000541, -4.057329063942999525, 9.430691159271001212 ) ) ;
#18481=CARTESIAN_POINT ( 'NONE',  ( 8.060801445049092351, -3.692626997221928331, 5.787670773964787685 ) ) ;
#18482=CARTESIAN_POINT ( 'NONE',  ( 9.166075977534999808, -4.023333687735000552, 9.122281080215000060 ) ) ;
#18493=B_SPLINE_CURVE_WITH_KNOTS ( 'NONE', 3,
 ( #51384, #3481, #45798, #40546, #34285, #24817, #66078, #61192, #45461, #18199, #13313, #67111, #60846, #66425, #29047, #35316, #34635, #55947, #8052, #50703, #24126, #13648, #66775, #46143, #18891, #40216, #56634, #34976, #8737, #40894, #35658, #62890, #57650, #68475, #37029, #58341, #47172 ),
 .UNSPECIFIED., .F., .F.,
 ( 4, 2, 2, 2, 2, 2, 2, 2, 2, 1, 1, 1, 2, 2, 2, 2, 2, 2, 2, 4 ),
 ( 0.000000000000000000, 0.06250000000000018041, 0.1250000000000003608, 0.1875000000000005551, 0.2500000000000007216, 0.3125000000000008882, 0.3750000000000011102, 0.4375000000000012768, 0.4687500000000014433, 0.4843750000000012212, 0.4921875000000011657, 0.4960937500000008327, 0.4980468750000006106, 0.5000000000000003331, 0.6250000000000004441, 0.7500000000000005551, 0.8125000000000004441, 0.8750000000000003331, 0.9375000000000001110, 1.000000000000000000 ),
 .UNSPECIFIED. ) ;
#18505=CARTESIAN_POINT ( 'NONE',  ( 8.636456853209999451, -3.869396851328000153, 5.695656592546999519 ) ) ;
#18510=VECTOR ( 'NONE', #27740, 1000.000000000000000 ) ;
#18512=CARTESIAN_POINT ( 'NONE',  ( 10.03977055961999909, -2.255583827894000137, -8.111980070942999888 ) ) ;
#18568=CARTESIAN_POINT ( 'NONE',  ( 7.355148097746750935, -3.352078922218864498, 9.122887315503605876 ) ) ;
#18584=ORIENTED_EDGE ( 'NONE', *, *, #12102, .F. ) ;
#18588=CARTESIAN_POINT ( 'NONE',  ( 8.959695231899726053, -5.323626131866632250, 7.230905480027200127 ) ) ;
#18592=CARTESIAN_POINT ( 'NONE',  ( 9.716851002543000604, -2.832432432432000269, 6.822293592207000934 ) ) ;
#18597=CARTESIAN_POINT ( 'NONE',  ( 9.924739995124999936, -5.060461104229999840, 8.686133300732999274 ) ) ;
#18602=ORIENTED_EDGE ( 'NONE', *, *, #17670, .T. ) ;
#18603=AXIS2_PLACEMENT_3D ( 'NONE', #6155, #48476, #54753 ) ;
#18606=CARTESIAN_POINT ( 'NONE',  ( 10.79415884302813389, -2.685269952713060793, -7.853379249108617621 ) ) ;
#18609=CARTESIAN_POINT ( 'NONE',  ( 9.611390067472999732, -3.334847606888000193, 5.869121315726000709 ) ) ;
#18610=ORIENTED_EDGE ( 'NONE', *, *, #49962, .F. ) ;
#18615=CARTESIAN_POINT ( 'NONE',  ( 10.61094409420999973, -5.100000000000000533, -6.571291218949999902 ) ) ;
#18617=CARTESIAN_POINT ( 'NONE',  ( 27.64127793187000037, -5.599999999999999645, 6.571291218949999902 ) ) ;
#18625=CARTESIAN_POINT ( 'NONE',  ( 9.702742433789000032, -5.491975933468000726, -7.893788029530999673 ) ) ;
#18632=CARTESIAN_POINT ( 'NONE',  ( 11.09500527153999982, -2.761300632964000190, 5.054570525499999967 ) ) ;
#18637=CARTESIAN_POINT ( 'NONE',  ( 9.753140057121997941, -4.104977100659999323, 9.293279163877999238 ) ) ;
#18640=CARTESIAN_POINT ( 'NONE',  ( 10.50286331871000023, -5.158900740613000302, 8.369962360110999811 ) ) ;
#18643=VERTEX_POINT ( 'NONE', #42772 ) ;
#18648=CARTESIAN_POINT ( 'NONE',  ( 11.00000000000000000, -0.4000000000000000222, 7.331472342878999626 ) ) ;
#18652=CARTESIAN_POINT ( 'NONE',  ( 9.130720302798000176, -5.231133027468000130, -6.569831606205999819 ) ) ;
#18665=EDGE_LOOP ( 'NONE', ( #42139, #9377, #61519, #18610 ) ) ;
#18674=CARTESIAN_POINT ( 'NONE',  ( 11.00833333333534370, -3.620091288824273335, 8.928205453213877263 ) ) ;
#18677=FACE_OUTER_BOUND ( 'NONE', #15166, .T. ) ;
#18691=CARTESIAN_POINT ( 'NONE',  ( 9.389934021418374854, -2.724469859320958420, 8.694040795412995237 ) ) ;
#18693=LINE ( 'NONE', #57114, #12453 ) ;
#18699=CARTESIAN_POINT ( 'NONE',  ( 9.753140057121997941, -4.104977100659999323, 9.293279163877999238 ) ) ;
#18706=EDGE_CURVE ( 'NONE', #44775, #57248, #23758, .T. ) ;
#18709=CARTESIAN_POINT ( 'NONE',  ( 9.129428851719998406, -5.099284414202999827, 6.151604790022999758 ) ) ;
#18713=CARTESIAN_POINT ( 'NONE',  ( 11.02035356290999957, -5.792383855159999761, 5.015468424570999950 ) ) ;
#18714=CARTESIAN_POINT ( 'NONE',  ( 7.766851002543999627, -2.832432432432000269, 6.822293592207000934 ) ) ;
#18717=CARTESIAN_POINT ( 'NONE',  ( 11.09999999999999964, -2.649999999999999911, 7.500000000000000000 ) ) ;
#18721=ORIENTED_EDGE ( 'NONE', *, *, #14747, .T. ) ;
#18737=CARTESIAN_POINT ( 'NONE',  ( 11.09999999999999964, -7.940796613052000019, -6.945951997396999644 ) ) ;
#18745=CARTESIAN_POINT ( 'NONE',  ( 9.625409048293999348, -2.899999999999999911, -6.226580113766999602 ) ) ;
#18746=CARTESIAN_POINT ( 'NONE',  ( 9.069066892820998760, -5.132803099462346808, -6.762400598726751255 ) ) ;
#18750=CARTESIAN_POINT ( 'NONE',  ( 10.03612181215999932, -3.011786236723999810, 8.746965724352000038 ) ) ;
#18753=CARTESIAN_POINT ( 'NONE',  ( 9.202754440379999679, -2.542850487891999745, 7.419808283050000064 ) ) ;
#18755=ORIENTED_EDGE ( 'NONE', *, *, #55712, .F. ) ;
#18764=CARTESIAN_POINT ( 'NONE',  ( 10.52638330645999964, -2.451090818816000105, 6.282756943804999494 ) ) ;
#18766=CARTESIAN_POINT ( 'NONE',  ( 11.09999999999999964, -6.593648099371000271, -5.598803483715999896 ) ) ;
#18775=CARTESIAN_POINT ( 'NONE',  ( 9.051550650638001017, -2.899999999999999911, 6.227445478845999638 ) ) ;
#18784=CARTESIAN_POINT ( 'NONE',  ( 11.07336076184000007, -2.375557098086999996, -8.393541296344000813 ) ) ;
#18787=CARTESIAN_POINT ( 'NONE',  ( 9.020066447149183375, -5.146940009916286307, 8.214567059322398279 ) ) ;
#18788=ORIENTED_EDGE ( 'NONE', *, *, #62444, .F. ) ;
#18794=CARTESIAN_POINT ( 'NONE',  ( 9.856851002545999663, -2.832432432432000269, -6.822293592207000934 ) ) ;
#18795=CARTESIAN_POINT ( 'NONE',  ( 7.501441940376999185, -2.138201851198999748, 6.814774777484000623 ) ) ;
#18800=DIRECTION ( 'NONE',  ( 1.000000000000000000, 9.560366183076000235E-10, 1.449015955545000044E-09 ) ) ;
#18808=CARTESIAN_POINT ( 'NONE',  ( 7.410855646792000151, -2.302293129340000188, 6.875167727519000849 ) ) ;
#18821=CARTESIAN_POINT ( 'NONE',  ( 9.247349085094461074, -4.940696344428553211, -6.064447655904166901 ) ) ;
#18823=CARTESIAN_POINT ( 'NONE',  ( 11.14993998249000029, -2.627133311863999676, 6.696092388640000337 ) ) ;
#18827=CARTESIAN_POINT ( 'NONE',  ( 10.10735564678999943, -4.293585439421999439, -8.994200998147999115 ) ) ;
#18828=CARTESIAN_POINT ( 'NONE',  ( 8.005929440722622914, -2.667435911584553843, 6.373521026562600333 ) ) ;
#18829=CARTESIAN_POINT ( 'NONE',  ( 10.55991645936999923, -5.094263939633999705, 6.075409946530999861 ) ) ;
#18833=CARTESIAN_POINT ( 'NONE',  ( 10.98942773129999928, -5.061072618684999469, -5.190416327777001015 ) ) ;
#18836=CARTESIAN_POINT ( 'NONE',  ( 9.096071945540000314, -5.102479135096000817, -6.621020973615999061 ) ) ;
#18837=VERTEX_POINT ( 'NONE', #4162 ) ;
#18838=CARTESIAN_POINT ( 'NONE',  ( 10.10633213213999859, -4.301175052434000001, -8.935144319903001175 ) ) ;
#18841=CARTESIAN_POINT ( 'NONE',  ( 8.202894943314742449, -2.713916317890127328, 7.026332083725546518 ) ) ;
#18848=CARTESIAN_POINT ( 'NONE',  ( 8.893206853209999707, -3.977267280662000193, 9.308921106447000327 ) ) ;
#18850=ORIENTED_EDGE ( 'NONE', *, *, #53095, .T. ) ;
#18853=CARTESIAN_POINT ( 'NONE',  ( 10.58470685321000104, -2.966812129551000154, -8.831977776575000050 ) ) ;
#18864=CIRCLE ( 'NONE', #52333, 0.3000000000000000444 ) ;
#18891=CARTESIAN_POINT ( 'NONE',  ( 10.83610788131087688, -3.761915004978170440, 9.251916359107640986 ) ) ;
#18892=CARTESIAN_POINT ( 'NONE',  ( 9.523691940378000709, -4.852736108563000528, 8.683927195503999386 ) ) ;
#18896=ORIENTED_EDGE ( 'NONE', *, *, #30948, .F. ) ;
#18898=EDGE_CURVE ( 'NONE', #41892, #48331, #64263, .T. ) ;
#18906=CARTESIAN_POINT ( 'NONE',  ( 10.90000000000000036, -5.283926297003000094, 7.082827057608000132 ) ) ;
#18910=LINE ( 'NONE', #56311, #50885 ) ;
#18927=ORIENTED_EDGE ( 'NONE', *, *, #8958, .F. ) ;
#18932=ADVANCED_FACE ( 'NONE', ( #58685 ), #49766, .F. ) ;
#18937=CARTESIAN_POINT ( 'NONE',  ( 10.34947173981000113, -4.457565973839000328, 6.154866550070000386 ) ) ;
#18943=CARTESIAN_POINT ( 'NONE',  ( 11.07206039417999932, -5.781505909594000236, -5.100555594908000145 ) ) ;
#18945=CARTESIAN_POINT ( 'NONE',  ( 10.70039988502568029, -3.823246508712720537, -8.849946088921091913 ) ) ;
#18948=CARTESIAN_POINT ( 'NONE',  ( 10.09181272066999924, -2.440908155048000516, 7.817368209339999652 ) ) ;
#18961=DIRECTION ( 'NONE',  ( 0.000000000000000000, -0.8648648648648717963, -0.5020047465136829867 ) ) ;
#18965=CARTESIAN_POINT ( 'NONE',  ( 9.482733921870000415, -2.757678812098000254, -6.584768124342000206 ) ) ;
#18974=ADVANCED_FACE ( 'NONE', ( #54220 ), #5634, .F. ) ;
#18976=CARTESIAN_POINT ( 'NONE',  ( 9.724613486786999772, -2.928302463146000179, 8.718481221599999387 ) ) ;
#18978=DIRECTION ( 'NONE',  ( 0.000000000000000000, 0.000000000000000000, -1.000000000000000000 ) ) ;
#18979=CARTESIAN_POINT ( 'NONE',  ( 10.68904248846000016, -2.568964727443000307, 7.728094434513999467 ) ) ;
#18984=CARTESIAN_POINT ( 'NONE',  ( 10.80830512578202018, -5.096679906444030017, -5.098988276665438413 ) ) ;
#18986=CARTESIAN_POINT ( 'NONE',  ( 11.13220159457000058, -2.670356040834999778, 5.051244813867000083 ) ) ;
#18989=CARTESIAN_POINT ( 'NONE',  ( 9.350728814717999882, -3.197530835772000035, -8.817973615970998935 ) ) ;
#18991=ORIENTED_EDGE ( 'NONE', *, *, #34201, .F. ) ;
#18993=CARTESIAN_POINT ( 'NONE',  ( 10.99791623168052723, -5.186580209184203483, -5.071961089083791840 ) ) ;
#18994=LINE ( 'NONE', #3589, #58892 ) ;
#19001=CARTESIAN_POINT ( 'NONE',  ( 9.323371907591601726, -2.820206136178896372, -8.179990968853758204 ) ) ;
#19011=CARTESIAN_POINT ( 'NONE',  ( 9.393246442089999704, -5.100000000000000533, -6.421387671005999387 ) ) ;
#19018=VERTEX_POINT ( 'NONE', #59814 ) ;
#19020=DIRECTION ( 'NONE',  ( 0.000000000000000000, 0.000000000000000000, 1.000000000000000000 ) ) ;
#19026=CARTESIAN_POINT ( 'NONE',  ( 9.382630518809056852, -2.846461560144221803, 8.802238404894030310 ) ) ;
#19029=CARTESIAN_POINT ( 'NONE',  ( 9.934999999999998721, -4.640430492595999823, -9.117542781427999898 ) ) ;
#19033=CARTESIAN_POINT ( 'NONE',  ( 10.37373728961999930, -2.215269876326000364, 7.703982265807999497 ) ) ;
#19035=CARTESIAN_POINT ( 'NONE',  ( 11.01356641589999974, -2.786433584103999994, 6.253463831328000211 ) ) ;
#19036=ORIENTED_EDGE ( 'NONE', *, *, #24051, .F. ) ;
#19037=ORIENTED_EDGE ( 'NONE', *, *, #57252, .F. ) ;
#19041=CARTESIAN_POINT ( 'NONE',  ( 9.972537864286000087, -2.899999999999999911, -6.571291218949999902 ) ) ;
#19043=CARTESIAN_POINT ( 'NONE',  ( 6.953073139469000630, -9.233001678504999532, 5.200628701625999994 ) ) ;
#19052=CARTESIAN_POINT ( 'NONE',  ( 9.402304893999998470, -4.531444417037000072, -6.133284059228000018 ) ) ;
#19055=ADVANCED_FACE ( 'NONE', ( #14001 ), #3155, .T. ) ;
#19057=CARTESIAN_POINT ( 'NONE',  ( 10.96431548498000197, -5.151797042792000347, 5.074130565745999633 ) ) ;
#19065=CARTESIAN_POINT ( 'NONE',  ( 11.03776249210999971, -8.050323671732000363, -6.914613055281999543 ) ) ;
#19077=CARTESIAN_POINT ( 'NONE',  ( 11.01776264201000011, -4.914128622650000722, 8.587713430305999651 ) ) ;
#19086=EDGE_CURVE ( 'NONE', #61050, #46630, #67084, .T. ) ;
#19088=VECTOR ( 'NONE', #18800, 1000.000000000000000 ) ;
#19089=DIRECTION ( 'NONE',  ( -0.7071067268961630514, -0.09465676129217508172, 0.7007425877737639697 ) ) ;
#19094=CARTESIAN_POINT ( 'NONE',  ( 10.77462219945999955, -5.575466189878000911, 8.682669263022999573 ) ) ;
#19101=CARTESIAN_POINT ( 'NONE',  ( 10.41164068750943450, -2.873222873819646583, -6.752018918863353925 ) ) ;
#19102=CARTESIAN_POINT ( 'NONE',  ( 10.91872448493765724, -2.825398922886805497, -6.797111659689116792 ) ) ;
#19110=ORIENTED_EDGE ( 'NONE', *, *, #45232, .T. ) ;
#19112=ADVANCED_FACE ( 'NONE', ( #34646 ), #8063, .F. ) ;
#19116=CARTESIAN_POINT ( 'NONE',  ( 10.01276877312999858, -3.440626575163999945, -9.267592337498999910 ) ) ;
#19122=CARTESIAN_POINT ( 'NONE',  ( 10.62549262323914334, -5.350086361207873509, -7.676738019119357048 ) ) ;
#19123=CARTESIAN_POINT ( 'NONE',  ( 7.629816940376999312, -4.763531818439999732, 5.668890958491999754 ) ) ;
#19137=CARTESIAN_POINT ( 'NONE',  ( 7.705394353206999725, -3.245532552444000185, 8.949627348471000943 ) ) ;
#19147=CARTESIAN_POINT ( 'NONE',  ( 10.90000000000000036, -8.091320520030999219, -7.077643127633000297 ) ) ;
#19152=CARTESIAN_POINT ( 'NONE',  ( 10.41185831014999863, -2.101597930377999912, 7.856264717901999539 ) ) ;
#19157=CARTESIAN_POINT ( 'NONE',  ( 7.962503634123480722, -2.285285773337808912, 7.208897372649888169 ) ) ;
#19158=CARTESIAN_POINT ( 'NONE',  ( 9.414314870535999802, -3.941041813398000304, 5.878346364186999295 ) ) ;
#19162=CARTESIAN_POINT ( 'NONE',  ( 10.48315960899000032, -5.083827399151000570, -4.649899757833000358 ) ) ;
#19167=ORIENTED_EDGE ( 'NONE', *, *, #47274, .T. ) ;
#19168=CARTESIAN_POINT ( 'NONE',  ( 10.09166489801000033, -4.565692099013000771, -8.879633571423999783 ) ) ;
#19180=CARTESIAN_POINT ( 'NONE',  ( 9.021581853209999835, -2.193670085072000120, 7.400591740205000768 ) ) ;
#19185=CARTESIAN_POINT ( 'NONE',  ( 10.09249435321000021, -2.841617206345000035, -8.724656239052000828 ) ) ;
#19196=ADVANCED_FACE ( 'NONE', ( #19926 ), #12360, .T. ) ;
#19205=CARTESIAN_POINT ( 'NONE',  ( 10.28172590882367743, -3.320041345951468159, -8.679799923475449930 ) ) ;
#19216=ADVANCED_FACE ( 'NONE', ( #53113 ), #62900, .F. ) ;
#19221=CARTESIAN_POINT ( 'NONE',  ( 7.919004440377000797, -5.361050935357000391, 6.973449182446000094 ) ) ;
#19236=CARTESIAN_POINT ( 'NONE',  ( 7.218293146793000048, -4.773080213113000347, 8.927399220053999329 ) ) ;
#19240=CARTESIAN_POINT ( 'NONE',  ( 7.418346648492968320, -2.395435861435949221, 8.173148036598570698 ) ) ;
#19247=CARTESIAN_POINT ( 'NONE',  ( 10.76947109217999810, -5.100000000000000533, -6.152188490330000370 ) ) ;
#19251=DIRECTION ( 'NONE',  ( 1.000000000000000000, 0.000000000000000000, 0.000000000000000000 ) ) ;
#19252=CARTESIAN_POINT ( 'NONE',  ( 10.57656694038000111, -5.344897889496000865, -7.298883676216999739 ) ) ;
#19268=DIRECTION ( 'NONE',  ( 0.7071067811865475727, -0.7071067811865475727, 0.000000000000000000 ) ) ;
#19270=CARTESIAN_POINT ( 'NONE',  ( 10.03612181215999932, -3.011786236723999810, 8.746965724352000038 ) ) ;
#19272=CARTESIAN_POINT ( 'NONE',  ( 9.947300131853999972, -4.892806669161000599, -9.067746434455999704 ) ) ;
#19277=ADVANCED_FACE ( 'NONE', ( #9765 ), #47533, .T. ) ;
#19279=CARTESIAN_POINT ( 'NONE',  ( 10.96239535880000027, -6.767634501268999792, -5.462414138040999845 ) ) ;
#19282=EDGE_CURVE ( 'NONE', #41592, #66341, #62562, .T. ) ;
#19286=CARTESIAN_POINT ( 'NONE',  ( 9.409421956854998825, -2.113407700033000047, 7.914197133433000353 ) ) ;
#19300=CARTESIAN_POINT ( 'NONE',  ( 9.350728814717999882, -3.197530835772000035, -8.817973615970998935 ) ) ;
#19310=CARTESIAN_POINT ( 'NONE',  ( 10.49785673611999925, -3.776281940467000275, 5.717636230565000588 ) ) ;
#19314=DIRECTION ( 'NONE',  ( -0.7071067811865975328, -0.7071067811864976127, 3.640777668006986975E-09 ) ) ;
#19316=CARTESIAN_POINT ( 'NONE',  ( 9.520528907821001141, -2.899999999999999911, 6.152188490330000370 ) ) ;
#19321=CARTESIAN_POINT ( 'NONE',  ( 10.45541918308390628, -4.873971636396174034, -4.983734050914551794 ) ) ;
#19325=CARTESIAN_POINT ( 'NONE',  ( 8.973021312994999832, -2.881074422252000389, -6.370633220842000455 ) ) ;
#19328=CARTESIAN_POINT ( 'NONE',  ( 9.304144223516997769, -2.772050158355999994, -8.125211791007998841 ) ) ;
#19331=CARTESIAN_POINT ( 'NONE',  ( 8.924662153698962541, -5.350575487761723537, 7.500021879703682615 ) ) ;
#19340=VECTOR ( 'NONE', #25102, 1000.000000000000000 ) ;
#19343=CARTESIAN_POINT ( 'NONE',  ( 8.591232269961309953, -3.293719616469516165, 8.705632950218230803 ) ) ;
#19352=B_SPLINE_CURVE_WITH_KNOTS ( 'NONE', 3,
 ( #30308, #30996, #15932, #5780, #58584, #200 ),
 .UNSPECIFIED., .F., .F.,
 ( 4, 2, 4 ),
 ( 0.000000000000000000, 0.5000000000000000000, 1.000000000000000000 ),
 .UNSPECIFIED. ) ;
#19353=CARTESIAN_POINT ( 'NONE',  ( 11.09999999999999964, -2.700688486617000006, 5.124965750789000296 ) ) ;
#19368=CARTESIAN_POINT ( 'NONE',  ( 9.483644241562705801, -2.404105139695982718, 6.777660126136261454 ) ) ;
#19373=CARTESIAN_POINT ( 'NONE',  ( 11.13520290286999881, -5.334297965861999558, -5.182437713717999550 ) ) ;
#19379=DIRECTION ( 'NONE',  ( 0.000000000000000000, 1.000000000000000000, 0.000000000000000000 ) ) ;
#19380=ORIENTED_EDGE ( 'NONE', *, *, #2401, .F. ) ;
#19391=CARTESIAN_POINT ( 'NONE',  ( 8.599275817281997192, -4.816070832762001430, -6.340446949048005543 ) ) ;
#19393=DIRECTION ( 'NONE',  ( -0.8660254037844288266, 0.000000000000000000, 0.5000000000000169864 ) ) ;
#19395=LINE ( 'NONE', #18717, #26240 ) ;
#19397=EDGE_CURVE ( 'NONE', #9159, #23524, #7905, .T. ) ;
#19398=CARTESIAN_POINT ( 'NONE',  ( 9.311718600414000235, -4.588307032459999490, -5.987050435448999508 ) ) ;
#19403=B_SPLINE_CURVE_WITH_KNOTS ( 'NONE', 3,
 ( #31736, #57599, #25795, #47125, #68426, #20549, #41873, #31391, #42229, #63536, #26489, #15647, #53055, #47819, #69127, #27873, #64558, #48846, #44308, #17371, #6530, #32766, #603, #49183 ),
 .UNSPECIFIED., .F., .F.,
 ( 4, 2, 1, 2, 2, 2, 2, 2, 2, 1, 2, 2, 4 ),
 ( 0.000000000000000000, 0.06250000000000012490, 0.1250000000000002498, 0.1875000000000003886, 0.2500000000000004996, 0.3750000000000006661, 0.5000000000000008882, 0.6250000000000008882, 0.6875000000000006661, 0.7500000000000005551, 0.8125000000000005551, 0.8750000000000004441, 1.000000000000000000 ),
 .UNSPECIFIED. ) ;
#19415=CARTESIAN_POINT ( 'NONE',  ( 9.674373738639999942, -2.899999999999999911, -6.185493860157000867 ) ) ;
#19416=ORIENTED_EDGE ( 'NONE', *, *, #38432, .T. ) ;
#19420=LINE ( 'NONE', #47374, #41046 ) ;
#19426=CARTESIAN_POINT ( 'NONE',  ( 10.48164908029000131, -4.022873587130999518, 9.090901241422999490 ) ) ;
#19429=CARTESIAN_POINT ( 'NONE',  ( 7.764230646791999924, -4.628942671846000501, 5.991663889842000046 ) ) ;
#19436=CARTESIAN_POINT ( 'NONE',  ( 10.18823468625795492, -2.651251756636299195, 7.275528047993060632 ) ) ;
#19438=CARTESIAN_POINT ( 'NONE',  ( 11.14698053895999941, -5.129799765052999838, 5.886044098803999702 ) ) ;
#19440=DIRECTION ( 'NONE',  ( 0.000000000000000000, 1.000000000000000000, 0.000000000000000000 ) ) ;
#19441=CARTESIAN_POINT ( 'NONE',  ( 10.13382174003999836, -5.176455793257000337, -8.189804425074999727 ) ) ;
#19456=B_SPLINE_CURVE_WITH_KNOTS ( 'NONE', 3,
 ( #17725, #55817, #29608, #39386 ),
 .UNSPECIFIED., .F., .F.,
 ( 4, 4 ),
 ( 0.000000000000000000, 1.000000000000000000 ),
 .UNSPECIFIED. ) ;
#19463=CARTESIAN_POINT ( 'NONE',  ( 9.934206403597999113, -5.120430559539999926, -8.883390070891001855 ) ) ;
#19465=CARTESIAN_POINT ( 'NONE',  ( 8.983363606030074777, -5.350321127414493283, 7.640157910728230028 ) ) ;
#19477=EDGE_CURVE ( 'NONE', #20897, #52805, #2097, .T. ) ;
#19485=CARTESIAN_POINT ( 'NONE',  ( 8.026331853209001110, -5.601799093797000140, 7.176147756900999930 ) ) ;
#19502=CARTESIAN_POINT ( 'NONE',  ( 11.02445830383999947, -3.404091099119999519, 5.822494319281999786 ) ) ;
#19505=FACE_OUTER_BOUND ( 'NONE', #24646, .T. ) ;
#19507=CARTESIAN_POINT ( 'NONE',  ( 8.237169251180624485, -5.550135988664304243, 8.289372690488722384 ) ) ;
#19511=CARTESIAN_POINT ( 'NONE',  ( 10.75904878004999965, -5.211536764922000131, -4.904134446986000206 ) ) ;
#19513=ORIENTED_EDGE ( 'NONE', *, *, #48866, .T. ) ;
#19516=CARTESIAN_POINT ( 'NONE',  ( 9.705151033051999221, -4.316974633926000671, -5.653758079558000027 ) ) ;
#19517=CARTESIAN_POINT ( 'NONE',  ( 10.32322131181000024, -3.346607553924000111, -4.621083566737000048 ) ) ;
#19526=CARTESIAN_POINT ( 'NONE',  ( 7.892605646791999163, -5.480312458445999901, 8.192326492433998908 ) ) ;
#19529=B_SPLINE_SURFACE_WITH_KNOTS ( 'NONE', 3, 3, ( 
 ( #7411, #44149, #34347, #60215 ),
 ( #50072, #49720, #18259, #33303 ),
 ( #1138, #56947, #24789, #65446 ),
 ( #17916, #12320, #65790, #55665 ),
 ( #33996, #6718, #65088, #39233 ),
 ( #7067, #1830, #13019, #28057 ),
 ( #28760, #51358, #17567, #60559 ),
 ( #38894, #59861, #12664, #11967 ),
 ( #44835, #44497, #22450, #55313 ),
 ( #3451, #2179, #67421, #7763 ),
 ( #23494, #30056, #46114, #19545 ) ),
 .UNSPECIFIED., .F., .F., .F.,
 ( 4, 1, 1, 1, 1, 1, 1, 1, 4 ),
 ( 4, 4 ),
 ( 0.5752755569481000641, 0.6250000000000000000, 0.6875000000000000000, 0.7500000000000000000, 0.8125000000000000000, 0.8750000000000000000, 0.9375000000000000000, 1.000000000000000000, 1.016621166648999930 ),
 ( -0.1690624953889000026, 1.168925165984000092 ),
 .UNSPECIFIED. ) ;
#19534=CARTESIAN_POINT ( 'NONE',  ( 10.48598064679000075, -5.506038521567000465, -7.274786670944999756 ) ) ;
#19542=CARTESIAN_POINT ( 'NONE',  ( 8.600625070212519319, -4.994744277835623691, 6.120354035033368056 ) ) ;
#19545=CARTESIAN_POINT ( 'NONE',  ( 10.26109516073000094, -4.557161966536000364, 4.532202352624000063 ) ) ;
#19551=AXIS2_PLACEMENT_3D ( 'NONE', #51812, #3910, #25244 ) ;
#19575=CARTESIAN_POINT ( 'NONE',  ( 9.433105646793000787, -4.954907757874000396, 8.825780921426000347 ) ) ;
#19589=CARTESIAN_POINT ( 'NONE',  ( 8.079129440378000737, -3.524751762020000179, 5.573845465339999805 ) ) ;
#19595=CARTESIAN_POINT ( 'NONE',  ( 7.464673621134763515, -2.291441534361882137, 7.172437561238989012 ) ) ;
#19612=CARTESIAN_POINT ( 'NONE',  ( -14.79345512259999929, -10.48174933044999868, -5.405686454350000503 ) ) ;
#19614=EDGE_LOOP ( 'NONE', ( #68488, #22051, #24088, #49697 ) ) ;
#19621=CARTESIAN_POINT ( 'NONE',  ( 10.96207173348999930, -5.399846879528999999, 7.743266618618998898 ) ) ;
#19637=CARTESIAN_POINT ( 'NONE',  ( 9.743567407955000093, -5.287392049455999832, 8.939957179821000466 ) ) ;
#19644=DIRECTION ( 'NONE',  ( 0.000000000000000000, 1.000000000000000000, 0.000000000000000000 ) ) ;
#19653=LINE ( 'NONE', #51801, #29703 ) ;
#19662=PLANE ( 'NONE',  #47582 ) ;
#19667=CARTESIAN_POINT ( 'NONE',  ( 10.99999999997000089, -4.000000000000000000, -7.500000000000000000 ) ) ;
#19670=CARTESIAN_POINT ( 'NONE',  ( 9.457462135716001583, -5.100000000000000533, -6.571291218949999902 ) ) ;
#19678=CARTESIAN_POINT ( 'NONE',  ( 8.226256224620007274, -3.202920229111001049, -6.615926928587001044 ) ) ;
#19680=CARTESIAN_POINT ( 'NONE',  ( 19.01453011999999987, 0.8000000000000000444, -3.149999999999999911 ) ) ;
#19685=CARTESIAN_POINT ( 'NONE',  ( 7.000000000000000000, -7.526486366024999874, 3.526486366024999874 ) ) ;
#19695=CARTESIAN_POINT ( 'NONE',  ( 8.570375340018552279, -3.646757250303549913, 8.848425586001473775 ) ) ;
#19717=CARTESIAN_POINT ( 'NONE',  ( 10.99183569977872565, -8.063891305078106697, -6.969091237525657512 ) ) ;
#19722=CARTESIAN_POINT ( 'NONE',  ( 8.133277933996801323, -2.820894615410645123, 8.178702166372193716 ) ) ;
#19727=CARTESIAN_POINT ( 'NONE',  ( 10.76232069631999977, -3.259150589222000072, -8.644998763029001054 ) ) ;
#19736=ADVANCED_FACE ( 'NONE', ( #38859 ), #5042, .T. ) ;
#19741=CARTESIAN_POINT ( 'NONE',  ( 8.894523589655003448, -4.897163489593995500, -6.153759344469004411 ) ) ;
#19744=CARTESIAN_POINT ( 'NONE',  ( 10.98991108309999909, -2.844095821392999657, -5.102617441991000646 ) ) ;
#19745=CARTESIAN_POINT ( 'NONE',  ( 9.534310001152000780, -5.383415012847999392, -8.183490493635000362 ) ) ;
#19772=CARTESIAN_POINT ( 'NONE',  ( 10.96207173348999930, -5.399846879528999999, 7.743266618618998898 ) ) ;
#19774=CARTESIAN_POINT ( 'NONE',  ( 7.674792391072008613, -2.650477653308784376, 7.499986425013215552 ) ) ;
#19775=CARTESIAN_POINT ( 'NONE',  ( 7.555275273711000494, -4.314043295739000250, 8.819145559946001356 ) ) ;
#19783=CARTESIAN_POINT ( 'NONE',  ( 10.20218235306506926, -2.710356544815101909, 7.038640550472702095 ) ) ;
#19785=CARTESIAN_POINT ( 'NONE',  ( 10.09196524370999981, -3.841385669346000231, 5.536421174581999338 ) ) ;
#19789=CARTESIAN_POINT ( 'NONE',  ( 10.44807121817999906, -3.684978196963999864, -6.173109031625999776 ) ) ;
#19809=CARTESIAN_POINT ( 'NONE',  ( 10.35427551197999918, -4.879111827962000270, -8.944027914303999793 ) ) ;
#19811=CARTESIAN_POINT ( 'NONE',  ( 9.010249263028118349, -5.224549296214872740, 8.068167775449891721 ) ) ;
#19821=AXIS2_PLACEMENT_3D ( 'NONE', #64359, #53551, #42716 ) ;
#19822=B_SPLINE_CURVE_WITH_KNOTS ( 'NONE', 3,
 ( #12298, #54946, #53900, #17185 ),
 .UNSPECIFIED., .F., .F.,
 ( 4, 4 ),
 ( 0.000000000000000000, 1.000000000000000000 ),
 .UNSPECIFIED. ) ;
#19823=EDGE_CURVE ( 'NONE', #69025, #13775, #12494, .T. ) ;
#19830=ORIENTED_EDGE ( 'NONE', *, *, #65652, .T. ) ;
#19831=CARTESIAN_POINT ( 'NONE',  ( 9.272293146792000229, -3.705847642455000202, 9.096432253453999195 ) ) ;
#19836=CARTESIAN_POINT ( 'NONE',  ( 10.90000000000000036, -0.2999999999999999889, -9.662944685757000940 ) ) ;
#19837=EDGE_CURVE ( 'NONE', #41592, #25195, #45074, .T. ) ;
#19843=CARTESIAN_POINT ( 'NONE',  ( 9.209046587350854907, -5.018376794265571483, -6.218521724468556222 ) ) ;
#19845=LINE ( 'NONE', #61803, #38844 ) ;
#19847=ORIENTED_EDGE ( 'NONE', *, *, #64394, .T. ) ;
#19848=CARTESIAN_POINT ( 'NONE',  ( 7.840802619469265267, -4.754872393406737174, 6.367696273718201461 ) ) ;
#19850=CARTESIAN_POINT ( 'NONE',  ( 8.094940203606975970, -4.449604110491481634, 5.819802056068767548 ) ) ;
#19852=ORIENTED_EDGE ( 'NONE', *, *, #54172, .F. ) ;
#19853=CARTESIAN_POINT ( 'NONE',  ( 10.49268136245999905, -4.966242441184999912, -4.914681127036000241 ) ) ;
#19868=CARTESIAN_POINT ( 'NONE',  ( 7.262120559621999760, -4.847802017252000439, 9.065364004483999594 ) ) ;
#19873=AXIS2_PLACEMENT_3D ( 'NONE', #10124, #20961, #14687 ) ;
#19874=CARTESIAN_POINT ( 'NONE',  ( 10.78888064679000003, -2.675723359162999859, -6.748225798259000818 ) ) ;
#19880=EDGE_CURVE ( 'NONE', #3964, #8090, #24261, .T. ) ;
#19884=CARTESIAN_POINT ( 'NONE',  ( 8.572537312455677849, -5.041095006993285388, 6.231862335800022912 ) ) ;
#19888=AXIS2_PLACEMENT_3D ( 'NONE', #9604, #67641, #63077 ) ;
#19889=DIRECTION ( 'NONE',  ( 1.000000000000000000, 0.000000000000000000, 0.000000000000000000 ) ) ;
#19912=ORIENTED_EDGE ( 'NONE', *, *, #19397, .F. ) ;
#19926=FACE_OUTER_BOUND ( 'NONE', #66357, .T. ) ;
#19933=CARTESIAN_POINT ( 'NONE',  ( 8.849379440379999906, -3.975070057433999438, 9.483761758588999058 ) ) ;
#19937=CARTESIAN_POINT ( 'NONE',  ( 10.03977055961999909, -2.255583827894000137, -8.111980070942999888 ) ) ;
#19938=CARTESIAN_POINT ( 'NONE',  ( 7.581694733679056775, -4.164585657937257324, 5.768241722127926074 ) ) ;
#19940=CARTESIAN_POINT ( 'NONE',  ( 7.936333720142999759, -5.123034382927999175, 6.721303993095999907 ) ) ;
#19945=CARTESIAN_POINT ( 'NONE',  ( 10.55162425919054137, -5.013906213569661929, 5.027077672038467782 ) ) ;
#19951=CARTESIAN_POINT ( 'NONE',  ( 10.98944156655594817, -5.203365389803279228, 6.677358443460799542 ) ) ;
#19967=CARTESIAN_POINT ( 'NONE',  ( 10.42595817177000050, -5.042180160032999403, 8.702227297563000619 ) ) ;
#19976=CARTESIAN_POINT ( 'NONE',  ( 11.12341523360999851, -6.060598086452000821, -5.274801696963999476 ) ) ;
#19977=CARTESIAN_POINT ( 'NONE',  ( 5.700000000000000178, 0.8000000000000000444, 3.149999999999999911 ) ) ;
#19982=DIRECTION ( 'NONE',  ( 0.000000000000000000, 1.000000000000000000, 0.000000000000000000 ) ) ;
#20007=CARTESIAN_POINT ( 'NONE',  ( 9.509907746701999898, -5.077451867123000007, 8.469011304701000498 ) ) ;
#20010=CARTESIAN_POINT ( 'NONE',  ( 10.75110221171000013, -2.822135527917999820, 6.655890318096999714 ) ) ;
#20011=EDGE_CURVE ( 'NONE', #16325, #39811, #20049, .T. ) ;
#20018=CARTESIAN_POINT ( 'NONE',  ( 10.37601093510613559, -4.718927363017628274, -4.957694817182617619 ) ) ;
#20021=CARTESIAN_POINT ( 'NONE',  ( 11.13481874607999877, -2.665701152538000329, 5.178754270907999668 ) ) ;
#20025=CARTESIAN_POINT ( 'NONE',  ( 9.964045559621999004, -3.485908552077000344, -9.275738075927998594 ) ) ;
#20030=CARTESIAN_POINT ( 'NONE',  ( 9.073148997461000675, -5.167567567567999731, -6.822293592207000934 ) ) ;
#20040=CARTESIAN_POINT ( 'NONE',  ( 8.475341021510246264, -5.350570349241358770, 7.499981640446112152 ) ) ;
#20045=CARTESIAN_POINT ( 'NONE',  ( 5.599999999407000217, -1.300000000000000044, -10.56294468516420082 ) ) ;
#20049=B_SPLINE_CURVE_WITH_KNOTS ( 'NONE', 3,
 ( #5227, #41605, #14695, #19940 ),
 .UNSPECIFIED., .F., .F.,
 ( 4, 4 ),
 ( 0.000000000000000000, 1.000000000000000000 ),
 .UNSPECIFIED. ) ;
#20050=VECTOR ( 'NONE', #4781, 1000.000000000000000 ) ;
#20057=CARTESIAN_POINT ( 'NONE',  ( 7.562137788010000250, -9.102769276979000068, -5.790556498848999922 ) ) ;
#20069=CARTESIAN_POINT ( 'NONE',  ( 11.10061802256000085, -3.093055606601000207, -6.153681532251999542 ) ) ;
#20073=CARTESIAN_POINT ( 'NONE',  ( 7.204907196771999978, -0.2999999999999999889, 3.099954730132999714 ) ) ;
#20080=CARTESIAN_POINT ( 'NONE',  ( 8.263772364603003240, -4.793682714277998080, -6.586182036516001759 ) ) ;
#20083=CARTESIAN_POINT ( 'NONE',  ( 8.493436541922999794, -2.902501512378997894, 6.607638123744003167 ) ) ;
#20094=B_SPLINE_SURFACE_WITH_KNOTS ( 'NONE', 3, 3, ( 
 ( #28459, #39286, #8501, #2562, #2229, #12718, #61299, #35423, #55365, #35086, #19328, #34050, #40653, #60954, #45905, #50811, #61986, #23891, #3253 ),
 ( #51156, #17967, #34398, #66878, #60607, #24582, #51490, #45226, #28813, #24922, #56048, #18989, #8845, #7460, #30183, #50123, #18652, #39632, #46253 ),
 ( #67217, #14097, #40317, #13069, #56398, #23544, #29848, #44883, #56747, #66188, #18308, #55716, #7812, #3585, #29153, #66532, #50461, #39985, #8159 ),
 ( #13418, #34737, #29505, #2904, #24234, #45572, #61636, #13752, #15469, #36795, #14781, #52520, #37133, #63343, #67558, #68243, #46603, #4619, #53209 ) ),
 .UNSPECIFIED., .F., .F., .F.,
 ( 4, 4 ),
 ( 4, 1, 1, 1, 1, 1, 1, 1, 1, 1, 1, 1, 1, 1, 1, 1, 4 ),
 ( -0.1039086239011999951, 1.103908623900999864 ),
 ( -0.008849010032007000384, 0.01991027257200999809, 0.04866955517603999831, 0.07742883778006000306, 0.1061881203840999988, 0.1349474029881000126, 0.1637066855920999986, 0.1924659681960999846, 0.2212252508002000018, 0.2499845334042000156, 0.2787438160081999738, 0.3075030986121999876, 0.3362623812162000014, 0.3650216638202999908, 0.3937809464243000046, 0.4225402290282999629, 0.4512995116322999767 ),
 .UNSPECIFIED. ) ;
#20112=CARTESIAN_POINT ( 'NONE',  ( 10.73930809942999964, -2.762991917822000154, 6.801028165221000066 ) ) ;
#20114=CARTESIAN_POINT ( 'NONE',  ( 9.451730340337091363, -5.271997571102815527, 7.951892843798163746 ) ) ;
#20115=CARTESIAN_POINT ( 'NONE',  ( 8.662855646795000197, -2.741638482234999952, 6.457327039244000311 ) ) ;
#20122=CARTESIAN_POINT ( 'NONE',  ( 8.186595852941859874, -2.905265993888614950, 6.578644981517261847 ) ) ;
#20130=CARTESIAN_POINT ( 'NONE',  ( 9.701728707608999969, -4.253751259212999791, -8.839942087209999855 ) ) ;
#20149=ADVANCED_FACE ( 'NONE', ( #59058 ), #56366, .T. ) ;
#20150=CARTESIAN_POINT ( 'NONE',  ( 10.40558062080000035, -5.599331384652000310, -8.437753779290000367 ) ) ;
#20151=CARTESIAN_POINT ( 'NONE',  ( 10.02314899745999988, -5.167567567567999731, -6.822293592207000934 ) ) ;
#20152=CARTESIAN_POINT ( 'NONE',  ( 9.040511248533881883, -4.920473672754849481, 8.487405920180457031 ) ) ;
#20167=ORIENTED_EDGE ( 'NONE', *, *, #5456, .F. ) ;
#20168=CARTESIAN_POINT ( 'NONE',  ( 9.053331853208000268, -5.618388245857000030, 7.727743016644000207 ) ) ;
#20171=ORIENTED_EDGE ( 'NONE', *, *, #2855, .F. ) ;
#20176=ORIENTED_EDGE ( 'NONE', *, *, #55265, .F. ) ;
#20181=CARTESIAN_POINT ( 'NONE',  ( 10.80169466977000070, -3.998196228428999355, 9.431543037543999475 ) ) ;
#20184=CARTESIAN_POINT ( 'NONE',  ( 7.867079331757252270, -5.122016962447125898, 6.719626049376892674 ) ) ;
#20187=CARTESIAN_POINT ( 'NONE',  ( 8.238125043277811699, -5.540983280400556765, 8.307145266245010262 ) ) ;
#20196=CARTESIAN_POINT ( 'NONE',  ( 7.717918984469999799, -2.852331559125000027, 6.784354950350999225 ) ) ;
#20197=FACE_OUTER_BOUND ( 'NONE', #18391, .T. ) ;
#20203=EDGE_CURVE ( 'NONE', #10513, #53921, #35047, .T. ) ;
#20205=VERTEX_POINT ( 'NONE', #39340 ) ;
#20208=CARTESIAN_POINT ( 'NONE',  ( 8.289120559623999185, -4.310353212080000773, 9.459493062793997709 ) ) ;
#20209=CARTESIAN_POINT ( 'NONE',  ( 11.09999999999999964, -5.449702618175999547, 5.124965750789000296 ) ) ;
#20213=CARTESIAN_POINT ( 'NONE',  ( 11.05391814679000184, -5.159486550382999859, -8.487149456222999433 ) ) ;
#20219=LINE ( 'NONE', #4129, #10553 ) ;
#20220=AXIS2_PLACEMENT_3D ( 'NONE', #27059, #64095, #11652 ) ;
#20224=ORIENTED_EDGE ( 'NONE', *, *, #19086, .T. ) ;
#20251=EDGE_LOOP ( 'NONE', ( #45003, #25109, #50839, #63289 ) ) ;
#20264=EDGE_CURVE ( 'NONE', #31044, #21661, #47544, .T. ) ;
#20271=CARTESIAN_POINT ( 'NONE',  ( 7.860168146793000687, -2.263562268490999951, 8.007440964304000985 ) ) ;
#20272=VERTEX_POINT ( 'NONE', #67268 ) ;
#20273=CARTESIAN_POINT ( 'NONE',  ( 9.615066448851507630, -5.349942704376990044, -7.499996115248991124 ) ) ;
#20276=B_SPLINE_CURVE_WITH_KNOTS ( 'NONE', 3,
 ( #18775, #60383, #24012, #66655 ),
 .UNSPECIFIED., .F., .F.,
 ( 4, 4 ),
 ( 0.000000000000000000, 1.000000000000000000 ),
 .UNSPECIFIED. ) ;
#20277=CARTESIAN_POINT ( 'NONE',  ( 7.644425692886670731, -5.344399174148395382, 6.396633767784401847 ) ) ;
#20280=ORIENTED_EDGE ( 'NONE', *, *, #53282, .F. ) ;
#20287=LINE ( 'NONE', #58041, #37116 ) ;
#20292=DIRECTION ( 'NONE',  ( 0.8843050097021416533, 0.1786785991673574547, 0.4313682974156609062 ) ) ;
#20304=CARTESIAN_POINT ( 'NONE',  ( 9.687876499438001332, -5.912252057206999645, 7.772299417761000306 ) ) ;
#20316=CARTESIAN_POINT ( 'NONE',  ( 9.576494682405000347, -4.593972507100000158, 5.662052676321000177 ) ) ;
#20319=ORIENTED_EDGE ( 'NONE', *, *, #19880, .T. ) ;
#20322=CARTESIAN_POINT ( 'NONE',  ( 10.74609562913000005, -4.263104965433000437, 9.276976808608999647 ) ) ;
#20331=CARTESIAN_POINT ( 'NONE',  ( 9.487899699504998452, -4.011292643094999555, -9.373220388412001114 ) ) ;
#20336=CARTESIAN_POINT ( 'NONE',  ( 8.205992358809998777, -3.399999999999999911, 6.138278517058000538 ) ) ;
#20340=AXIS2_PLACEMENT_3D ( 'NONE', #39951, #12684, #65109 ) ;
#20354=EDGE_CURVE ( 'NONE', #52223, #48042, #58428, .T. ) ;
#20361=CARTESIAN_POINT ( 'NONE',  ( 8.693622321799001185, -3.165380393025999162, -6.276830322369005621 ) ) ;
#20364=DIRECTION ( 'NONE',  ( 0.000000000000000000, 1.000000000000000000, 0.000000000000000000 ) ) ;
#20365=CARTESIAN_POINT ( 'NONE',  ( 9.888320559623000605, -5.105186397454999359, -8.895598708036001057 ) ) ;
#20366=CARTESIAN_POINT ( 'NONE',  ( 9.517197013793815330, -5.205368702674399550, 8.206177812345709199 ) ) ;
#20385=FACE_OUTER_BOUND ( 'NONE', #20251, .T. ) ;
#20387=FACE_OUTER_BOUND ( 'NONE', #46186, .T. ) ;
#20389=ORIENTED_EDGE ( 'NONE', *, *, #56434, .T. ) ;
#20396=EDGE_CURVE ( 'NONE', #20484, #46842, #30914, .T. ) ;
#20401=ORIENTED_EDGE ( 'NONE', *, *, #7179, .T. ) ;
#20404=CARTESIAN_POINT ( 'NONE',  ( 11.09034140454999928, -5.289188190482000174, -5.109507762678999754 ) ) ;
#20408=CARTESIAN_POINT ( 'NONE',  ( 9.675541251098000117, -4.656741678598999457, -8.653222148251000334 ) ) ;
#20411=B_SPLINE_CURVE_WITH_KNOTS ( 'NONE', 3,
 ( #63531, #47121, #15643, #15303, #20196 ),
 .UNSPECIFIED., .F., .F.,
 ( 4, 1, 4 ),
 ( 0.000000000000000000, 0.5000000000000000000, 1.000000000000000000 ),
 .UNSPECIFIED. ) ;
#20420=CARTESIAN_POINT ( 'NONE',  ( 7.736994134724001881, -2.836597362165000913, 6.822571831264003350 ) ) ;
#20423=CARTESIAN_POINT ( 'NONE',  ( 11.09999999999999964, -2.700688486617000006, 5.124965750789000296 ) ) ;
#20424=CARTESIAN_POINT ( 'NONE',  ( 10.37122746244000027, -3.416394293729999809, -5.010285895928999977 ) ) ;
#20425=CARTESIAN_POINT ( 'NONE',  ( 9.844904806657000407, -2.626678530444999993, -7.387134320497999340 ) ) ;
#20453=CARTESIAN_POINT ( 'NONE',  ( 11.09648096125000016, -3.099777420064000033, 6.097103007060000301 ) ) ;
#20455=CARTESIAN_POINT ( 'NONE',  ( 8.498348583768846609, -3.349589723688465526, 5.969486571880056935 ) ) ;
#20456=CARTESIAN_POINT ( 'NONE',  ( 7.374102686541000651, -4.389298280625000714, 9.135255728583000945 ) ) ;
#20465=CARTESIAN_POINT ( 'NONE',  ( 10.68403590588000007, -5.436611040123999317, 8.578433628717998971 ) ) ;
#20470=CARTESIAN_POINT ( 'NONE',  ( 10.93146935944000120, -2.472881306517999978, -7.514158774805000718 ) ) ;
#20472=CARTESIAN_POINT ( 'NONE',  ( 10.99239898671664228, -6.454658201019197961, -5.240588185469198024 ) ) ;
#20481=EDGE_CURVE ( 'NONE', #63766, #9350, #24619, .T. ) ;
#20483=CARTESIAN_POINT ( 'NONE',  ( 10.12670810574000058, -3.117521507207000386, 8.613544937223998943 ) ) ;
#20484=VERTEX_POINT ( 'NONE', #30897 ) ;
#20492=DIRECTION ( 'NONE',  ( 0.000000000000000000, 0.2461538461537955413, -0.9692307692307821076 ) ) ;
#20495=CARTESIAN_POINT ( 'NONE',  ( 9.526243286405723154, -2.763914616263006607, -8.778142438547300586 ) ) ;
#20501=CARTESIAN_POINT ( 'NONE',  ( 8.656816940379998826, -5.329429281359999493, 6.027400270608000099 ) ) ;
#20511=ORIENTED_EDGE ( 'NONE', *, *, #48444, .T. ) ;
#20512=CARTESIAN_POINT ( 'NONE',  ( 9.160311019873999427, -4.122021308488999836, 9.013573548576999883 ) ) ;
#20513=ADVANCED_FACE ( 'NONE', ( #3962 ), #34777, .T. ) ;
#20518=AXIS2_PLACEMENT_3D ( 'NONE', #51105, #24533, #2180 ) ;
#20526=CARTESIAN_POINT ( 'NONE',  ( 10.57893103570000015, -4.649956431060000561, 5.681096060554999383 ) ) ;
#20528=ORIENTED_EDGE ( 'NONE', *, *, #68436, .F. ) ;
#20529=CARTESIAN_POINT ( 'NONE',  ( 7.834146155765201236, -4.877287769396863482, 6.428085084284855810 ) ) ;
#20532=CARTESIAN_POINT ( 'NONE',  ( 8.111474497621481206, -4.780564565339348704, 5.942454047483178847 ) ) ;
#20533=AXIS2_PLACEMENT_3D ( 'NONE', #41505, #56900, #36260 ) ;
#20538=ORIENTED_EDGE ( 'NONE', *, *, #67214, .T. ) ;
#20544=DIRECTION ( 'NONE',  ( 1.000000000000000000, 0.000000000000000000, 0.000000000000000000 ) ) ;
#20547=VECTOR ( 'NONE', #27764, 1000.000000000000000 ) ;
#20549=CARTESIAN_POINT ( 'NONE',  ( 8.683840764065545059, -5.715804157004961361, 7.158468558862815634 ) ) ;
#20565=ORIENTED_EDGE ( 'NONE', *, *, #11669, .T. ) ;
#20568=( LENGTH_UNIT ( ) NAMED_UNIT ( * ) SI_UNIT ( .MILLI., .METRE. ) );
#20572=DIRECTION ( 'NONE',  ( 0.8480635683783770418, 0.000000000000000000, 0.5298945026977860406 ) ) ;
#20575=EDGE_CURVE ( 'NONE', #52805, #58951, #28349, .T. ) ;
#20578=CARTESIAN_POINT ( 'NONE',  ( 8.677205275792569950, -4.798748112014699529, -6.411199558850072755 ) ) ;
#20587=CARTESIAN_POINT ( 'NONE',  ( 9.934206403597999113, -5.120430559539999926, -8.883390070891001855 ) ) ;
#20597=EDGE_CURVE ( 'NONE', #53568, #37636, #45841, .T. ) ;
#20598=EDGE_CURVE ( 'NONE', #28877, #9679, #34173, .T. ) ;
#20617=CARTESIAN_POINT ( 'NONE',  ( 8.154706853209001238, -4.255646685191999623, 9.114089645792999406 ) ) ;
#20618=ORIENTED_EDGE ( 'NONE', *, *, #54379, .F. ) ;
#20620=CARTESIAN_POINT ( 'NONE',  ( 9.996404771875521789, -5.349457780297906417, 7.853068642099824359 ) ) ;
#20621=CARTESIAN_POINT ( 'NONE',  ( 10.87274555961999845, -5.407608219159000029, -8.698392243238998844 ) ) ;
#20622=CARTESIAN_POINT ( 'NONE',  ( 7.547935135705676757, -3.440357416814149971, 5.843313060613724019 ) ) ;
#20639=B_SPLINE_CURVE_WITH_KNOTS ( 'NONE', 3,
 ( #9858, #31886, #62316, #19670 ),
 .UNSPECIFIED., .F., .F.,
 ( 4, 4 ),
 ( 0.000000000000000000, 1.000000000000000000 ),
 .UNSPECIFIED. ) ;
#20650=CARTESIAN_POINT ( 'NONE',  ( 11.09424907396999949, -2.431867116603999790, 7.769513708858000633 ) ) ;
#20664=CARTESIAN_POINT ( 'NONE',  ( 11.00589466765999802, -3.012766713855000056, 5.961506477028999385 ) ) ;
#20671=CARTESIAN_POINT ( 'NONE',  ( 10.40727044253999978, -3.797905333157999941, 5.889909992361999969 ) ) ;
#20679=CARTESIAN_POINT ( 'NONE',  ( 10.70920446233376744, -2.899999999999999911, 6.662590550603483486 ) ) ;
#20685=CARTESIAN_POINT ( 'NONE',  ( 10.90291609082000157, -2.900148980393999931, 5.141822371583000262 ) ) ;
#20687=ORIENTED_EDGE ( 'NONE', *, *, #18454, .F. ) ;
#20709=CARTESIAN_POINT ( 'NONE',  ( 10.95319508605000181, -2.845003304712999892, -5.173782098108999250 ) ) ;
#20711=CARTESIAN_POINT ( 'NONE',  ( 9.579652738407462564, -4.352972272612487536, 8.851639610528229341 ) ) ;
#20717=ORIENTED_EDGE ( 'NONE', *, *, #59344, .F. ) ;
#20751=CARTESIAN_POINT ( 'NONE',  ( 8.470944094208999076, -5.100000000000000533, 6.571291218949999902 ) ) ;
#20755=CARTESIAN_POINT ( 'NONE',  ( 9.819572261909000233, -2.688237737290000151, -7.873041261681999359 ) ) ;
#20757=ORIENTED_EDGE ( 'NONE', *, *, #14665, .F. ) ;
#20766=CARTESIAN_POINT ( 'NONE',  ( 7.475100008705002352, -3.230432416208002699, 6.447622763416998914 ) ) ;
#20770=CARTESIAN_POINT ( 'NONE',  ( 11.09999999999999964, -6.518019921535999295, 5.523175303137000114 ) ) ;
#20773=CARTESIAN_POINT ( 'NONE',  ( 10.24961784311999935, -4.184221496660999406, 9.286877953065999947 ) ) ;
#20777=CARTESIAN_POINT ( 'NONE',  ( 8.222954734881996686, -4.680061443183004322, 6.135926641887999189 ) ) ;
#20788=CARTESIAN_POINT ( 'NONE',  ( 6.928163941478000076, -9.243153458936999911, -5.233361216079999600 ) ) ;
#20800=CARTESIAN_POINT ( 'NONE',  ( 11.00589466765999802, -3.012766713855000056, 5.961506477028999385 ) ) ;
#20801=ORIENTED_EDGE ( 'NONE', *, *, #2833, .T. ) ;
#20802=CARTESIAN_POINT ( 'NONE',  ( 9.450686119113880679, -5.278034476077728243, 7.934633963864382800 ) ) ;
#20803=CARTESIAN_POINT ( 'NONE',  ( 9.433105646793000787, -4.954907757874000396, 8.825780921426000347 ) ) ;
#20811=CARTESIAN_POINT ( 'NONE',  ( 10.99433452212999818, -3.697619272994999928, 5.729306330972000261 ) ) ;
#20815=VECTOR ( 'NONE', #14543, 1000.000000000000000 ) ;
#20816=CARTESIAN_POINT ( 'NONE',  ( 9.716851002543000604, -2.832432432432000269, 6.822293592207000934 ) ) ;
#20830=CARTESIAN_POINT ( 'NONE',  ( 8.189586429382003985, -5.107684026525003418, 6.413118510302999731 ) ) ;
#20836=CONICAL_SURFACE ( 'NONE', #64378, 10.64999982788999944, 0.7853981633972997312 ) ;
#20838=CARTESIAN_POINT ( 'NONE',  ( 9.814967517147769271, -2.649990781018497721, -7.499998108648967765 ) ) ;
#20848=CARTESIAN_POINT ( 'NONE',  ( 9.106129440379998385, -4.192917962110999319, 5.525484568403999930 ) ) ;
#20857=ORIENTED_EDGE ( 'NONE', *, *, #34995, .F. ) ;
#20858=CARTESIAN_POINT ( 'NONE',  ( 8.957394353210000659, -2.678334737187000325, 8.735278777293000729 ) ) ;
#20859=CARTESIAN_POINT ( 'NONE',  ( 8.770183059623999355, -3.049610585291000042, 6.392533570808999421 ) ) ;
#20862=VERTEX_POINT ( 'NONE', #34353 ) ;
#20873=AXIS2_PLACEMENT_3D ( 'NONE', #1883, #11662, #38946 ) ;
#20875=ORIENTED_EDGE ( 'NONE', *, *, #59962, .F. ) ;
#20878=CARTESIAN_POINT ( 'NONE',  ( 8.139549708658289973, -5.282892974517072737, 6.298817220362490588 ) ) ;
#20884=ORIENTED_EDGE ( 'NONE', *, *, #56434, .F. ) ;
#20890=AXIS2_PLACEMENT_3D ( 'NONE', #27793, #55389, #17646 ) ;
#20897=VERTEX_POINT ( 'NONE', #39586 ) ;
#20899=CARTESIAN_POINT ( 'NONE',  ( 9.187745559622999991, -5.964711531933999389, 7.776478361891000723 ) ) ;
#20914=( BOUNDED_SURFACE ( )  B_SPLINE_SURFACE ( 3, 3, ( 
 ( #65575, #60340, #13146, #34476, #66610, #61708, #17698, #40061, #7201 ),
 ( #7892, #2979, #56123, #65916, #39360, #66950, #60681, #55442, #29228 ),
 ( #50538, #45976, #10284, #9589, #14849, #57147, #57835, #52247, #9244 ),
 ( #26024, #68312, #30254, #51556, #35831, #52589, #24993, #20777, #47011 ) ),
 .UNSPECIFIED., .F., .F., .T. ) 
 B_SPLINE_SURFACE_WITH_KNOTS ( ( 4, 4 ),
 ( 4, 1, 1, 1, 1, 1, 4 ),
 ( 0.000000000000000000, 1.000000000000000000 ),
 ( 0.8657679006235999841, 0.8794646334505999974, 0.9056938526918999477, 0.9344431701380999655, 0.9658387281735000274, 1.000000000000000000, 1.004641266558000012 ),
 .UNSPECIFIED. ) 
 GEOMETRIC_REPRESENTATION_ITEM ( )  RATIONAL_B_SPLINE_SURFACE ( (
 ( 1.157353709788000007, 1.157353709788000007, 1.157353709788000007, 1.157353709788000007, 1.157353709788000007, 1.157353709788000007, 1.157353709788000007, 1.157353709788000007, 1.157353709788000007),
 ( 0.9475487634039000406, 0.9475487634039000406, 0.9475487634039000406, 0.9475487634039000406, 0.9475487634039000406, 0.9475487634039000406, 0.9475487634039000406, 0.9475487634039000406, 0.9475487634039000406),
 ( 0.9475487634039000406, 0.9475487634039000406, 0.9475487634039000406, 0.9475487634039000406, 0.9475487634039000406, 0.9475487634039000406, 0.9475487634039000406, 0.9475487634039000406, 0.9475487634039000406),
 ( 1.157353709788000007, 1.157353709788000007, 1.157353709788000007, 1.157353709788000007, 1.157353709788000007, 1.157353709788000007, 1.157353709788000007, 1.157353709788000007, 1.157353709788000007) ) ) 
 REPRESENTATION_ITEM ( '' )  SURFACE ( )  );
#20926=CIRCLE ( 'NONE', #55515, 0.8000000000000002665 ) ;
#20961=DIRECTION ( 'NONE',  ( 1.000000000000000000, 0.000000000000000000, 0.000000000000000000 ) ) ;
#20962=CARTESIAN_POINT ( 'NONE',  ( 9.181706853207000307, -3.734278838175999482, 8.942129638874000364 ) ) ;
#20963=ORIENTED_EDGE ( 'NONE', *, *, #45507, .T. ) ;
#20967=CARTESIAN_POINT ( 'NONE',  ( 10.30480805961999913, -5.828319785709999756, -7.226592660401000678 ) ) ;
#20968=CARTESIAN_POINT ( 'NONE',  ( 7.612466077185790603, -4.791086490674309140, 5.950606121273764870 ) ) ;
#20976=VECTOR ( 'NONE', #38066, 1000.000000000000114 ) ;
#20995=CARTESIAN_POINT ( 'NONE',  ( 10.11260824411999870, -3.359889198679999911, 5.859131457670000209 ) ) ;
#21002=EDGE_CURVE ( 'NONE', #22321, #53841, #10174, .T. ) ;
#21010=DIRECTION ( 'NONE',  ( 8.848526463087000198E-11, -8.848494979014000266E-11, -1.000000000000000000 ) ) ;
#21017=CARTESIAN_POINT ( 'NONE',  ( 10.00638553269999953, -5.119272496996000399, 8.420388242270998802 ) ) ;
#21031=CARTESIAN_POINT ( 'NONE',  ( 10.90437356726000040, -2.900476673752999890, 5.132566153004000320 ) ) ;
#21037=CARTESIAN_POINT ( 'NONE',  ( 10.44080359545000114, -5.435731278187999393, 7.303630150377999009 ) ) ;
#21043=CARTESIAN_POINT ( 'NONE',  ( 10.26947109217999810, -5.100000000000000533, -6.152188490330000370 ) ) ;
#21047=CARTESIAN_POINT ( 'NONE',  ( 9.585762625467372899, -5.314684444510202610, -7.853443062599636981 ) ) ;
#21048=DIRECTION ( 'NONE',  ( 0.000000000000000000, 1.000000000000000000, 0.000000000000000000 ) ) ;
#21052=EDGE_CURVE ( 'NONE', #58368, #18643, #29974, .T. ) ;
#21055=CARTESIAN_POINT ( 'NONE',  ( 11.13359748671999938, -2.664949685833000181, -5.114435929787000568 ) ) ;
#21056=CARTESIAN_POINT ( 'NONE',  ( 10.94847055962000049, -3.841065069379000274, -9.341805385095000247 ) ) ;
#21058=LINE ( 'NONE', #6339, #56509 ) ;
#21089=B_SPLINE_CURVE_WITH_KNOTS ( 'NONE', 3,
 ( #15825, #52890, #31918, #42743, #16167, #43440 ),
 .UNSPECIFIED., .F., .F.,
 ( 4, 2, 4 ),
 ( 0.000000000000000000, 0.5000000000000000000, 1.000000000000000000 ),
 .UNSPECIFIED. ) ;
#21093=VERTEX_POINT ( 'NONE', #46894 ) ;
#21097=CARTESIAN_POINT ( 'NONE',  ( 8.424688440789097399, -5.350083765069893360, 7.500019236172019710 ) ) ;
#21101=CARTESIAN_POINT ( 'NONE',  ( 10.69578225082999978, -5.505007625740000243, -7.759264430206000540 ) ) ;
#21102=ORIENTED_EDGE ( 'NONE', *, *, #58230, .T. ) ;
#21105=DIRECTION ( 'NONE',  ( 1.000000000000000000, 0.000000000000000000, 0.000000000000000000 ) ) ;
#21112=CARTESIAN_POINT ( 'NONE',  ( 7.964385314170995933, -2.867871570892000399, 6.759005350280994584 ) ) ;
#21116=CARTESIAN_POINT ( 'NONE',  ( 11.09999999999999964, -5.449702618175999547, 5.124965750789000296 ) ) ;
#21120=CARTESIAN_POINT ( 'NONE',  ( 9.305875415870998424, -4.945293979885000191, 9.077881967919999795 ) ) ;
#21132=EDGE_CURVE ( 'NONE', #32339, #44819, #50017, .T. ) ;
#21136=LINE ( 'NONE', #26732, #58029 ) ;
#21138=VERTEX_POINT ( 'NONE', #44760 ) ;
#21144=DIRECTION ( 'NONE',  ( 0.000000000000000000, 1.000000000000000000, 0.000000000000000000 ) ) ;
#21147=CARTESIAN_POINT ( 'NONE',  ( 10.30047649312000146, -4.027768368024999823, 9.431342508940000258 ) ) ;
#21151=CARTESIAN_POINT ( 'NONE',  ( 7.390495559621999888, -2.216884807317999861, 8.370075800106999253 ) ) ;
#21159=CARTESIAN_POINT ( 'NONE',  ( 11.05639424537999993, -5.030223832177999732, 6.028291574375000295 ) ) ;
#21172=CARTESIAN_POINT ( 'NONE',  ( 8.295839940244002619, -5.118638632597003912, 6.383292232312004266 ) ) ;
#21183=ORIENTED_EDGE ( 'NONE', *, *, #20597, .T. ) ;
#21187=CARTESIAN_POINT ( 'NONE',  ( 8.502043146794999728, -3.869396851328000153, 5.695656592546999519 ) ) ;
#21198=VERTEX_POINT ( 'NONE', #13633 ) ;
#21199=CARTESIAN_POINT ( 'NONE',  ( 7.711433059622000208, -5.797088532631000213, 8.340479314546998424 ) ) ;
#21200=CARTESIAN_POINT ( 'NONE',  ( 9.069724726289001282, -4.108965473266000146, 8.851626696081998702 ) ) ;
#21210=B_SPLINE_CURVE_WITH_KNOTS ( 'NONE', 3,
 ( #21452, #68309, #48032, #42788 ),
 .UNSPECIFIED., .F., .F.,
 ( 4, 4 ),
 ( 0.000000000000000000, 1.000000000000000000 ),
 .UNSPECIFIED. ) ;
#21214=CARTESIAN_POINT ( 'NONE',  ( 7.225322421146570306, -2.650264760010439868, 7.500018091723870128 ) ) ;
#21218=EDGE_CURVE ( 'NONE', #23850, #64065, #35804, .T. ) ;
#21221=CARTESIAN_POINT ( 'NONE',  ( 8.541897605312588126, -3.315623613928524005, 5.901107281712603125 ) ) ;
#21223=VERTEX_POINT ( 'NONE', #39855 ) ;
#21228=FACE_OUTER_BOUND ( 'NONE', #45114, .T. ) ;
#21237=EDGE_CURVE ( 'NONE', #51258, #14644, #8287, .T. ) ;
#21241=B_SPLINE_CURVE_WITH_KNOTS ( 'NONE', 3,
 ( #50645, #45061, #7302, #18836 ),
 .UNSPECIFIED., .F., .F.,
 ( 4, 4 ),
 ( 0.000000000000000000, 1.000000000000000000 ),
 .UNSPECIFIED. ) ;
#21244=EDGE_LOOP ( 'NONE', ( #33200, #54723, #66023, #6871 ) ) ;
#21245=B_SPLINE_SURFACE_WITH_KNOTS ( 'NONE', 3, 3, ( 
 ( #17218, #54272, #1487, #6371, #53927, #11618, #25727, #64402, #16524, #9989, #68364, #65094, #20483, #38543, #59865, #448, #41809, #36565, #32616, #27721, #43798, #33307, #6722, #57889, #59176, #21763, #36221, #6029, #31327, #52638, #5686, #43100, #37852, #11275, #48693 ),
 ( #795, #24189, #38898, #45526, #65795, #50767, #55670, #66837, #18263, #50416, #39583, #44839, #50077, #18948, #7072, #8115, #1834, #60219, #17571, #7768, #66486, #2861, #51108, #2184, #40277, #39238, #56008, #12324, #60907, #2519, #23846, #28411, #13372, #45181, #61594 ),
 ( #66145, #60563, #44153, #33655, #35040, #54972, #18609, #29110, #39937, #29459, #22803, #12670, #61254, #34697, #65451, #13025, #49725, #13711, #44501, #56354, #23152, #17920, #34351, #8460, #34001, #23498, #55319, #7415, #29805, #28764, #36398, #4229, #67516, #52473, #15072 ),
 ( #57714, #25908, #35717, #15424, #19286, #52125, #57368, #20316, #9822, #3210, #19637, #25566, #41643, #45863, #41304, #24538, #46893, #24879, #9472, #51448, #67172, #46555, #62949, #40611, #3884, #46209, #31502, #47238, #31170, #4571, #68197, #40958, #68541, #20664, #67858 ) ),
 .UNSPECIFIED., .F., .F., .F.,
 ( 4, 4 ),
 ( 4, 1, 1, 1, 1, 1, 1, 1, 1, 1, 1, 1, 1, 1, 1, 1, 1, 1, 1, 1, 1, 1, 1, 1, 1, 1, 1, 1, 1, 1, 1, 1, 4 ),
 ( -0.1039086239011999951, 1.103908623900999864 ),
 ( -0.01735257130020999988, 0.01084535706264999969, 0.03904328542550000031, 0.06724121378835999641, 0.09543914215121999944, 0.1236370705141000004, 0.1518349988768999959, 0.1800329272397999947, 0.2082308556026999935, 0.2364287839655000167, 0.2646267123283999601, 0.2928246406912000110, 0.3210225690540999821, 0.3492204974169000331, 0.3774184257798000042, 0.4056163541427000307, 0.4338142825054999707, 0.4620122108683999973, 0.4902101392311999928, 0.5184080675940999638, 0.5466059959569999904, 0.5748039243197999859, 0.6030018526827000125, 0.6311997810455000080, 0.6593977094084000345, 0.6875956377712000300, 0.7157935661340999456, 0.7439914944969999722, 0.7721894228597999676, 0.8003873512226999942, 0.8285852795854999897, 0.8567832079484000163, 0.8849811363112999318 ),
 .UNSPECIFIED. ) ;
#21249=LINE ( 'NONE', #68440, #22982 ) ;
#21255=CARTESIAN_POINT ( 'NONE',  ( 10.96239488738000034, -5.423100855659000352, -4.905500182035000378 ) ) ;
#21261=PLANE ( 'NONE',  #44405 ) ;
#21268=CARTESIAN_POINT ( 'NONE',  ( 10.32322128467999889, -3.399999874579999748, -4.621083553505000552 ) ) ;
#21275=VECTOR ( 'NONE', #1322, 1000.000000000000114 ) ;
#21278=CARTESIAN_POINT ( 'NONE',  ( 9.970944094204998720, -5.100000000000000533, 6.571291218949999902 ) ) ;
#21279=CARTESIAN_POINT ( 'NONE',  ( 9.198982189547734833, -2.717686045645804960, 7.939987363064203052 ) ) ;
#21286=AXIS2_PLACEMENT_3D ( 'NONE', #42292, #52071, #14683 ) ;
#21288=ORIENTED_EDGE ( 'NONE', *, *, #67549, .F. ) ;
#21299=CARTESIAN_POINT ( 'NONE',  ( 10.59303089732000025, -2.436232726560000117, 7.793465286118999913 ) ) ;
#21300=CARTESIAN_POINT ( 'NONE',  ( 7.935745559623000212, -5.430412429559000387, 7.210798766422999329 ) ) ;
#21303=EDGE_CURVE ( 'NONE', #34155, #4646, #25735, .T. ) ;
#21304=EDGE_CURVE ( 'NONE', #10663, #57286, #59165, .T. ) ;
#21306=CARTESIAN_POINT ( 'NONE',  ( 9.888320559623000605, -5.105186397454999359, -8.895598708036001057 ) ) ;
#21307=CARTESIAN_POINT ( 'NONE',  ( 7.746088648720403036, -5.452065268544131982, 8.457849491477853476 ) ) ;
#21321=DIRECTION ( 'NONE',  ( 9.801401651172999747E-11, -9.801400427915999291E-11, 1.000000000000000000 ) ) ;
#21322=VERTEX_POINT ( 'NONE', #21268 ) ;
#21332=CARTESIAN_POINT ( 'NONE',  ( 9.945535518573000999, -2.906050966242999856, 8.880386511481999534 ) ) ;
#21334=CONICAL_SURFACE ( 'NONE', #60413, 1.449999999965999375, 0.7853981633972997312 ) ;
#21343=AXIS2_PLACEMENT_3D ( 'NONE', #37405, #63625, #53488 ) ;
#21350=ORIENTED_EDGE ( 'NONE', *, *, #8880, .T. ) ;
#21371=CYLINDRICAL_SURFACE ( 'NONE', #15975, 1.350000000000000089 ) ;
#21380=EDGE_CURVE ( 'NONE', #20862, #16031, #42449, .T. ) ;
#21384=CARTESIAN_POINT ( 'NONE',  ( 9.637847264149046467, -4.829496491575645756, -8.579553154517226332 ) ) ;
#21390=CARTESIAN_POINT ( 'NONE',  ( 10.41839555962000041, -4.531908721143000029, -9.270473926467998282 ) ) ;
#21411=ORIENTED_EDGE ( 'NONE', *, *, #62179, .F. ) ;
#21414=CARTESIAN_POINT ( 'NONE',  ( 10.90000000000000036, -5.100000000000000533, -6.436740704805999691 ) ) ;
#21430=CARTESIAN_POINT ( 'NONE',  ( 11.01003172897000049, -3.180716007396000133, -6.283809484240999943 ) ) ;
#21431=EDGE_CURVE ( 'NONE', #11630, #51331, #288, .T. ) ;
#21437=CARTESIAN_POINT ( 'NONE',  ( 8.712385177405817416, -3.301664264255438574, -6.339997339881533911 ) ) ;
#21439=DIRECTION ( 'NONE',  ( 1.258720292987999992E-10, 1.258720804380000048E-10, 1.000000000000000000 ) ) ;
#21440=B_SPLINE_CURVE_WITH_KNOTS ( 'NONE', 3,
 ( #44018, #27243, #33871, #38766 ),
 .UNSPECIFIED., .F., .F.,
 ( 4, 4 ),
 ( 0.000000000000000000, 1.000000000000000000 ),
 .UNSPECIFIED. ) ;
#21445=CARTESIAN_POINT ( 'NONE',  ( 7.100000000000000533, -4.000000000000000000, 8.849999999999999645 ) ) ;
#21446=VERTEX_POINT ( 'NONE', #32456 ) ;
#21448=CARTESIAN_POINT ( 'NONE',  ( 10.33483735105000179, -3.422629205013000053, -4.713488022966999758 ) ) ;
#21450=CARTESIAN_POINT ( 'NONE',  ( 7.000000000000000000, -9.186881182980000560, -5.186879035586000164 ) ) ;
#21451=CARTESIAN_POINT ( 'NONE',  ( 9.318721994369999706, -2.755032632138999737, 8.795122807847999269 ) ) ;
#21452=CARTESIAN_POINT ( 'NONE',  ( 9.817462135711998883, -5.100000000000000533, 6.571291218949999902 ) ) ;
#21475=CARTESIAN_POINT ( 'NONE',  ( 9.214598350284001427, -2.899999999999999911, -6.571291218949999902 ) ) ;
#21479=CARTESIAN_POINT ( 'NONE',  ( 10.16829915263999951, -4.567213659083999566, 5.832528837986999726 ) ) ;
#21484=CARTESIAN_POINT ( 'NONE',  ( 9.385311019873999072, -4.135077143711000325, 9.175520401071999288 ) ) ;
#21493=CARTESIAN_POINT ( 'NONE',  ( 10.15903154954000165, -4.166415630773999901, 9.114167874391000623 ) ) ;
#21498=CARTESIAN_POINT ( 'NONE',  ( 10.46297944037999983, -3.993164663709000362, -6.140164943008000087 ) ) ;
#21508=B_SPLINE_SURFACE_WITH_KNOTS ( 'NONE', 3, 3, ( 
 ( #43482, #53953, #32985, #42784, #5714, #48370, #6058, #38927, #16207, #22484, #27751, #58858, #1170, #825, #65126, #1864, #12351, #43826, #37882, #49063, #27395, #59202, #44179, #33684, #48724, #38568, #43127, #53617, #55001, #28088, #64780, #59894, #33339, #60249, #12001 ),
 ( #22142, #37531, #27055, #478, #59550, #1514, #21794, #54654, #49402, #32643, #18637, #24566, #28794, #39967, #23527, #39613, #40635, #67200, #61284, #56034, #13400, #8486, #19310, #34723, #40301, #8142, #29491, #2890, #60938, #13054, #45889, #50105, #2546, #2213, #44869 ),
 ( #34381, #66173, #3239, #14081, #7795, #50797, #18293, #12697, #35406, #56384, #23873, #18976, #13735, #61970, #24214, #61620, #35068, #29832, #45557, #66863, #50444, #51137, #56732, #34035, #8826, #45212, #55699, #30169, #51474, #29136, #23181, #44530, #55347, #65824, #66514 ),
 ( #17950, #39268, #60591, #7444, #30843, #41671, #31532, #4601, #9502, #20007, #25937, #36082, #42370, #25596, #46922, #36775, #41332, #46582, #62639, #47265, #10538, #15451, #31198, #68923, #21037, #9852, #46235, #67542, #52503, #63671, #68570, #58097, #42022, #31879, #37119 ) ),
 .UNSPECIFIED., .F., .F., .F.,
 ( 4, 4 ),
 ( 4, 1, 1, 1, 1, 1, 1, 1, 1, 1, 1, 1, 1, 1, 1, 1, 1, 1, 1, 1, 1, 1, 1, 1, 1, 1, 1, 1, 1, 1, 1, 1, 4 ),
 ( -0.1039086239011999951, 1.103908623900999864 ),
 ( -0.01933701211302999920, 0.01208563257065999909, 0.04350827725433999843, 0.07493092193802000645, 0.1063535666217000075, 0.1377762113054000204, 0.1691988559891000055, 0.2006215006727000150, 0.2320441453564000001, 0.2634667900400999851, 0.2948894347238000258, 0.3263120794074999553, 0.3577347240911999959, 0.3891573687748000054, 0.4205800134584999905, 0.4520026581421999756, 0.4834253028259000162, 0.5148479475096000568, 0.5462705921932000663, 0.5776932368768999959, 0.6091158815606000365, 0.6405385262443000771, 0.6719611709280000067, 0.7033838156117000473, 0.7348064602953000568, 0.7662291049789999864, 0.7976517496627000270, 0.8290743943464000676, 0.8604970390300999972, 0.8919196837138000378, 0.9233423283974000473, 0.9547649730810999769, 0.9861876177648000175 ),
 .UNSPECIFIED. ) ;
#21511=VERTEX_POINT ( 'NONE', #35806 ) ;
#21513=DIRECTION ( 'NONE',  ( 0.000000000000000000, 0.000000000000000000, -1.000000000000000000 ) ) ;
#21514=B_SPLINE_CURVE_WITH_KNOTS ( 'NONE', 3,
 ( #35050, #29815, #25229, #8125 ),
 .UNSPECIFIED., .F., .F.,
 ( 4, 4 ),
 ( 0.000000000000000000, 1.000000000000000000 ),
 .UNSPECIFIED. ) ;
#21521=CARTESIAN_POINT ( 'NONE',  ( 9.475931479132977842, -3.758245030697716427, -9.262048976456073390 ) ) ;
#21522=EDGE_CURVE ( 'NONE', #15201, #53670, #57458, .T. ) ;
#21528=CARTESIAN_POINT ( 'NONE',  ( 7.860168146793000687, -2.263562268490999951, 8.007440964304000985 ) ) ;
#21539=CARTESIAN_POINT ( 'NONE',  ( 9.085769353209000698, -2.821866379289000193, 6.127148604720000336 ) ) ;
#21540=CARTESIAN_POINT ( 'NONE',  ( 9.091120559621998609, -3.762710033898000184, 8.787827024292999667 ) ) ;
#21543=ORIENTED_EDGE ( 'NONE', *, *, #42633, .T. ) ;
#21548=ORIENTED_EDGE ( 'NONE', *, *, #14665, .T. ) ;
#21550=CARTESIAN_POINT ( 'NONE',  ( 9.512931135678952543, -5.100000000000000533, 6.444141223441286925 ) ) ;
#21554=VERTEX_POINT ( 'NONE', #49908 ) ;
#21557=CARTESIAN_POINT ( 'NONE',  ( 8.545743765261121894, -3.391202971854105019, 5.870433013438566050 ) ) ;
#21558=CARTESIAN_POINT ( 'NONE',  ( 10.90000000000000036, -8.091325576830000088, 7.077637346582999811 ) ) ;
#21559=ORIENTED_EDGE ( 'NONE', *, *, #43586, .T. ) ;
#21563=EDGE_CURVE ( 'NONE', #34400, #14642, #34908, .T. ) ;
#21566=CARTESIAN_POINT ( 'NONE',  ( 7.875861560654877636, -4.439160970441643705, 6.199066551597841368 ) ) ;
#21568=CARTESIAN_POINT ( 'NONE',  ( 10.66052890781999984, -2.899999999999999911, -6.152188490330000370 ) ) ;
#21569=CARTESIAN_POINT ( 'NONE',  ( 8.975133088423635996, -5.349981448246158955, 7.499992563499107590 ) ) ;
#21579=CARTESIAN_POINT ( 'NONE',  ( 8.674830025576039105, -2.649890579813208191, 7.499988935010342139 ) ) ;
#21580=EDGE_LOOP ( 'NONE', ( #65934, #19037, #13932, #54481 ) ) ;
#21582=VECTOR ( 'NONE', #9727, 1000.000000000000000 ) ;
#21592=ORIENTED_EDGE ( 'NONE', *, *, #67909, .F. ) ;
#21596=FACE_OUTER_BOUND ( 'NONE', #3498, .T. ) ;
#21603=EDGE_LOOP ( 'NONE', ( #51204, #42028, #53772 ) ) ;
#21605=B_SPLINE_CURVE_WITH_KNOTS ( 'NONE', 3,
 ( #46595, #67901, #20018, #41342, #62655, #19321, #51149, #62986, #52170, #46246, #4270, #9171, #14775, #67552, #57071, #56741, #30177, #3247, #8151, #18984, #41682 ),
 .UNSPECIFIED., .F., .F.,
 ( 4, 2, 2, 2, 2, 2, 2, 1, 2, 2, 4 ),
 ( 0.000000000000000000, 0.2500000000000056066, 0.3750000000000068279, 0.4375000000000077716, 0.5000000000000086597, 0.6250000000000166533, 0.6875000000000203171, 0.7187500000000186517, 0.7343750000000178746, 0.7500000000000172085, 1.000000000000000000 ),
 .UNSPECIFIED. ) ;
#21624=ORIENTED_EDGE ( 'NONE', *, *, #32052, .T. ) ;
#21636=CARTESIAN_POINT ( 'NONE',  ( 10.70441271436000008, -3.444516450945999786, 6.009051312948000323 ) ) ;
#21637=CARTESIAN_POINT ( 'NONE',  ( 8.475644353210000759, -5.095088356574999366, 6.286978111459999852 ) ) ;
#21638=ORIENTED_EDGE ( 'NONE', *, *, #9398, .T. ) ;
#21641=CARTESIAN_POINT ( 'NONE',  ( 10.37239314679000124, -3.992345679293999972, -5.977234595428000397 ) ) ;
#21642=CARTESIAN_POINT ( 'NONE',  ( 7.888460647515415758, -2.737986541543418806, 8.699910899329831082 ) ) ;
#21643=CARTESIAN_POINT ( 'NONE',  ( 10.65050275296000137, -5.200029647236999786, 5.937716681140000397 ) ) ;
#21661=VERTEX_POINT ( 'NONE', #23857 ) ;
#21667=CARTESIAN_POINT ( 'NONE',  ( 11.11504459742000073, -3.456612073675000119, 5.970342812640000218 ) ) ;
#21690=CARTESIAN_POINT ( 'NONE',  ( 8.745593092018999926, -5.100000000000000533, 6.404090157675000228 ) ) ;
#21691=CARTESIAN_POINT ( 'NONE',  ( 9.820206362952999868, -3.883324525498000224, 6.055606607331999847 ) ) ;
#21720=DIRECTION ( 'NONE',  ( 1.000000000000000000, 0.000000000000000000, 0.000000000000000000 ) ) ;
#21721=CARTESIAN_POINT ( 'NONE',  ( 9.564964385875493136, -5.350010280223940207, -7.500002129152480101 ) ) ;
#21722=FACE_OUTER_BOUND ( 'NONE', #37591, .T. ) ;
#21726=CARTESIAN_POINT ( 'NONE',  ( 7.000000000000000000, -6.255435840762999966, -3.000000000000000000 ) ) ;
#21727=CARTESIAN_POINT ( 'NONE',  ( 9.978906853208000527, -5.007779786185999171, -8.772596342864998675 ) ) ;
#21746=CARTESIAN_POINT ( 'NONE',  ( 9.856851002545999663, -2.832432432432000269, -6.822293592207000934 ) ) ;
#21750=CARTESIAN_POINT ( 'NONE',  ( 10.33022766388000058, -2.650179121646999647, -7.694581537458001108 ) ) ;
#21752=ORIENTED_EDGE ( 'NONE', *, *, #38135, .T. ) ;
#21762=PLANE ( 'NONE',  #24035 ) ;
#21763=CARTESIAN_POINT ( 'NONE',  ( 10.85068991645999859, -4.478102922274999287, 6.162028334171000488 ) ) ;
#21765=EDGE_CURVE ( 'NONE', #8532, #8998, #31557, .T. ) ;
#21775=CARTESIAN_POINT ( 'NONE',  ( 10.32701825126999928, -5.663784181836000187, -6.682035927671000408 ) ) ;
#21776=VERTEX_POINT ( 'NONE', #66499 ) ;
#21783=B_SPLINE_CURVE_WITH_KNOTS ( 'NONE', 3,
 ( #13321, #44787, #3153, #45126, #45808 ),
 .UNSPECIFIED., .F., .F.,
 ( 4, 1, 4 ),
 ( 0.000000000000000000, 0.5000000000000000000, 1.000000000000000000 ),
 .UNSPECIFIED. ) ;
#21789=CARTESIAN_POINT ( 'NONE',  ( 7.602716214150000873, -2.929796814311000919, 6.536389039862005035 ) ) ;
#21792=ADVANCED_FACE ( 'NONE', ( #60575 ), #34014, .F. ) ;
#21794=CARTESIAN_POINT ( 'NONE',  ( 9.504901164121001500, -3.934733502342999678, 5.704835336325999151 ) ) ;
#21797=CARTESIAN_POINT ( 'NONE',  ( 11.20904026220999938, -5.937811873294999820, 7.147336919140999001 ) ) ;
#21805=DIRECTION ( 'NONE',  ( 1.000000000000000000, 0.000000000000000000, 0.000000000000000000 ) ) ;
#21806=ORIENTED_EDGE ( 'NONE', *, *, #16084, .F. ) ;
#21812=CARTESIAN_POINT ( 'NONE',  ( 8.239310352252543268, -2.650829846289642688, 7.263894687833495567 ) ) ;
#21814=CARTESIAN_POINT ( 'NONE',  ( 7.673170892156151446, -2.921517931055129580, 8.328373548166320361 ) ) ;
#21822=CARTESIAN_POINT ( 'NONE',  ( 9.799258316471000541, -4.057329063942999525, 9.430691159271001212 ) ) ;
#21836=CARTESIAN_POINT ( 'NONE',  ( 9.848732933287999813, -2.769734897491000325, 6.441850735262000249 ) ) ;
#21841=CARTESIAN_POINT ( 'NONE',  ( 10.10735564678999943, -4.293585439421999439, -8.994200998147999115 ) ) ;
#21869=CARTESIAN_POINT ( 'NONE',  ( 8.785191940379998954, -5.414909314743000301, 8.890670256079998168 ) ) ;
#21883=CARTESIAN_POINT ( 'NONE',  ( 9.112168146794999757, -2.368260286481999710, 7.410200011629000549 ) ) ;
#21884=CARTESIAN_POINT ( 'NONE',  ( 8.962745559623000347, -5.445226602819000838, 7.703375344019999460 ) ) ;
#21886=CARTESIAN_POINT ( 'NONE',  ( 11.09999999999999964, -5.350000000000000533, -7.500000000000000000 ) ) ;
#21896=ORIENTED_EDGE ( 'NONE', *, *, #7524, .F. ) ;
#21899=CARTESIAN_POINT ( 'NONE',  ( 8.415400305754983989, -2.414631728478774164, 8.215148636469683296 ) ) ;
#21910=EDGE_CURVE ( 'NONE', #54965, #67391, #21514, .T. ) ;
#21911=EDGE_LOOP ( 'NONE', ( #65592, #49448, #67897, #26751 ) ) ;
#21912=CARTESIAN_POINT ( 'NONE',  ( 10.07314899745999881, -5.167567567567999731, -6.822293592207000934 ) ) ;
#21913=SURFACE_STYLE_FILL_AREA ( #1292 ) ;
#21936=ADVANCED_FACE ( 'NONE', ( #61950 ), #13384, .T. ) ;
#21942=CARTESIAN_POINT ( 'NONE',  ( 10.21238410957999854, -4.072568653311000375, -8.861841462475000597 ) ) ;
#21950=CARTESIAN_POINT ( 'NONE',  ( 10.11094409420000062, -5.100000000000000533, -6.571291218949999902 ) ) ;
#21954=VECTOR ( 'NONE', #1639, 1000.000000000000000 ) ;
#21957=VECTOR ( 'NONE', #63966, 1000.000000000000000 ) ;
#21969=VECTOR ( 'NONE', #650, 1000.000000000000000 ) ;
#21977=AXIS2_PLACEMENT_3D ( 'NONE', #16152, #1114, #49343 ) ;
#21980=CARTESIAN_POINT ( 'NONE',  ( 10.79499900793999956, -3.503951165873000040, 6.168577387731000172 ) ) ;
#21981=CARTESIAN_POINT ( 'NONE',  ( 7.962144353208000069, -4.874569256861000177, 6.119503992241999590 ) ) ;
#21985=CARTESIAN_POINT ( 'NONE',  ( 10.25880564679000173, -2.491773655925000330, -7.289938045981000592 ) ) ;
#21986=CARTESIAN_POINT ( 'NONE',  ( 7.805655517671931776, -4.414680877279917759, 9.189650186020678291 ) ) ;
#21987=CARTESIAN_POINT ( 'NONE',  ( 10.12549839661999940, -5.788806995403000144, 7.335561828691000485 ) ) ;
#21993=ORIENTED_EDGE ( 'NONE', *, *, #224, .F. ) ;
#21997=EDGE_CURVE ( 'NONE', #49573, #25777, #27338, .T. ) ;
#22003=CARTESIAN_POINT ( 'NONE',  ( 7.790629440376999781, -3.416208448044999901, 6.162501393933999871 ) ) ;
#22004=FACE_OUTER_BOUND ( 'NONE', #47052, .T. ) ;
#22012=CARTESIAN_POINT ( 'NONE',  ( 10.96876739532000045, -2.333349849211999949, 6.524062020538999640 ) ) ;
#22023=LINE ( 'NONE', #27632, #47039 ) ;
#22045=B_SPLINE_CURVE_WITH_KNOTS ( 'NONE', 3,
 ( #10479, #30782, #30443, #35689 ),
 .UNSPECIFIED., .F., .F.,
 ( 4, 4 ),
 ( 0.000000000000000000, 1.000000000000000000 ),
 .UNSPECIFIED. ) ;
#22051=ORIENTED_EDGE ( 'NONE', *, *, #59479, .F. ) ;
#22054=CARTESIAN_POINT ( 'NONE',  ( 9.383148997457999130, -5.167567567567999731, 6.822293592207000934 ) ) ;
#22065=CARTESIAN_POINT ( 'NONE',  ( 9.762850396985012225, -2.920672817053836745, -8.329416270159347491 ) ) ;
#22071=B_SPLINE_CURVE_WITH_KNOTS ( 'NONE', 3,
 ( #18592, #34679, #7056, #28391 ),
 .UNSPECIFIED., .F., .F.,
 ( 4, 4 ),
 ( 0.000000000000000000, 1.000000000000000000 ),
 .UNSPECIFIED. ) ;
#22072=VECTOR ( 'NONE', #26075, 1000.000000000000227 ) ;
#22074=CARTESIAN_POINT ( 'NONE',  ( 10.52384314678999999, -5.441919393629000012, -7.989634081859001036 ) ) ;
#22076=B_SPLINE_SURFACE_WITH_KNOTS ( 'NONE', 3, 3, ( 
 ( #37654, #58986, #32422, #53737 ),
 ( #60365, #56495, #28561, #45328 ),
 ( #7918, #13175, #66638, #55121 ),
 ( #24683, #65940, #66288, #18413 ),
 ( #8258, #3006, #61056, #39047 ) ),
 .UNSPECIFIED., .F., .F., .F.,
 ( 4, 1, 4 ),
 ( 4, 4 ),
 ( 0.4073867043412000011, 0.4166666666666999919, 0.4317812135810999985 ),
 ( -0.1884351840153000168, 1.188534893118999847 ),
 .UNSPECIFIED. ) ;
#22078=CARTESIAN_POINT ( 'NONE',  ( 11.09999999999999964, -5.350000000000000533, -7.500000000000000000 ) ) ;
#22082=ORIENTED_EDGE ( 'NONE', *, *, #18147, .F. ) ;
#22085=VERTEX_POINT ( 'NONE', #54816 ) ;
#22096=CARTESIAN_POINT ( 'NONE',  ( 10.70780617489000086, -5.157482071823000780, -6.267811103859000532 ) ) ;
#22107=VECTOR ( 'NONE', #14348, 1000.000000000000000 ) ;
#22124=CARTESIAN_POINT ( 'NONE',  ( 10.15786958814999963, -4.213496663054999480, -5.822956951053000374 ) ) ;
#22130=CARTESIAN_POINT ( 'NONE',  ( 10.90000000000000036, -2.899999999999999911, 6.414037451299000381 ) ) ;
#22142=CARTESIAN_POINT ( 'NONE',  ( 9.194602547868999665, -5.157768569202000108, 8.637845986715998237 ) ) ;
#22146=CARTESIAN_POINT ( 'NONE',  ( 10.00638553269999953, -5.119272496996000399, 8.420388242270998802 ) ) ;
#22169=ORIENTED_EDGE ( 'NONE', *, *, #32749, .T. ) ;
#22172=ORIENTED_EDGE ( 'NONE', *, *, #42774, .T. ) ;
#22180=CARTESIAN_POINT ( 'NONE',  ( 10.52314899745999988, -5.167567567567999731, -6.822293592207000934 ) ) ;
#22183=CARTESIAN_POINT ( 'NONE',  ( 10.87522165821000009, -4.831071966430999787, 6.312786525516999703 ) ) ;
#22188=EDGE_CURVE ( 'NONE', #23757, #52126, #25062, .T. ) ;
#22191=CARTESIAN_POINT ( 'NONE',  ( 10.27366694038000006, -3.065543393453000309, -8.487918777453998587 ) ) ;
#22200=CARTESIAN_POINT ( 'NONE',  ( 9.327427652207148867, -3.945165805631096312, 9.238792170091185696 ) ) ;
#22202=CARTESIAN_POINT ( 'NONE',  ( 8.245455708338628398, -4.975154674665282606, 6.309433999826808304 ) ) ;
#22207=CARTESIAN_POINT ( 'NONE',  ( 11.27109998545999936, -5.469594811916000054, 8.504700858852999090 ) ) ;
#22217=CARTESIAN_POINT ( 'NONE',  ( 9.447848023450999833, -5.447470167531999863, 7.431328114251999573 ) ) ;
#22219=CARTESIAN_POINT ( 'NONE',  ( 7.833769353207999941, -2.583664704444999849, 6.684748541034000624 ) ) ;
#22220=LINE ( 'NONE', #2284, #41585 ) ;
#22228=CARTESIAN_POINT ( 'NONE',  ( 10.34286678428582640, -2.713835889960352965, -7.027064066396518704 ) ) ;
#22233=FACE_OUTER_BOUND ( 'NONE', #31646, .T. ) ;
#22241=DIRECTION ( 'NONE',  ( -1.000000000000000000, 0.000000000000000000, 0.000000000000000000 ) ) ;
#22243=CARTESIAN_POINT ( 'NONE',  ( 7.110997236279914091, -3.823158075381482668, 8.850159282918328429 ) ) ;
#22250=CARTESIAN_POINT ( 'NONE',  ( 8.449546238384577634, -2.260405780409438403, 7.505456740821800032 ) ) ;
#22253=ORIENTED_EDGE ( 'NONE', *, *, #20203, .T. ) ;
#22261=CARTESIAN_POINT ( 'NONE',  ( 10.53010726722364510, -2.706054758365612489, -8.716665077408118023 ) ) ;
#22265=CARTESIAN_POINT ( 'NONE',  ( 9.433148997456999751, -5.167567567567999731, 6.822293592207000934 ) ) ;
#22266=ORIENTED_EDGE ( 'NONE', *, *, #10476, .T. ) ;
#22274=ORIENTED_EDGE ( 'NONE', *, *, #68827, .T. ) ;
#22279=CYLINDRICAL_SURFACE ( 'NONE', #11849, 1.350000000000000089 ) ;
#22292=CARTESIAN_POINT ( 'NONE',  ( 9.675541251098000117, -4.656741678598999457, -8.653222148251000334 ) ) ;
#22297=CARTESIAN_POINT ( 'NONE',  ( 10.88314899746000108, -5.167567567567999731, 6.822293592207000934 ) ) ;
#22316=CARTESIAN_POINT ( 'NONE',  ( 10.60664092702312189, -5.179495029648551352, -8.179803431736287322 ) ) ;
#22321=VERTEX_POINT ( 'NONE', #45711 ) ;
#22325=CARTESIAN_POINT ( 'NONE',  ( 10.07101719722999889, -4.042170815906999337, 8.920201479886998186 ) ) ;
#22332=CARTESIAN_POINT ( 'NONE',  ( 10.97819314679000158, -5.476828481365000556, -7.128717489481000591 ) ) ;
#22334=CARTESIAN_POINT ( 'NONE',  ( 7.778522546713435126, -4.944928104213000886, 8.960707585029377142 ) ) ;
#22335=CARTESIAN_POINT ( 'NONE',  ( 11.08492081570999943, -3.668392767032000013, 5.558160538745999801 ) ) ;
#22354=CARTESIAN_POINT ( 'NONE',  ( 9.459504440379001622, -5.445226602819000838, 7.703375344019999460 ) ) ;
#22363=CARTESIAN_POINT ( 'NONE',  ( 7.975339216757299177, -5.350090185752664595, 7.499980949462679014 ) ) ;
#22371=CARTESIAN_POINT ( 'NONE',  ( 8.225195096046189036, -2.649880853682571313, 7.500010424662522546 ) ) ;
#22378=FACE_OUTER_BOUND ( 'NONE', #49146, .T. ) ;
#22385=B_SPLINE_SURFACE_WITH_KNOTS ( 'NONE', 3, 3, ( 
 ( #54867, #48237, #54166, #23044, #27265, #22003, #44394, #17816, #39131, #12565, #53826, #42992, #64301, #16419, #37747, #59074, #11174, #38438, #6266, #5924, #48588, #59760, #38085, #691, #43351, #64651, #59411, #11511, #27607, #48935, #1043, #22354, #43693, #17104, #14290 ),
 ( #40503, #2081, #44737, #35619, #35273, #61150, #13268, #50316, #19526, #8353, #24433, #29699, #34594, #8011, #45077, #56590, #40174, #51342, #2760, #61828, #51001, #30039, #13609, #3435, #60802, #13947, #55562, #66383, #3099, #2415, #66729, #8696, #7312, #55908, #24772 ),
 ( #23398, #23739, #28654, #39829, #49966, #46099, #67405, #45419, #45758, #29348, #50660, #66035, #34931, #61491, #40847, #62168, #24086, #18159, #39481, #12914, #34242, #18505, #56246, #67067, #7663, #18848, #29009, #19180, #15654, #52367, #15992, #56930, #31057, #26150, #9028 ),
 ( #19868, #69135, #46443, #41199, #25800, #47133, #36987, #68783, #4460, #46785, #26495, #30368, #3775, #14627, #5162, #52712, #47825, #20208, #57962, #51677, #68090, #9712, #62508, #62846, #47475, #58299, #31396, #63880, #25111, #57607, #4809, #20899, #42238, #67744, #63543 ) ),
 .UNSPECIFIED., .F., .F., .F.,
 ( 4, 4 ),
 ( 4, 1, 1, 1, 1, 1, 1, 1, 1, 1, 1, 1, 1, 1, 1, 1, 1, 1, 1, 1, 1, 1, 1, 1, 1, 1, 1, 1, 1, 1, 1, 1, 4 ),
 ( -0.1039086239011999951, 1.103908623900999864 ),
 ( -0.02000000000000000042, 0.01250000000000000069, 0.04499999999999999833, 0.07749999999999999944, 0.1100000000000000006, 0.1424999999999999878, 0.1749999999999999889, 0.2074999999999999900, 0.2399999999999999911, 0.2725000000000000200, 0.3049999999999999933, 0.3375000000000000222, 0.3699999999999999956, 0.4025000000000000244, 0.4349999999999999978, 0.4675000000000000266, 0.5000000000000000000, 0.5324999999999999734, 0.5649999999999999467, 0.5975000000000000311, 0.6300000000000000044, 0.6624999999999999778, 0.6949999999999999512, 0.7275000000000000355, 0.7600000000000000089, 0.7924999999999999822, 0.8249999999999999556, 0.8575000000000000400, 0.8900000000000000133, 0.9224999999999999867, 0.9549999999999999600, 0.9875000000000000444, 1.020000000000000018 ),
 .UNSPECIFIED. ) ;
#22416=ADVANCED_FACE ( 'NONE', ( #42186 ), #21334, .F. ) ;
#22421=AXIS2_PLACEMENT_3D ( 'NONE', #44266, #11051, #65561 ) ;
#22423=CARTESIAN_POINT ( 'NONE',  ( 10.01676935320999995, -4.324998011277000565, -9.154075058362000306 ) ) ;
#22424=DIRECTION ( 'NONE',  ( 0.7071067811865475727, 0.7071067811865475727, 0.000000000000000000 ) ) ;
#22433=VERTEX_POINT ( 'NONE', #53358 ) ;
#22442=CARTESIAN_POINT ( 'NONE',  ( 10.66852499011999988, -4.435470817312999969, -5.866470266317000082 ) ) ;
#22450=CARTESIAN_POINT ( 'NONE',  ( 10.26390815928000144, -4.634708712637999994, 4.688349230856999839 ) ) ;
#22451=CARTESIAN_POINT ( 'NONE',  ( 10.69674062800671166, -2.930427565545544066, 5.070473834605100372 ) ) ;
#22464=CARTESIAN_POINT ( 'NONE',  ( 9.947300131853999972, -4.892806669161000599, -9.067746434455999704 ) ) ;
#22465=EDGE_CURVE ( 'NONE', #31041, #16661, #26447, .T. ) ;
#22466=EDGE_CURVE ( 'NONE', #51230, #873, #60307, .T. ) ;
#22468=CARTESIAN_POINT ( 'NONE',  ( 9.472537864290000442, -2.899999999999999911, -6.571291218949999902 ) ) ;
#22470=CARTESIAN_POINT ( 'NONE',  ( 8.316694573732000606, -2.898380360490000029, 6.611503418275999522 ) ) ;
#22475=CARTESIAN_POINT ( 'NONE',  ( 8.576923877145999242, -3.399999999999999911, 5.924121105096999962 ) ) ;
#22480=CARTESIAN_POINT ( 'NONE',  ( 11.08388352126999976, -2.665717300265999956, 4.955856577691999831 ) ) ;
#22484=CARTESIAN_POINT ( 'NONE',  ( 9.781666627457001439, -5.464740618746000145, 8.817321229216000589 ) ) ;
#22487=CARTESIAN_POINT ( 'NONE',  ( 9.261668853699999815, -2.944250413017999612, 6.507387951280999339 ) ) ;
#22488=CARTESIAN_POINT ( 'NONE',  ( 9.938536681611822132, -2.240210568168245597, 7.748637171123511358 ) ) ;
#22494=CARTESIAN_POINT ( 'NONE',  ( 8.896907940197010589, -2.871668805576999883, -6.751846157836005169 ) ) ;
#22510=FACE_OUTER_BOUND ( 'NONE', #12742, .T. ) ;
#22514=CARTESIAN_POINT ( 'NONE',  ( 8.802620559624999785, -3.975070057433999438, 9.483761758588999058 ) ) ;
#22521=ADVANCED_FACE ( 'NONE', ( #17328 ), #12088, .T. ) ;
#22542=VERTEX_POINT ( 'NONE', #39010 ) ;
#22548=B_SPLINE_CURVE_WITH_KNOTS ( 'NONE', 3,
 ( #45772, #9722, #62521, #4130, #13960, #3115, #45432, #50677, #19884, #19542, #3448, #40189 ),
 .UNSPECIFIED., .F., .F.,
 ( 4, 2, 2, 2, 2, 4 ),
 ( 0.000000000000000000, 0.2500000000000020539, 0.3750000000000017208, 0.4375000000000028866, 0.5000000000000039968, 1.000000000000000000 ),
 .UNSPECIFIED. ) ;
#22549=CARTESIAN_POINT ( 'NONE',  ( 10.02990552045999983, -2.506467134554999809, 6.215414506835998942 ) ) ;
#22559=CARTESIAN_POINT ( 'NONE',  ( 7.267328493169560311, -2.819480080816116896, 6.820320496870126981 ) ) ;
#22561=CARTESIAN_POINT ( 'NONE',  ( 7.358058059621999547, -4.561648098548999997, 6.153050355516999304 ) ) ;
#22564=CARTESIAN_POINT ( 'NONE',  ( 10.29353630810780018, -2.899999999999999911, 6.665341197265856721 ) ) ;
#22573=CARTESIAN_POINT ( 'NONE',  ( 7.968183059622999664, -2.280579276705999803, 6.510290672242000198 ) ) ;
#22577=ADVANCED_FACE ( 'NONE', ( #59977 ), #11728, .F. ) ;
#22582=CONICAL_SURFACE ( 'NONE', #51583, 0.4311160744474001327, 0.7853981633972997312 ) ;
#22584=VERTEX_POINT ( 'NONE', #33767 ) ;
#22586=DIRECTION ( 'NONE',  ( -1.000000000000000000, -5.693641285695000080E-09, 1.583067011023000022E-09 ) ) ;
#22593=CARTESIAN_POINT ( 'NONE',  ( 8.380370550424483866, -2.884289483078743555, 8.834819442766946196 ) ) ;
#22598=CARTESIAN_POINT ( 'NONE',  ( 10.18239901426000138, -2.607725299334000102, 7.783410967795999724 ) ) ;
#22607=B_SPLINE_CURVE_WITH_KNOTS ( 'NONE', 3,
 ( #6419, #21812, #44201, #43844 ),
 .UNSPECIFIED., .F., .F.,
 ( 4, 4 ),
 ( 0.8747102644739949140, 1.000000000000000000 ),
 .UNSPECIFIED. ) ;
#22609=CARTESIAN_POINT ( 'NONE',  ( 9.440795537696432760, -5.100000000000000533, 6.662590550605512085 ) ) ;
#22614=VECTOR ( 'NONE', #27831, 999.9999999999998863 ) ;
#22633=CARTESIAN_POINT ( 'NONE',  ( 10.49937632700000023, -2.985311165300999825, -6.358653174814000053 ) ) ;
#22643=DIRECTION ( 'NONE',  ( 0.000000000000000000, 0.000000000000000000, -1.000000000000000000 ) ) ;
#22651=CARTESIAN_POINT ( 'NONE',  ( 8.913566940379999082, -2.550589632307000088, 8.854674225901000284 ) ) ;
#22652=CARTESIAN_POINT ( 'NONE',  ( 9.663732219486000474, -2.297586052318000061, -7.360088033824999876 ) ) ;
#22654=EDGE_CURVE ( 'NONE', #64219, #35557, #24393, .T. ) ;
#22670=CARTESIAN_POINT ( 'NONE',  ( 9.646285452541999206, -2.591464128784999765, 6.760053199270999791 ) ) ;
#22676=CARTESIAN_POINT ( 'NONE',  ( 10.16821935321000048, -2.330398934821000356, -7.267462182607999921 ) ) ;
#22677=CARTESIAN_POINT ( 'NONE',  ( 7.751324872093176666, -5.382780984143693992, 8.555630740302449411 ) ) ;
#22682=ORIENTED_EDGE ( 'NONE', *, *, #14369, .F. ) ;
#22694=CARTESIAN_POINT ( 'NONE',  ( 8.960616452296999768, -2.899999999999999911, 6.279946362737000243 ) ) ;
#22702=LINE ( 'NONE', #44399, #15280 ) ;
#22718=CARTESIAN_POINT ( 'NONE',  ( 11.09999999999999964, -2.649999999999999911, 7.500000000000000000 ) ) ;
#22722=ADVANCED_FACE ( 'NONE', ( #66598 ), #62044, .T. ) ;
#22733=CARTESIAN_POINT ( 'NONE',  ( 5.700000000399000122, -0.2999999996014000025, -3.150000003758000044 ) ) ;
#22735=ORIENTED_EDGE ( 'NONE', *, *, #56185, .T. ) ;
#22740=DIRECTION ( 'NONE',  ( 0.000000000000000000, 0.000000000000000000, -1.000000000000000000 ) ) ;
#22746=EDGE_CURVE ( 'NONE', #49595, #48149, #2289, .T. ) ;
#22757=CARTESIAN_POINT ( 'NONE',  ( 8.571413182548997867, -4.600000000000999734, 5.927302706106000407 ) ) ;
#22769=CARTESIAN_POINT ( 'NONE',  ( 11.12964314679000033, -3.869080819553999628, -9.017146989745999264 ) ) ;
#22789=CARTESIAN_POINT ( 'NONE',  ( 11.07336076184000007, -2.375557098086999996, -8.393541296344000813 ) ) ;
#22790=CIRCLE ( 'NONE', #40657, 10.55000000000000426 ) ;
#22793=CARTESIAN_POINT ( 'NONE',  ( 10.75905508291875989, -2.921956017810039441, -5.082778843723144924 ) ) ;
#22798=CARTESIAN_POINT ( 'NONE',  ( 11.09999999999999964, -7.940796613052000019, 6.945951997396999644 ) ) ;
#22799=CARTESIAN_POINT ( 'NONE',  ( 10.45746920027980487, -3.052701587494784263, 4.998914760967365645 ) ) ;
#22803=CARTESIAN_POINT ( 'NONE',  ( 9.834153701540001791, -5.173926576843999925, 8.813045240277000758 ) ) ;
#22817=CARTESIAN_POINT ( 'NONE',  ( 10.27571314244999989, -5.689440078020999714, -7.562019725378000601 ) ) ;
#22819=CARTESIAN_POINT ( 'NONE',  ( 10.53706676393821162, -5.286158710546942530, -7.027080267280065407 ) ) ;
#22827=CARTESIAN_POINT ( 'NONE',  ( 10.75590824504000054, -2.705649759953999922, 4.786982446041000649 ) ) ;
#22828=CARTESIAN_POINT ( 'NONE',  ( 8.062814847549001129, -3.480055400096998319, 6.228346641557002350 ) ) ;
#22836=CARTESIAN_POINT ( 'NONE',  ( 10.31668414895000119, -3.819528725844000494, 6.062183754159999438 ) ) ;
#22837=CARTESIAN_POINT ( 'NONE',  ( 9.685974049303974098, -5.723140299379433138, 7.204273367287987284 ) ) ;
#22852=DIRECTION ( 'NONE',  ( 0.000000000000000000, -1.000000000000000000, 0.000000000000000000 ) ) ;
#22864=CARTESIAN_POINT ( 'NONE',  ( 8.417495559623999313, -2.029110377978999846, 7.726994002375999315 ) ) ;
#22875=EDGE_LOOP ( 'NONE', ( #40081, #4384, #47645 ) ) ;
#22904=CARTESIAN_POINT ( 'NONE',  ( 9.637133777480245911, -2.899999999999999911, -6.201439514950156884 ) ) ;
#22906=CARTESIAN_POINT ( 'NONE',  ( 8.604019353210000887, -5.165500668528999917, 8.645534272955000432 ) ) ;
#22910=CARTESIAN_POINT ( 'NONE',  ( 8.736375959668992053, -5.159793961343003055, -6.817201505920002624 ) ) ;
#22920=CARTESIAN_POINT ( 'NONE',  ( 7.903995559621998623, -2.095727472214000020, 8.056487497515000484 ) ) ;
#22942=CARTESIAN_POINT ( 'NONE',  ( 11.09999999999999964, -2.700000000000000178, 5.160242730440000258 ) ) ;
#22953=CARTESIAN_POINT ( 'NONE',  ( 8.793505787816332742, -5.100000000000000533, 6.515557531858333640 ) ) ;
#22955=DIRECTION ( 'NONE',  ( 1.000000000000000000, 1.736057635237000010E-14, 9.258974054599999947E-14 ) ) ;
#22958=EDGE_CURVE ( 'NONE', #29557, #61812, #26874, .T. ) ;
#22978=VECTOR ( 'NONE', #12980, 1000.000000000000000 ) ;
#22981=CARTESIAN_POINT ( 'NONE',  ( 10.06728329455999926, -4.192861215955000276, -5.985050974557999837 ) ) ;
#22982=VECTOR ( 'NONE', #63886, 1000.000000000000000 ) ;
#22999=ADVANCED_FACE ( 'NONE', ( #40462 ), #61792, .T. ) ;
#23000=ORIENTED_EDGE ( 'NONE', *, *, #564, .F. ) ;
#23001=CARTESIAN_POINT ( 'NONE',  ( 7.667605646792000407, -5.638700495537999124, 8.266402903491000487 ) ) ;
#23002=CARTESIAN_POINT ( 'NONE',  ( 9.837156140204001531, -5.811247906278000031, -7.978055797018001272 ) ) ;
#23006=B_SPLINE_CURVE_WITH_KNOTS ( 'NONE', 3,
 ( #67745, #10404, #68784, #36640, #57963 ),
 .UNSPECIFIED., .F., .F.,
 ( 4, 1, 4 ),
 ( 0.000000000000000000, 0.5000000000000000000, 1.000000000000000000 ),
 .UNSPECIFIED. ) ;
#23008=FACE_OUTER_BOUND ( 'NONE', #50987, .T. ) ;
#23019=CARTESIAN_POINT ( 'NONE',  ( 11.18706725482999964, -3.186788126275999833, 6.232699537089999353 ) ) ;
#23022=CARTESIAN_POINT ( 'NONE',  ( 8.193904585095999948, -3.399974355387999747, 6.145257543266000155 ) ) ;
#23025=CARTESIAN_POINT ( 'NONE',  ( 8.093307509540114353, -4.415759437142675381, 5.811247418746839699 ) ) ;
#23026=CARTESIAN_POINT ( 'NONE',  ( 9.939319226872999735, -2.638101016021999978, 6.328632621050000573 ) ) ;
#23043=ORIENTED_EDGE ( 'NONE', *, *, #55635, .T. ) ;
#23044=CARTESIAN_POINT ( 'NONE',  ( 7.662254440376999653, -2.688354259407999880, 8.140021027181001401 ) ) ;
#23046=ORIENTED_EDGE ( 'NONE', *, *, #47435, .T. ) ;
#23047=CARTESIAN_POINT ( 'NONE',  ( 10.06646012162292969, -2.291509473315214596, -8.026256863629807725 ) ) ;
#23049=CARTESIAN_POINT ( 'NONE',  ( 11.02419555961999897, -2.407899345275000158, -8.439548421502999886 ) ) ;
#23052=CARTESIAN_POINT ( 'NONE',  ( 8.121343566036618000, -3.646810248691512601, 8.848457998379473111 ) ) ;
#23062=DIRECTION ( 'NONE',  ( 1.000000000000000000, 0.000000000000000000, 0.000000000000000000 ) ) ;
#23072=CARTESIAN_POINT ( 'NONE',  ( 8.924662153698962541, -5.350575487761723537, 7.500021879703682615 ) ) ;
#23076=CARTESIAN_POINT ( 'NONE',  ( 11.09999999999999964, -4.000000000000000000, 7.500000000000000000 ) ) ;
#23090=DIRECTION ( 'NONE',  ( 0.9925497095595060548, 0.000000000000000000, 0.1218403629892008122 ) ) ;
#23094=VERTEX_POINT ( 'NONE', #8993 ) ;
#23107=DIRECTION ( 'NONE',  ( 0.000000000000000000, -1.000000000000000000, 0.000000000000000000 ) ) ;
#23118=CARTESIAN_POINT ( 'NONE',  ( 10.46297944037999983, -3.993164663709000362, -6.140164943008000087 ) ) ;
#23126=CARTESIAN_POINT ( 'NONE',  ( 11.02939238023000001, -8.053283849414000883, -6.898628641089999292 ) ) ;
#23131=ORIENTED_EDGE ( 'NONE', *, *, #66488, .F. ) ;
#23136=DIRECTION ( 'NONE',  ( 1.000000000000000000, 0.000000000000000000, 0.000000000000000000 ) ) ;
#23140=CARTESIAN_POINT ( 'NONE',  ( 10.00074484908000194, -2.373896846742000299, -7.962434077545999855 ) ) ;
#23143=ORIENTED_EDGE ( 'NONE', *, *, #50757, .T. ) ;
#23149=CARTESIAN_POINT ( 'NONE',  ( 11.04384236319999957, -5.374613432488000164, -5.035088906224999938 ) ) ;
#23152=CARTESIAN_POINT ( 'NONE',  ( 10.39106278671000005, -4.025320977579999848, 9.261121875182000807 ) ) ;
#23165=CARTESIAN_POINT ( 'NONE',  ( 10.86493091395000121, -4.678465004315999209, -9.048463592221999363 ) ) ;
#23170=CARTESIAN_POINT ( 'NONE',  ( 9.306727112333998519, -4.009302068291999532, -9.043024413115999138 ) ) ;
#23176=CARTESIAN_POINT ( 'NONE',  ( 10.33091365668000172, -3.119355846288000222, 4.717868057528999515 ) ) ;
#23177=CARTESIAN_POINT ( 'NONE',  ( 9.906851002540999929, -2.832432432432000269, -6.822293592207000934 ) ) ;
#23181=CARTESIAN_POINT ( 'NONE',  ( 10.90374822854000136, -3.726845778959999578, 5.900452123196999743 ) ) ;
#23186=VECTOR ( 'NONE', #8669, 1000.000000000000114 ) ;
#23187=CARTESIAN_POINT ( 'NONE',  ( 10.09697182628999990, -5.253379538902000156, 8.530665717066000298 ) ) ;
#23188=CARTESIAN_POINT ( 'NONE',  ( 9.694121230991363802, -5.744981173682874420, 7.383335460396494909 ) ) ;
#23191=ORIENTED_EDGE ( 'NONE', *, *, #24620, .T. ) ;
#23199=CARTESIAN_POINT ( 'NONE',  ( 8.616332388160998335, -5.167567399848000065, -6.822293593032000558 ) ) ;
#23201=CARTESIAN_POINT ( 'NONE',  ( 5.500000000000000000, 0.8000000000000000444, -3.149999999999999911 ) ) ;
#23217=EDGE_LOOP ( 'NONE', ( #20687, #40664, #12402, #30591, #985, #65427, #1382, #18465, #12870 ) ) ;
#23218=CARTESIAN_POINT ( 'NONE',  ( 10.42819717211483521, -5.125396288440269288, 6.749639981106747122 ) ) ;
#23226=CARTESIAN_POINT ( 'NONE',  ( 11.06666666666870746, -2.480181672121660519, 7.732127511715526147 ) ) ;
#23228=CARTESIAN_POINT ( 'NONE',  ( 10.81316193496000011, -3.756072284922999938, 6.071597915422999314 ) ) ;
#23244=CARTESIAN_POINT ( 'NONE',  ( 9.474491361279490320, -2.332153331583475264, 6.968217119213045763 ) ) ;
#23245=ORIENTED_EDGE ( 'NONE', *, *, #27877, .T. ) ;
#23251=B_SPLINE_CURVE_WITH_KNOTS ( 'NONE', 3,
 ( #42034, #58793, #10552, #64362 ),
 .UNSPECIFIED., .F., .F.,
 ( 4, 4 ),
 ( 0.000000000000000000, 1.000000000000000000 ),
 .UNSPECIFIED. ) ;
#23252=CARTESIAN_POINT ( 'NONE',  ( 11.02286109245999945, -2.398753588646000079, 6.352476128646999065 ) ) ;
#23260=CARTESIAN_POINT ( 'NONE',  ( 10.13050497920000126, -3.092053006542000215, 8.629388195475000245 ) ) ;
#23262=CARTESIAN_POINT ( 'NONE',  ( 8.256683059623998844, -2.876278577719999952, 6.568889245344999850 ) ) ;
#23269=EDGE_CURVE ( 'NONE', #53475, #60701, #38184, .T. ) ;
#23271=CARTESIAN_POINT ( 'NONE',  ( 10.90291315457000110, -5.099848460227999425, 5.141818958950999274 ) ) ;
#23272=CARTESIAN_POINT ( 'NONE',  ( 11.09999999999999964, -5.538898460221000519, 7.685179721164000277 ) ) ;
#23282=FACE_OUTER_BOUND ( 'NONE', #2613, .T. ) ;
#23285=CARTESIAN_POINT ( 'NONE',  ( 8.571413182548997867, -4.600000000000999734, 5.927302706106000407 ) ) ;
#23296=CARTESIAN_POINT ( 'NONE',  ( 8.575831600094877771, -4.020817762796284889, 5.760477547183362468 ) ) ;
#23298=VECTOR ( 'NONE', #27200, 1000.000000000000000 ) ;
#23302=CARTESIAN_POINT ( 'NONE',  ( 9.903944471677000649, -5.205019707614999547, 6.747219600580999455 ) ) ;
#23304=CARTESIAN_POINT ( 'NONE',  ( 9.481861110199060860, -5.015380455770686474, 8.392903197087751010 ) ) ;
#23307=ORIENTED_EDGE ( 'NONE', *, *, #43087, .T. ) ;
#23309=CARTESIAN_POINT ( 'NONE',  ( 11.09999999999999964, -2.899999999999999911, -4.336547745386999608 ) ) ;
#23313=VERTEX_POINT ( 'NONE', #45522 ) ;
#23320=ADVANCED_FACE ( 'NONE', ( #2515 ), #13018, .F. ) ;
#23330=ORIENTED_EDGE ( 'NONE', *, *, #16823, .F. ) ;
#23334=CARTESIAN_POINT ( 'NONE',  ( 11.08752429429999964, -2.871531501602999636, -6.302910744985999791 ) ) ;
#23339=CARTESIAN_POINT ( 'NONE',  ( 10.08070436339981768, -5.349944892048520195, -7.768717962862259796 ) ) ;
#23342=CARTESIAN_POINT ( 'NONE',  ( 10.75046352948140438, -3.823292445202751466, -8.850187295431151568 ) ) ;
#23354=CARTESIAN_POINT ( 'NONE',  ( 7.239688980126000040, -4.389298280625000714, 9.135255728583000945 ) ) ;
#23362=CARTESIAN_POINT ( 'NONE',  ( 10.57538794102227264, -5.349775832304747070, -7.676723066621575775 ) ) ;
#23371=CARTESIAN_POINT ( 'NONE',  ( 10.50244460374000077, -2.268915328469999881, 7.824865002012999504 ) ) ;
#23376=CARTESIAN_POINT ( 'NONE',  ( 10.99305444037999990, -4.495427106425000652, -6.233607450113000326 ) ) ;
#23377=CARTESIAN_POINT ( 'NONE',  ( 7.917165897655459084, -2.404019642809257729, 8.192082336436831369 ) ) ;
#23378=CARTESIAN_POINT ( 'NONE',  ( 11.08992739829000129, -5.210546653347999602, 8.327600405525998895 ) ) ;
#23386=ORIENTED_EDGE ( 'NONE', *, *, #18427, .F. ) ;
#23397=EDGE_LOOP ( 'NONE', ( #299, #6198, #27053, #37282 ) ) ;
#23398=CARTESIAN_POINT ( 'NONE',  ( 7.352706853207999771, -4.773080213113000347, 8.927399220053999329 ) ) ;
#23404=EDGE_CURVE ( 'NONE', #25841, #57495, #171, .T. ) ;
#23405=CARTESIAN_POINT ( 'NONE',  ( 5.500000000627999874, -0.4999999993719999591, -3.150000005921999691 ) ) ;
#23408=CARTESIAN_POINT ( 'NONE',  ( 10.91307648679999964, -2.096298111716999646, 7.827187677719999570 ) ) ;
#23442=CARTESIAN_POINT ( 'NONE',  ( 9.074379440379999551, -3.981661727120999750, 8.959239802162999311 ) ) ;
#23445=VECTOR ( 'NONE', #40175, 1000.000000000000000 ) ;
#23455=CARTESIAN_POINT ( 'NONE',  ( 9.416239699516157913, -5.342737953096846404, 7.360744645781648998 ) ) ;
#23461=DIRECTION ( 'NONE',  ( 1.636082834842964734E-07, -0.7071067247530858912, -0.7071068376199858285 ) ) ;
#23466=CARTESIAN_POINT ( 'NONE',  ( 8.486008579191000933, -3.399999999999999911, 5.976611076844000614 ) ) ;
#23469=CARTESIAN_POINT ( 'NONE',  ( 10.41104069048442149, -5.348816829097293279, 7.263526753701751382 ) ) ;
#23471=CARTESIAN_POINT ( 'NONE',  ( 10.99239898671677906, -5.801279784331776490, 4.969949983916245095 ) ) ;
#23476=ORIENTED_EDGE ( 'NONE', *, *, #27557, .F. ) ;
#23489=CARTESIAN_POINT ( 'NONE',  ( 10.62924380535000068, -3.609488729914999805, -5.855142811286000004 ) ) ;
#23492=CARTESIAN_POINT ( 'NONE',  ( 10.98768577056000062, -2.700436730051000378, -4.945210085382000464 ) ) ;
#23494=CARTESIAN_POINT ( 'NONE',  ( 10.27736255359000062, -4.572640260524000411, 5.004092596557000228 ) ) ;
#23495=FACE_OUTER_BOUND ( 'NONE', #3084, .T. ) ;
#23498=CARTESIAN_POINT ( 'NONE',  ( 10.66951732929000052, -4.592671928130000580, 5.841406818427000047 ) ) ;
#23510=CARTESIAN_POINT ( 'NONE',  ( 11.09999999999999964, -6.593648099371000271, -5.598803483715999896 ) ) ;
#23514=CARTESIAN_POINT ( 'NONE',  ( 9.040134009213000255, -5.099406281193999746, -6.669356233738001016 ) ) ;
#23517=EDGE_CURVE ( 'NONE', #61050, #21198, #63293, .T. ) ;
#23521=CARTESIAN_POINT ( 'NONE',  ( 8.241912900173000267, -4.599999999999999645, 6.117539782833000928 ) ) ;
#23524=VERTEX_POINT ( 'NONE', #26254 ) ;
#23527=CARTESIAN_POINT ( 'NONE',  ( 10.00137895011999944, -3.855365288061999962, 5.709482985498999241 ) ) ;
#23530=AXIS2_PLACEMENT_3D ( 'NONE', #3894, #46219, #18961 ) ;
#23531=CARTESIAN_POINT ( 'NONE',  ( 10.46933016578999975, -4.988498232033999891, 6.213103211926000569 ) ) ;
#23532=CARTESIAN_POINT ( 'NONE',  ( 9.669679685929221336, -5.627806328728547136, 6.860704028586689596 ) ) ;
#23540=CARTESIAN_POINT ( 'NONE',  ( 9.264851123445994929, -2.902720251407998830, -6.598525194663996452 ) ) ;
#23544=CARTESIAN_POINT ( 'NONE',  ( 9.705325322606999094, -5.130141620686999637, -6.219151643305999677 ) ) ;
#23566=ORIENTED_EDGE ( 'NONE', *, *, #3989, .T. ) ;
#23568=CARTESIAN_POINT ( 'NONE',  ( -2.147830119999999621, -1.300000000000000044, -9.662944685757000940 ) ) ;
#23578=CARTESIAN_POINT ( 'NONE',  ( 5.700000000000000178, -1.433333333332999837, 10.65401593558000037 ) ) ;
#23583=CARTESIAN_POINT ( 'NONE',  ( 9.510967806033882255, -2.744763247581829990, 6.279873002373912882 ) ) ;
#23584=ORIENTED_EDGE ( 'NONE', *, *, #33792, .T. ) ;
#23585=CARTESIAN_POINT ( 'NONE',  ( 5.500000000000000000, 0.000000000000000000, -1.449999999999970202 ) ) ;
#23598=CARTESIAN_POINT ( 'NONE',  ( 9.185618987146705550, -5.739014642741299355, 7.194290269894461964 ) ) ;
#23600=EDGE_CURVE ( 'NONE', #28855, #31101, #30809, .T. ) ;
#23601=CARTESIAN_POINT ( 'NONE',  ( 8.320870559624999885, -3.894643656844000379, 6.044452984962999764 ) ) ;
#23604=CARTESIAN_POINT ( 'NONE',  ( 10.96873203361999849, -6.471573332185999838, 5.204310805270999651 ) ) ;
#23607=EDGE_CURVE ( 'NONE', #43113, #50410, #22023, .T. ) ;
#23609=CARTESIAN_POINT ( 'NONE',  ( 11.13327849887000021, -2.674582802342999610, -4.980994678569999223 ) ) ;
#23625=ORIENTED_EDGE ( 'NONE', *, *, #58868, .F. ) ;
#23639=FACE_OUTER_BOUND ( 'NONE', #18425, .T. ) ;
#23655=CARTESIAN_POINT ( 'NONE',  ( 11.09999999999999964, -5.538898460221000519, 7.685179721164000277 ) ) ;
#23675=CARTESIAN_POINT ( 'NONE',  ( 10.94349328348999961, -3.081618981425999770, -8.919377696680001577 ) ) ;
#23679=DIRECTION ( 'NONE',  ( 0.000000000000000000, 0.8648648648648717963, 0.5020047465136827647 ) ) ;
#23684=EDGE_CURVE ( 'NONE', #16325, #37501, #16774, .T. ) ;
#23695=DIRECTION ( 'NONE',  ( 0.8843050093870579165, 0.1786785976936114684, 0.4313682986720279167 ) ) ;
#23697=ORIENTED_EDGE ( 'NONE', *, *, #59217, .F. ) ;
#23698=CARTESIAN_POINT ( 'NONE',  ( 9.362879440377000151, -3.677416446733000388, 9.250734868033999803 ) ) ;
#23704=EDGE_CURVE ( 'NONE', #65709, #25033, #63791, .T. ) ;
#23712=CARTESIAN_POINT ( 'NONE',  ( 10.83659005484000026, -5.133183563847000030, 8.848364935581999546 ) ) ;
#23717=CARTESIAN_POINT ( 'NONE',  ( 7.902908229829841424, -2.546181505345110008, 8.455233271057512212 ) ) ;
#23718=CARTESIAN_POINT ( 'NONE',  ( 10.46933016578999975, -4.988498232033999891, 6.213103211926000569 ) ) ;
#23721=ORIENTED_EDGE ( 'NONE', *, *, #38342, .F. ) ;
#23728=CARTESIAN_POINT ( 'NONE',  ( 10.06233042975999936, -5.062748727288000516, -8.618689820632001286 ) ) ;
#23730=CARTESIAN_POINT ( 'NONE',  ( 9.411640687503366465, -2.873222873813585654, -6.752018918873797126 ) ) ;
#23735=ORIENTED_EDGE ( 'NONE', *, *, #42168, .T. ) ;
#23739=CARTESIAN_POINT ( 'NONE',  ( 7.374102686541000651, -4.389298280625000714, 9.135255728583000945 ) ) ;
#23744=FACE_OUTER_BOUND ( 'NONE', #55294, .T. ) ;
#23757=VERTEX_POINT ( 'NONE', #27455 ) ;
#23758=B_SPLINE_CURVE_WITH_KNOTS ( 'NONE', 3,
 ( #33327, #65112, #53943, #16543, #32299, #44170, #11635, #65466, #43817, #17591, #59539, #22475 ),
 .UNSPECIFIED., .F., .F.,
 ( 4, 2, 2, 2, 2, 4 ),
 ( 0.000000000000000000, 0.2499999999999977240, 0.3749999999999977796, 0.4999999999999978906, 0.7499999999999988898, 1.000000000000000000 ),
 .UNSPECIFIED. ) ;
#23760=CARTESIAN_POINT ( 'NONE',  ( 5.500000000000000000, -1.449999999999999956, 0.000000000000000000 ) ) ;
#23771=CARTESIAN_POINT ( 'NONE',  ( 8.455992358812000731, -5.100000000000000533, 6.571291218949999902 ) ) ;
#23783=CARTESIAN_POINT ( 'NONE',  ( 7.956793146791999227, -4.524489047957000132, 9.047757046927999980 ) ) ;
#23788=( GEOMETRIC_REPRESENTATION_CONTEXT ( 3 ) GLOBAL_UNCERTAINTY_ASSIGNED_CONTEXT ( ( #33690 ) ) GLOBAL_UNIT_ASSIGNED_CONTEXT ( ( #59323, #53738, #42906 ) ) REPRESENTATION_CONTEXT ( 'NONE', 'WORKASPACE' ) );
#23803=CARTESIAN_POINT ( 'NONE',  ( 10.40685100253999984, -2.832432432432000269, -6.822293592207000934 ) ) ;
#23804=CARTESIAN_POINT ( 'NONE',  ( 7.432385141095590342, -2.300021307827942341, 7.868234740325537047 ) ) ;
#23805=CARTESIAN_POINT ( 'NONE',  ( 7.674792391072008613, -2.650477653308784376, 7.499986425013215552 ) ) ;
#23809=CARTESIAN_POINT ( 'NONE',  ( 10.78315545572531065, -5.333388898808085088, -6.342471701929282446 ) ) ;
#23812=CARTESIAN_POINT ( 'NONE',  ( 9.587263606520540549, -3.377808641630456243, 8.716806737538737693 ) ) ;
#23813=CARTESIAN_POINT ( 'NONE',  ( 10.53870444038000009, -5.103398787993000063, -6.705198626796000205 ) ) ;
#23839=AXIS2_PLACEMENT_3D ( 'NONE', #40395, #55799, #34823 ) ;
#23840=CARTESIAN_POINT ( 'NONE',  ( 10.90000000000000036, -8.091325576830000088, 7.077637346582999811 ) ) ;
#23846=CARTESIAN_POINT ( 'NONE',  ( 11.03855816545999957, -2.974093234901999949, 8.716125417860000724 ) ) ;
#23850=VERTEX_POINT ( 'NONE', #23585 ) ;
#23853=EDGE_CURVE ( 'NONE', #10703, #8532, #16818, .T. ) ;
#23857=CARTESIAN_POINT ( 'NONE',  ( 7.474999999999999645, -5.349999999999999645, 7.500000000000000000 ) ) ;
#23860=CARTESIAN_POINT ( 'NONE',  ( 10.32322128467999889, -4.600000125420001140, -4.621083553505000552 ) ) ;
#23862=CARTESIAN_POINT ( 'NONE',  ( 9.793328727373999953, -5.651611919872999934, -7.935921913274999184 ) ) ;
#23864=DIRECTION ( 'NONE',  ( 0.7071067811866525998, 0.000000000000000000, -0.7071067811864425456 ) ) ;
#23868=CARTESIAN_POINT ( 'NONE',  ( 10.73288376472999950, -2.790050529699000137, 4.894999077959000466 ) ) ;
#23873=CARTESIAN_POINT ( 'NONE',  ( 9.662553763536999796, -4.094830574823999925, 9.119950378356000087 ) ) ;
#23886=CARTESIAN_POINT ( 'NONE',  ( 11.04677151279999947, -2.764386413791999786, -5.039776830043000366 ) ) ;
#23888=CARTESIAN_POINT ( 'NONE',  ( 10.94076550314999885, -5.140765503144999471, -6.571291218949999902 ) ) ;
#23891=CARTESIAN_POINT ( 'NONE',  ( 9.010799540956998754, -4.699533657262000119, -6.366989705700999203 ) ) ;
#23893=ORIENTED_EDGE ( 'NONE', *, *, #14023, .T. ) ;
#23913=ORIENTED_EDGE ( 'NONE', *, *, #25663, .F. ) ;
#23917=DIRECTION ( 'NONE',  ( 0.000000000000000000, 0.000000000000000000, -1.000000000000000000 ) ) ;
#23919=ORIENTED_EDGE ( 'NONE', *, *, #67572, .F. ) ;
#23930=FACE_OUTER_BOUND ( 'NONE', #3950, .T. ) ;
#23937=FACE_OUTER_BOUND ( 'NONE', #3789, .T. ) ;
#23941=CARTESIAN_POINT ( 'NONE',  ( 10.22109127278999807, -2.983266195621000261, 8.764707262515999631 ) ) ;
#23950=CARTESIAN_POINT ( 'NONE',  ( 7.307500000000000107, -0.2999999999999999889, 3.149999999999999911 ) ) ;
#23963=CARTESIAN_POINT ( 'NONE',  ( 10.86324669354999983, -5.065490477172999384, 5.172188879882000379 ) ) ;
#23968=AXIS2_PLACEMENT_3D ( 'NONE', #47867, #63232, #68826 ) ;
#23976=CARTESIAN_POINT ( 'NONE',  ( 11.02452225494999993, -2.775477745048999800, -6.571291218949999902 ) ) ;
#23981=CYLINDRICAL_SURFACE ( 'NONE', #62017, 1.350000000000000089 ) ;
#23987=CARTESIAN_POINT ( 'NONE',  ( 9.959635380193999410, -5.406637819064000539, 7.700301345050000634 ) ) ;
#23990=CARTESIAN_POINT ( 'NONE',  ( 8.020980646792999380, -3.245532552444000185, 8.949627348471000943 ) ) ;
#24011=CARTESIAN_POINT ( 'NONE',  ( 10.44773515094007799, -5.286251723462822127, 7.027580072218823304 ) ) ;
#24012=CARTESIAN_POINT ( 'NONE',  ( 9.030800552329743880, -2.902287361240535102, 6.174410955705745607 ) ) ;
#24017=ORIENTED_EDGE ( 'NONE', *, *, #46397, .F. ) ;
#24018=CARTESIAN_POINT ( 'NONE',  ( 5.700000000000000178, -10.75000000000000000, 0.000000000000000000 ) ) ;
#24022=CARTESIAN_POINT ( 'NONE',  ( 11.17811058788999823, -2.762459764047000110, -6.187206491620000470 ) ) ;
#24024=PRODUCT_DEFINITION_FORMATION_WITH_SPECIFIED_SOURCE ( 'ANY', '', #56164, .NOT_KNOWN. ) ;
#24029=CARTESIAN_POINT ( 'NONE',  ( 10.16052890781999984, -2.899999999999999911, -6.152188490330000370 ) ) ;
#24035=AXIS2_PLACEMENT_3D ( 'NONE', #37850, #53242, #64748 ) ;
#24042=CARTESIAN_POINT ( 'NONE',  ( 8.400066940379998570, -2.800111029801999774, 9.079936276749000612 ) ) ;
#24051=EDGE_CURVE ( 'NONE', #3478, #53120, #18693, .T. ) ;
#24057=CARTESIAN_POINT ( 'NONE',  ( 10.89228096335999929, -3.998355205482000851, 9.261304730013998565 ) ) ;
#24061=CARTESIAN_POINT ( 'NONE',  ( 11.06877944038000017, -5.318813217120000658, -7.168443364726000411 ) ) ;
#24062=CARTESIAN_POINT ( 'NONE',  ( 7.913001903775949586, -2.440633479413790052, 8.271164008384964461 ) ) ;
#24064=CARTESIAN_POINT ( 'NONE',  ( 11.11845396862999991, -5.767021056207999763, 7.178419201465000121 ) ) ;
#24068=CARTESIAN_POINT ( 'NONE',  ( 10.38718558795000035, -4.935364245016000240, -4.601021236483000543 ) ) ;
#24073=CARTESIAN_POINT ( 'NONE',  ( 9.749152735436000583, -5.239375073306999475, -6.095351682555999240 ) ) ;
#24086=CARTESIAN_POINT ( 'NONE',  ( 8.315519353208999931, -5.485781663882000281, 8.532068390166999805 ) ) ;
#24088=ORIENTED_EDGE ( 'NONE', *, *, #38342, .T. ) ;
#24090=AXIS2_PLACEMENT_3D ( 'NONE', #38145, #21720, #54584 ) ;
#24092=CARTESIAN_POINT ( 'NONE',  ( 11.07691935321000010, -3.101896674955000321, -8.926549689995999515 ) ) ;
#24116=B_SPLINE_CURVE_WITH_KNOTS ( 'NONE', 3,
 ( #23886, #7115, #59906, #6413 ),
 .UNSPECIFIED., .F., .F.,
 ( 4, 4 ),
 ( 0.000000000000000000, 1.000000000000000000 ),
 .UNSPECIFIED. ) ;
#24126=CARTESIAN_POINT ( 'NONE',  ( 10.82056172568756303, -4.095931573296573980, 9.237050133684192588 ) ) ;
#24140=DIRECTION ( 'NONE',  ( -1.000000000000000000, 0.000000000000000000, 0.000000000000000000 ) ) ;
#24141=CARTESIAN_POINT ( 'NONE',  ( 5.499999999523999428, -0.5000000004757000349, 9.662944681389999957 ) ) ;
#24144=CARTESIAN_POINT ( 'NONE',  ( 7.629816940376999312, -4.763531818439999732, 5.668890958491999754 ) ) ;
#24148=LINE ( 'NONE', #45135, #57441 ) ;
#24150=CARTESIAN_POINT ( 'NONE',  ( 10.72510394928771227, -2.650147065043205519, 7.500007457243348163 ) ) ;
#24152=ORIENTED_EDGE ( 'NONE', *, *, #24998, .F. ) ;
#24158=CARTESIAN_POINT ( 'NONE',  ( 10.91732944037999964, -3.256268970540999952, -6.361552695759000287 ) ) ;
#24176=CARTESIAN_POINT ( 'NONE',  ( 10.81579453138999902, -5.374572909254000663, 6.698726302909000729 ) ) ;
#24178=DIRECTION ( 'NONE',  ( -0.7071067811865474617, 0.7071067811865474617, -3.640778010129241947E-09 ) ) ;
#24182=VECTOR ( 'NONE', #22586, 1000.000000000000000 ) ;
#24189=CARTESIAN_POINT ( 'NONE',  ( 9.442085454646999665, -4.742494605615999781, 8.809986937145000141 ) ) ;
#24203=CARTESIAN_POINT ( 'NONE',  ( 8.996132306828998892, -4.474581801608000120, -6.279517683005999551 ) ) ;
#24214=CARTESIAN_POINT ( 'NONE',  ( 9.910792656537999790, -3.869344906782000049, 5.882544796414999944 ) ) ;
#24221=CARTESIAN_POINT ( 'NONE',  ( 10.22452454188782767, -3.422561976923117477, -8.739574331469325941 ) ) ;
#24222=B_SPLINE_CURVE_WITH_KNOTS ( 'NONE', 3,
 ( #5080, #47744, #69059, #28451 ),
 .UNSPECIFIED., .F., .F.,
 ( 4, 4 ),
 ( 0.8745842163858279505, 1.000000000000000000 ),
 .UNSPECIFIED. ) ;
#24230=CARTESIAN_POINT ( 'NONE',  ( 10.88079290149999956, -2.937478892754000093, 5.081605332078000359 ) ) ;
#24234=CARTESIAN_POINT ( 'NONE',  ( 9.839913318575998602, -5.792391408692000532, -6.955579396894000510 ) ) ;
#24237=DIRECTION ( 'NONE',  ( -0.5298945030328949812, -4.148149686514954961E-09, 0.8480635681689911998 ) ) ;
#24252=CARTESIAN_POINT ( 'NONE',  ( 11.09999999999999964, -2.409623100499390436, -8.041736326814033831 ) ) ;
#24260=ORIENTED_EDGE ( 'NONE', *, *, #46002, .F. ) ;
#24261=B_SPLINE_CURVE_WITH_KNOTS ( 'NONE', 3,
 ( #40569, #51406, #61216, #34306, #39545, #66798, #8418, #35340, #29761, #67131, #45138, #24150 ),
 .UNSPECIFIED., .F., .F.,
 ( 4, 2, 2, 2, 2, 4 ),
 ( 0.1254754252289749794, 0.3127772825098947829, 0.5000791397908146418, 0.6873809970717346118, 0.7810319257121947079, 0.8746828543526545818 ),
 .UNSPECIFIED. ) ;
#24275=CARTESIAN_POINT ( 'NONE',  ( 9.408510579921751216, -2.486340047029418798, 8.356969995776358573 ) ) ;
#24279=CARTESIAN_POINT ( 'NONE',  ( 11.04391448624000027, -5.244599162544999693, -5.180563645961999697 ) ) ;
#24283=CARTESIAN_POINT ( 'NONE',  ( 9.290195424034999760, -2.377814350880000038, 7.540992175424999999 ) ) ;
#24299=CARTESIAN_POINT ( 'NONE',  ( 10.88830300260000072, -2.841398431944000436, -5.064211128354999758 ) ) ;
#24300=CARTESIAN_POINT ( 'NONE',  ( 9.235799540957000175, -4.950980172046000050, -5.959730545597000884 ) ) ;
#24301=CARTESIAN_POINT ( 'NONE',  ( 10.90437023801000116, -5.099522774867000230, 5.132565236215000049 ) ) ;
#24306=CARTESIAN_POINT ( 'NONE',  ( 10.90000000000000036, -0.2999999999999999889, 4.902439024389999567 ) ) ;
#24332=CARTESIAN_POINT ( 'NONE',  ( 10.79499900793999956, -3.503951165873000040, 6.168577387731000172 ) ) ;
#24333=ORIENTED_EDGE ( 'NONE', *, *, #56717, .T. ) ;
#24335=CARTESIAN_POINT ( 'NONE',  ( 8.753441940380000119, -2.876278577719999952, 6.568889245344999850 ) ) ;
#24351=DIRECTION ( 'NONE',  ( -0.7071067759742961645, 0.7071067863987962054, 5.966942998097971758E-08 ) ) ;
#24361=ORIENTED_EDGE ( 'NONE', *, *, #41059, .T. ) ;
#24367=CARTESIAN_POINT ( 'NONE',  ( 10.87695483801000051, -5.827068285690999438, -7.814745128155998977 ) ) ;
#24369=CARTESIAN_POINT ( 'NONE',  ( 9.044057935147195693, -4.875277019998068617, 8.528246069510029059 ) ) ;
#24387=CARTESIAN_POINT ( 'NONE',  ( 8.924956853209002006, -4.158911960977000000, 5.873536005760000123 ) ) ;
#24391=CARTESIAN_POINT ( 'NONE',  ( 7.777775979742000523, -3.623726805927396821, 6.172770137145197289 ) ) ;
#24393=B_SPLINE_CURVE_WITH_KNOTS ( 'NONE', 3,
 ( #45968, #61360, #67278, #45635, #13817, #40049, #66939, #2628, #45291, #13136 ),
 .UNSPECIFIED., .F., .F.,
 ( 4, 1, 1, 1, 1, 1, 1, 4 ),
 ( 0.000000000000000000, 0.1626725439853999866, 0.3253459288523000148, 0.4880193137191000119, 0.6506926985859999846, 0.8133660834529000683, 0.9760394683197000099, 1.000000000000000000 ),
 .UNSPECIFIED. ) ;
#24394=ORIENTED_EDGE ( 'NONE', *, *, #17034, .T. ) ;
#24403=CARTESIAN_POINT ( 'NONE',  ( 10.18909467608999897, -5.907859813488999912, 7.801539220053999912 ) ) ;
#24405=ORIENTED_EDGE ( 'NONE', *, *, #18898, .F. ) ;
#24410=CARTESIAN_POINT ( 'NONE',  ( 8.059688117792761730, -3.668144782959516181, 5.792266635259295526 ) ) ;
#24411=CARTESIAN_POINT ( 'NONE',  ( 10.59344961228999971, -5.297755890367000120, 8.474197994416998725 ) ) ;
#24415=CARTESIAN_POINT ( 'NONE',  ( 10.36994085745000049, -4.628299740363999604, -5.009923106717000252 ) ) ;
#24421=AXIS2_PLACEMENT_3D ( 'NONE', #3542, #51787, #19982 ) ;
#24422=ORIENTED_EDGE ( 'NONE', *, *, #64955, .T. ) ;
#24431=ORIENTED_EDGE ( 'NONE', *, *, #48777, .F. ) ;
#24433=CARTESIAN_POINT ( 'NONE',  ( 8.020980646792999380, -3.245532552444000185, 8.949627348471000943 ) ) ;
#24438=CARTESIAN_POINT ( 'NONE',  ( 11.12964314679000033, -3.869080819553999628, -9.017146989745999264 ) ) ;
#24447=ORIENTED_EDGE ( 'NONE', *, *, #3274, .T. ) ;
#24448=ORIENTED_EDGE ( 'NONE', *, *, #26995, .F. ) ;
#24459=CARTESIAN_POINT ( 'NONE',  ( 10.35465597998723553, -2.649863840850919416, -7.676734101936328436 ) ) ;
#24460=ORIENTED_EDGE ( 'NONE', *, *, #21522, .F. ) ;
#24477=CARTESIAN_POINT ( 'NONE',  ( 7.828418146791999099, -5.524126964933000927, 6.910359834012999691 ) ) ;
#24485=CARTESIAN_POINT ( 'NONE',  ( 8.767879976495999372, -3.394455611366999914, -6.293427637271999942 ) ) ;
#24487=CARTESIAN_POINT ( 'NONE',  ( 7.000000000000000000, -7.526486366024999874, 3.526486366024999874 ) ) ;
#24491=DIRECTION ( 'NONE',  ( 0.000000000000000000, -1.000000000000000000, 0.000000000000000000 ) ) ;
#24492=CARTESIAN_POINT ( 'NONE',  ( 7.667605646792000407, -5.638700495537999124, 8.266402903491000487 ) ) ;
#24495=DIRECTION ( 'NONE',  ( -1.000000000000000000, -2.893429392047000287E-14, 4.629487027275000025E-14 ) ) ;
#24497=CARTESIAN_POINT ( 'NONE',  ( 7.362367228725729795, -3.210354122145276712, 9.056218515521349488 ) ) ;
#24508=CARTESIAN_POINT ( 'NONE',  ( 11.06877944038000017, -5.318813217120000658, -7.168443364726000411 ) ) ;
#24509=CARTESIAN_POINT ( 'NONE',  ( 7.831326693633717362, -3.674448254819469017, 6.164223331809817630 ) ) ;
#24524=CARTESIAN_POINT ( 'NONE',  ( 9.701976361057999654, -3.399137684422000039, 6.026753338319999820 ) ) ;
#24528=CARTESIAN_POINT ( 'NONE',  ( 5.500000000000000000, 0.000000000000000000, 0.000000000000000000 ) ) ;
#24529=ORIENTED_EDGE ( 'NONE', *, *, #36782, .T. ) ;
#24530=CARTESIAN_POINT ( 'NONE',  ( 9.433148997456999751, -5.167567567567999731, 6.822293592207000934 ) ) ;
#24533=DIRECTION ( 'NONE',  ( -1.000000000000000000, 0.000000000000000000, 0.000000000000000000 ) ) ;
#24538=CARTESIAN_POINT ( 'NONE',  ( 10.02202195053999922, -3.298019507654999849, 5.700533868754000366 ) ) ;
#24539=ORIENTED_EDGE ( 'NONE', *, *, #11126, .F. ) ;
#24545=VECTOR ( 'NONE', #32922, 999.9999999999998863 ) ;
#24547=DIRECTION ( 'NONE',  ( -1.000000000000000000, 0.000000000000000000, 0.000000000000000000 ) ) ;
#24563=ORIENTED_EDGE ( 'NONE', *, *, #59648, .T. ) ;
#24566=CARTESIAN_POINT ( 'NONE',  ( 9.815199780373001559, -2.813634733202999616, 8.848854270764999086 ) ) ;
#24568=FACE_OUTER_BOUND ( 'NONE', #22875, .T. ) ;
#24570=CARTESIAN_POINT ( 'NONE',  ( 10.97865453029000093, -5.273142482194999481, 7.958032781726000593 ) ) ;
#24579=CARTESIAN_POINT ( 'NONE',  ( 11.04628392526000091, -2.754466683149000339, 5.119640974370000208 ) ) ;
#24580=DIRECTION ( 'NONE',  ( 0.000000000000000000, 0.000000000000000000, -1.000000000000000000 ) ) ;
#24582=CARTESIAN_POINT ( 'NONE',  ( 9.614739029020999084, -5.020908168068000776, -6.342951604057000203 ) ) ;
#24588=DIRECTION ( 'NONE',  ( 0.000000000000000000, 1.000000000000000000, 0.000000000000000000 ) ) ;
#24591=AXIS2_PLACEMENT_3D ( 'NONE', #45587, #18325, #40670 ) ;
#24619=LINE ( 'NONE', #57111, #43597 ) ;
#24620=EDGE_CURVE ( 'NONE', #4443, #44819, #51704, .T. ) ;
#24622=CARTESIAN_POINT ( 'NONE',  ( 9.404541696082119984, -2.531018779588075862, 8.431930544983709197 ) ) ;
#24627=DIRECTION ( 'NONE',  ( 0.000000000000000000, 1.000000000000000000, 0.000000000000000000 ) ) ;
#24637=CARTESIAN_POINT ( 'NONE',  ( 10.75304154458338424, -2.714670728013225176, 7.026954893539181235 ) ) ;
#24638=CARTESIAN_POINT ( 'NONE',  ( 7.474999999999999645, -5.349999999999999645, 7.500000000000000000 ) ) ;
#24642=VECTOR ( 'NONE', #59372, 1000.000000000000000 ) ;
#24646=EDGE_LOOP ( 'NONE', ( #53025, #28803, #54297, #6617 ) ) ;
#24649=CARTESIAN_POINT ( 'NONE',  ( 9.971744136172999262, -5.176458967229000230, -8.738385553646999426 ) ) ;
#24652=CARTESIAN_POINT ( 'NONE',  ( 11.04399668386999878, -5.244518219639999757, 5.182772251997000090 ) ) ;
#24656=EDGE_CURVE ( 'NONE', #8263, #37501, #37590, .T. ) ;
#24663=CARTESIAN_POINT ( 'NONE',  ( 5.500000000000000000, 0.000000000000000000, 0.000000000000000000 ) ) ;
#24675=B_SPLINE_CURVE_WITH_KNOTS ( 'NONE', 3,
 ( #34516, #55826, #50576, #2678 ),
 .UNSPECIFIED., .F., .F.,
 ( 4, 4 ),
 ( 0.000000000000000000, 1.000000000000000000 ),
 .UNSPECIFIED. ) ;
#24676=CARTESIAN_POINT ( 'NONE',  ( 9.701976361057999654, -3.399137684422000039, 6.026753338319999820 ) ) ;
#24679=CARTESIAN_POINT ( 'NONE',  ( 8.503174978518606153, -3.164505085781523785, 6.034520370687764590 ) ) ;
#24680=CARTESIAN_POINT ( 'NONE',  ( 7.726441940376999717, -2.630475685621000093, 6.995953627589999613 ) ) ;
#24683=CARTESIAN_POINT ( 'NONE',  ( 7.724131401290000198, -9.034333619270000781, 5.486219533306999629 ) ) ;
#24689=VERTEX_POINT ( 'NONE', #22468 ) ;
#24693=CARTESIAN_POINT ( 'NONE',  ( 10.40879003340999986, -3.093879171920000282, -6.480773124728999690 ) ) ;
#24704=EDGE_CURVE ( 'NONE', #67791, #43366, #61736, .T. ) ;
#24712=CARTESIAN_POINT ( 'NONE',  ( 10.24845588172999911, -4.234132110154000372, -5.660862927546999934 ) ) ;
#24720=CARTESIAN_POINT ( 'NONE',  ( 8.143316940379001778, -5.061720701958000390, 5.824087910811999613 ) ) ;
#24732=CARTESIAN_POINT ( 'NONE',  ( 9.143918146793000190, -5.791549888895000109, 7.752110689268000954 ) ) ;
#24734=CARTESIAN_POINT ( 'NONE',  ( 7.827987191645501497, -4.479149983889610276, 6.206347837179650995 ) ) ;
#24748=CARTESIAN_POINT ( 'NONE',  ( 11.09999999999999964, -5.299999998684000069, -5.146420581040999309 ) ) ;
#24749=ORIENTED_EDGE ( 'NONE', *, *, #16130, .T. ) ;
#24752=CARTESIAN_POINT ( 'NONE',  ( 8.218889947459839362, -5.685407169154115259, 7.929140997506675781 ) ) ;
#24756=CARTESIAN_POINT ( 'NONE',  ( 10.49744223918999886, -4.907449962201999583, -5.047071811637001026 ) ) ;
#24758=ORIENTED_EDGE ( 'NONE', *, *, #48697, .T. ) ;
#24761=CARTESIAN_POINT ( 'NONE',  ( 9.485142521132999605, -3.025808284870999731, -9.100010361367001366 ) ) ;
#24762=CARTESIAN_POINT ( 'NONE',  ( 10.90054769436000015, -2.705757430156999988, -4.902711565806999516 ) ) ;
#24772=CARTESIAN_POINT ( 'NONE',  ( 9.497293146791999874, -3.734278838175999482, 8.942129638874000364 ) ) ;
#24777=CARTESIAN_POINT ( 'NONE',  ( 11.20536814679000059, -2.688541832249000230, -8.273932507170000505 ) ) ;
#24784=EDGE_CURVE ( 'NONE', #49271, #35912, #53250, .T. ) ;
#24787=VERTEX_POINT ( 'NONE', #54641 ) ;
#24789=CARTESIAN_POINT ( 'NONE',  ( 10.91949602487000170, -5.247971730353000019, 4.977236201457000853 ) ) ;
#24790=AXIS2_PLACEMENT_3D ( 'NONE', #23076, #17495, #7342 ) ;
#24791=CARTESIAN_POINT ( 'NONE',  ( 8.571413182548997867, -4.600000000000999734, 5.927302706106000407 ) ) ;
#24796=VECTOR ( 'NONE', #28152, 1000.000000000000000 ) ;
#24817=CARTESIAN_POINT ( 'NONE',  ( 10.70424414268935287, -5.750615589152155316, 7.605733149126583825 ) ) ;
#24818=CARTESIAN_POINT ( 'NONE',  ( 9.266941940380000631, -3.049610585291000042, 6.392533570808999421 ) ) ;
#24833=CARTESIAN_POINT ( 'NONE',  ( 7.410855646792000151, -2.302293129340000188, 6.875167727519000849 ) ) ;
#24845=CARTESIAN_POINT ( 'NONE',  ( 10.67745206237895417, -5.060860780720525476, 5.064629868885281105 ) ) ;
#24850=DIRECTION ( 'NONE',  ( -1.000000000000000000, 0.000000000000000000, 0.000000000000000000 ) ) ;
#24851=CARTESIAN_POINT ( 'NONE',  ( 8.654006363155202664, -3.802134689411699853, 5.879617511049518797 ) ) ;
#24858=ORIENTED_EDGE ( 'NONE', *, *, #35668, .F. ) ;
#24859=CARTESIAN_POINT ( 'NONE',  ( 8.766851002546001581, -2.832432432432000269, 6.822293592207000934 ) ) ;
#24865=CARTESIAN_POINT ( 'NONE',  ( 9.736871746126999128, -2.742172332680000046, 6.839224809731999422 ) ) ;
#24867=CARTESIAN_POINT ( 'NONE',  ( 10.16989351219999982, -2.594225604561000154, -6.291264536816999708 ) ) ;
#24870=PLANE ( 'NONE',  #64590 ) ;
#24873=CARTESIAN_POINT ( 'NONE',  ( 11.07071157029000119, -5.425561924405000624, -5.078387321380000152 ) ) ;
#24879=CARTESIAN_POINT ( 'NONE',  ( 10.13340376756999994, -5.653635692335999607, 6.501829690795999817 ) ) ;
#24892=CARTESIAN_POINT ( 'NONE',  ( 7.000000000000000000, -7.526486366024999874, -3.526486366024999874 ) ) ;
#24909=CARTESIAN_POINT ( 'NONE',  ( 9.384624721950221016, -2.899999999999999911, 6.445686799063069294 ) ) ;
#24922=CARTESIAN_POINT ( 'NONE',  ( 9.438732219486000830, -2.462132291381999849, -7.373611177161000008 ) ) ;
#24923=CARTESIAN_POINT ( 'NONE',  ( 10.26947109217999810, -5.100000000000000533, -6.152188490330000370 ) ) ;
#24930=LINE ( 'NONE', #36108, #39612 ) ;
#24932=ORIENTED_EDGE ( 'NONE', *, *, #13546, .T. ) ;
#24937=CYLINDRICAL_SURFACE ( 'NONE', #24591, 1.350000000000000089 ) ;
#24942=CARTESIAN_POINT ( 'NONE',  ( 11.09999999999999964, -2.649999999999999911, -7.500000000000000000 ) ) ;
#24963=CARTESIAN_POINT ( 'NONE',  ( 9.961660622463165637, -5.351629337096486694, 7.263483964539670268 ) ) ;
#24968=CARTESIAN_POINT ( 'NONE',  ( 10.06493315628555862, -5.349942305088194239, -7.500003965376651038 ) ) ;
#24969=CARTESIAN_POINT ( 'NONE',  ( 10.60519595724999853, -5.343977295764999802, -7.731524081231999190 ) ) ;
#24981=CARTESIAN_POINT ( 'NONE',  ( 8.248511556582998949, -4.520635131647999572, -6.809650021909999573 ) ) ;
#24985=CARTESIAN_POINT ( 'NONE',  ( 10.49202233201000034, -3.034490706411000271, -4.914423043680000269 ) ) ;
#24986=CARTESIAN_POINT ( 'NONE',  ( 9.443723707566000769, -5.531435376468999188, -8.256621485025000595 ) ) ;
#24993=CARTESIAN_POINT ( 'NONE',  ( 8.164397154371004106, -4.665396042252996978, 6.167056685642003266 ) ) ;
#24997=ORIENTED_EDGE ( 'NONE', *, *, #33105, .T. ) ;
#24998=EDGE_CURVE ( 'NONE', #11391, #21776, #68208, .T. ) ;
#25015=CARTESIAN_POINT ( 'NONE',  ( 10.81579453138999902, -5.374572909254000663, 6.698726302909000729 ) ) ;
#25017=CARTESIAN_POINT ( 'NONE',  ( 7.653716352205310436, -2.685215128838110310, 7.854066585618749485 ) ) ;
#25026=CARTESIAN_POINT ( 'NONE',  ( 8.161249603540388975, -2.987768769759142629, 6.407057936808166154 ) ) ;
#25028=CARTESIAN_POINT ( 'NONE',  ( 9.409308287954999628, -2.634700736117999931, 8.920302460802998823 ) ) ;
#25031=CARTESIAN_POINT ( 'NONE',  ( 10.84088306584999906, -2.636277440143000472, -7.512643837511999934 ) ) ;
#25032=CARTESIAN_POINT ( 'NONE',  ( 9.702862956261629535, -2.713451880143079809, 7.026479373627134706 ) ) ;
#25033=VERTEX_POINT ( 'NONE', #57998 ) ;
#25037=CARTESIAN_POINT ( 'NONE',  ( 10.47530200610951034, -5.350262918594152595, 7.499984559551212904 ) ) ;
#25043=CARTESIAN_POINT ( 'NONE',  ( 7.729221580034996819, -5.085115902530001897, 6.553339126910996626 ) ) ;
#25049=CARTESIAN_POINT ( 'NONE',  ( 10.23643195768000069, -5.517145045299000294, -6.754127937316000363 ) ) ;
#25058=CARTESIAN_POINT ( 'NONE',  ( 7.694004440376999376, -5.850279024084999335, 6.784181137144999596 ) ) ;
#25062=LINE ( 'NONE', #50609, #19088 ) ;
#25069=CARTESIAN_POINT ( 'NONE',  ( 7.807370559623000084, -3.650411072918999800, 6.083135626079000602 ) ) ;
#25074=AXIS2_PLACEMENT_3D ( 'NONE', #55032, #49785, #2241 ) ;
#25087=DIRECTION ( 'NONE',  ( 0.4384236320214023874, 0.000000000000000000, 0.8987684456439055669 ) ) ;
#25091=DIRECTION ( 'NONE',  ( 1.000000000000000000, 0.000000000000000000, 0.000000000000000000 ) ) ;
#25093=CARTESIAN_POINT ( 'NONE',  ( 8.125618316923414852, -5.037132069328078998, 6.102874426331527324 ) ) ;
#25096=CARTESIAN_POINT ( 'NONE',  ( 10.31494349883999995, -4.644418916688000110, -4.564229129027999932 ) ) ;
#25101=CARTESIAN_POINT ( 'NONE',  ( 9.622313405920001728, -4.009302068291999532, -9.043024413115999138 ) ) ;
#25102=DIRECTION ( 'NONE',  ( -1.000000000000000000, 0.000000000000000000, -5.786858784063000233E-14 ) ) ;
#25109=ORIENTED_EDGE ( 'NONE', *, *, #30018, .T. ) ;
#25111=CARTESIAN_POINT ( 'NONE',  ( 8.995183059623999000, -2.707994276285999646, 5.994456121676999594 ) ) ;
#25113=VERTEX_POINT ( 'NONE', #44346 ) ;
#25117=( GEOMETRIC_REPRESENTATION_CONTEXT ( 3 ) GLOBAL_UNCERTAINTY_ASSIGNED_CONTEXT ( ( #10116 ) ) GLOBAL_UNIT_ASSIGNED_CONTEXT ( ( #20568, #34949, #57276 ) ) REPRESENTATION_CONTEXT ( 'NONE', 'WORKASPACE' ) );
#25118=CARTESIAN_POINT ( 'NONE',  ( 11.11478185320999934, -2.548220588762000194, -8.356740464335999263 ) ) ;
#25151=CARTESIAN_POINT ( 'NONE',  ( 9.175271089438615135, -2.907098125219630624, 8.295045686540735375 ) ) ;
#25170=FACE_OUTER_BOUND ( 'NONE', #6089, .T. ) ;
#25171=CARTESIAN_POINT ( 'NONE',  ( 8.758793146794999984, -3.977267280662000193, 9.308921106447000327 ) ) ;
#25176=CARTESIAN_POINT ( 'NONE',  ( 10.00190805961999807, -2.729654112791000120, -8.843024969850999284 ) ) ;
#25177=CARTESIAN_POINT ( 'NONE',  ( 7.481712774526203091, -2.396946871456744788, 6.823884033406665495 ) ) ;
#25191=CARTESIAN_POINT ( 'NONE',  ( 9.475279990687656806, -5.350441389720279162, 7.499985493516659218 ) ) ;
#25195=VERTEX_POINT ( 'NONE', #48080 ) ;
#25204=CARTESIAN_POINT ( 'NONE',  ( 10.31457635473999979, -5.362146312020000138, 6.677778992223999843 ) ) ;
#25209=ORIENTED_EDGE ( 'NONE', *, *, #53095, .F. ) ;
#25211=CARTESIAN_POINT ( 'NONE',  ( 6.799999045260999964, -9.295457794069999835, 5.399713664196000629 ) ) ;
#25229=CARTESIAN_POINT ( 'NONE',  ( 8.940795537697432849, -5.100000000000000533, 6.662590550605505868 ) ) ;
#25234=DIRECTION ( 'NONE',  ( -1.000000000000000000, 0.000000000000000000, 0.000000000000000000 ) ) ;
#25244=DIRECTION ( 'NONE',  ( 0.000000000000000000, 1.000000000000000000, 0.000000000000000000 ) ) ;
#25253=EDGE_CURVE ( 'NONE', #27541, #25841, #9982, .T. ) ;
#25260=CARTESIAN_POINT ( 'NONE',  ( 8.267078902232004367, -3.206627312864001489, -6.583550664415995790 ) ) ;
#25261=AXIS2_PLACEMENT_3D ( 'NONE', #64231, #59006, #52722 ) ;
#25265=CARTESIAN_POINT ( 'NONE',  ( 10.38053305961999939, -5.283785200568999585, -8.830188095997000275 ) ) ;
#25266=CARTESIAN_POINT ( 'NONE',  ( 8.945154276125833803, -5.350566776863196594, 7.852883605855081051 ) ) ;
#25269=CARTESIAN_POINT ( 'NONE',  ( 9.174642513462206495, -2.649442673322992103, 7.499981897072125925 ) ) ;
#25278=CARTESIAN_POINT ( 'NONE',  ( 8.476519155276850626, -5.080278632455760501, 8.330433920098281320 ) ) ;
#25281=EDGE_CURVE ( 'NONE', #2324, #2854, #24222, .T. ) ;
#25300=CARTESIAN_POINT ( 'NONE',  ( 10.52657390975000062, -8.217615421285000110, -6.595888977210999649 ) ) ;
#25308=CARTESIAN_POINT ( 'NONE',  ( 9.792315001194999979, -4.284154785471999460, -9.000488933596999530 ) ) ;
#25315=CARTESIAN_POINT ( 'NONE',  ( 7.102406491832000235, -0.2966009291953999871, 3.049954386258999950 ) ) ;
#25316=CARTESIAN_POINT ( 'NONE',  ( 8.241912900173000267, -4.599999999999999645, 6.117539782833000928 ) ) ;
#25322=CARTESIAN_POINT ( 'NONE',  ( 8.914833952003988315, -4.559940160807997245, -6.172232737057998797 ) ) ;
#25324=CARTESIAN_POINT ( 'NONE',  ( 11.05581126733999930, -2.753616725312000302, 5.054244401329000880 ) ) ;
#25325=CARTESIAN_POINT ( 'NONE',  ( 10.36275829612999821, -3.274066978825000085, -4.865563198160999470 ) ) ;
#25343=PLANE ( 'NONE',  #36823 ) ;
#25346=CARTESIAN_POINT ( 'NONE',  ( 8.455992358785000107, -3.399999999999999911, 6.571291218964999459 ) ) ;
#25354=CARTESIAN_POINT ( 'NONE',  ( 10.57223537388000167, -4.020426196685999543, 8.920680607665000039 ) ) ;
#25357=FACE_OUTER_BOUND ( 'NONE', #39371, .T. ) ;
#25365=LINE ( 'NONE', #26407, #16369 ) ;
#25368=CARTESIAN_POINT ( 'NONE',  ( 10.21608469020999976, -5.961703525007000515, 7.319668113368000384 ) ) ;
#25372=CARTESIAN_POINT ( 'NONE',  ( 10.05525937050999907, -5.223866772223000332, -6.898311956607000361 ) ) ;
#25384=CARTESIAN_POINT ( 'NONE',  ( 7.613711861438999584, -4.858906194260998568, 6.437673909214002954 ) ) ;
#25390=CARTESIAN_POINT ( 'NONE',  ( 9.961463664312999455, -2.787129471086000176, -8.677705025472000955 ) ) ;
#25392=CARTESIAN_POINT ( 'NONE',  ( 9.040000584825472529, -4.926967860734864146, 8.481257932625776874 ) ) ;
#25398=( BOUNDED_SURFACE ( )  B_SPLINE_SURFACE ( 3, 3, ( 
 ( #1947, #12086, #59976, #6835, #49484, #1595, #22910, #65560, #17684 ),
 ( #56109, #67965, #45965, #66595, #67275, #8562, #51547, #8221, #34798 ),
 ( #19741, #46314, #9233, #61696, #19391, #14500, #3643, #20080, #29568 ),
 ( #25322, #67614, #35145, #14158, #56457, #61358, #30573, #30243, #24981 ) ),
 .UNSPECIFIED., .F., .F., .T. ) 
 B_SPLINE_SURFACE_WITH_KNOTS ( ( 4, 4 ),
 ( 4, 1, 1, 1, 1, 1, 4 ),
 ( 0.000000000000000000, 1.000000000000000000 ),
 ( -0.006083171280208000097, 0.000000000000000000, 0.04308213411242000496, 0.08189950809580999469, 0.1190113006902999981, 0.1566624088843000251, 0.1888062695230000032 ),
 .UNSPECIFIED. ) 
 GEOMETRIC_REPRESENTATION_ITEM ( )  RATIONAL_B_SPLINE_SURFACE ( (
 ( 1.221012668528999923, 1.221012668528999923, 1.221012668528999923, 1.221012668528999923, 1.221012668528999923, 1.221012668528999923, 1.221012668528999923, 1.221012668528999923, 1.221012668528999923),
 ( 0.9263291104904000095, 0.9263291104904000095, 0.9263291104904000095, 0.9263291104904000095, 0.9263291104904000095, 0.9263291104904000095, 0.9263291104904000095, 0.9263291104904000095, 0.9263291104904000095),
 ( 0.9263291104904000095, 0.9263291104904000095, 0.9263291104904000095, 0.9263291104904000095, 0.9263291104904000095, 0.9263291104904000095, 0.9263291104904000095, 0.9263291104904000095, 0.9263291104904000095),
 ( 1.221012668528999923, 1.221012668528999923, 1.221012668528999923, 1.221012668528999923, 1.221012668528999923, 1.221012668528999923, 1.221012668528999923, 1.221012668528999923, 1.221012668528999923) ) ) 
 REPRESENTATION_ITEM ( '' )  SURFACE ( )  );
#25414=ORIENTED_EDGE ( 'NONE', *, *, #46050, .F. ) ;
#25415=CARTESIAN_POINT ( 'NONE',  ( 8.256683059623998844, -2.876278577719999952, 6.568889245344999850 ) ) ;
#25418=EDGE_LOOP ( 'NONE', ( #42747, #1296, #15148, #34170, #67108, #32074, #49654, #5712, #65219, #48855, #49858, #61040, #24460, #67659 ) ) ;
#25427=FACE_OUTER_BOUND ( 'NONE', #29618, .T. ) ;
#25429=CARTESIAN_POINT ( 'NONE',  ( 7.955253088807634043, -4.981915319337616666, 6.461888573305477834 ) ) ;
#25434=CARTESIAN_POINT ( 'NONE',  ( 8.128235176271338958, -5.082034189686122971, 6.137861258929247832 ) ) ;
#25437=CARTESIAN_POINT ( 'NONE',  ( 9.150552008289244199, -4.457243628887224141, 8.907160125525155792 ) ) ;
#25443=CARTESIAN_POINT ( 'NONE',  ( 8.610875063856999745, -4.757997781751000410, 5.934102420827000124 ) ) ;
#25458=CARTESIAN_POINT ( 'NONE',  ( 10.73615685320999980, -3.078046833211999900, -6.088743704655001032 ) ) ;
#25463=VECTOR ( 'NONE', #17235, 1000.000000000000000 ) ;
#25471=FILL_AREA_STYLE ('',( #4476 ) ) ;
#25475=CARTESIAN_POINT ( 'NONE',  ( 10.90000000000000036, -1.300000000000000044, -9.662944685757000940 ) ) ;
#25497=CARTESIAN_POINT ( 'NONE',  ( 9.210689323432788456, -2.672069879332360731, 7.743984006150673949 ) ) ;
#25520=CARTESIAN_POINT ( 'NONE',  ( 7.282480646792000023, -3.448181789123000218, 9.222458996124998976 ) ) ;
#25522=CARTESIAN_POINT ( 'NONE',  ( 9.709999999999999076, -4.496968146123999865, -8.755198255949000696 ) ) ;
#25525=CARTESIAN_POINT ( 'NONE',  ( 7.595193963087873534, -4.443510954364005450, 5.817927645250587254 ) ) ;
#25546=CARTESIAN_POINT ( 'NONE',  ( 10.58422653167975902, -2.899999999999999911, 6.304440313954331465 ) ) ;
#25548=CARTESIAN_POINT ( 'NONE',  ( 10.26195635058000022, -4.650927364049000090, 4.591198219796000402 ) ) ;
#25553=CARTESIAN_POINT ( 'NONE',  ( 9.792562654643999664, -3.463427761954999795, 6.184385360914999907 ) ) ;
#25566=CARTESIAN_POINT ( 'NONE',  ( 9.799258316471000541, -4.057329063942999525, 9.430691159271001212 ) ) ;
#25568=VECTOR ( 'NONE', #45721, 1000.000000000000000 ) ;
#25570=EDGE_CURVE ( 'NONE', #20484, #27255, #21605, .T. ) ;
#25572=EDGE_CURVE ( 'NONE', #45838, #21138, #14435, .T. ) ;
#25576=CARTESIAN_POINT ( 'NONE',  ( 10.46933016578999975, -4.988498232033999891, 6.213103211926000569 ) ) ;
#25577=FACE_OUTER_BOUND ( 'NONE', #15022, .T. ) ;
#25593=B_SPLINE_CURVE_WITH_KNOTS ( 'NONE', 3,
 ( #37460, #33262, #48987, #57 ),
 .UNSPECIFIED., .F., .F.,
 ( 4, 4 ),
 ( 0.000000000000000000, 0.1252897476283257872 ),
 .UNSPECIFIED. ) ;
#25596=CARTESIAN_POINT ( 'NONE',  ( 9.758146639703001668, -2.901368778958000050, 6.555068849476000103 ) ) ;
#25609=CARTESIAN_POINT ( 'NONE',  ( 11.13352130964999809, -2.664740441716999975, 5.115464099832999878 ) ) ;
#25613=CARTESIAN_POINT ( 'NONE',  ( 10.34267055962000015, -5.750479631840000216, -8.094412205797999249 ) ) ;
#25624=CARTESIAN_POINT ( 'NONE',  ( 8.379867906070000316, -2.923743482135000349, 6.439439799216000182 ) ) ;
#25632=LINE ( 'NONE', #24942, #212 ) ;
#25638=AXIS2_PLACEMENT_3D ( 'NONE', #8084, #19251, #28376 ) ;
#25655=CARTESIAN_POINT ( 'NONE',  ( 10.85290698989999925, -3.170384785323999921, -8.782188229854000383 ) ) ;
#25662=DIRECTION ( 'NONE',  ( 1.000000000000000000, 0.000000000000000000, 0.000000000000000000 ) ) ;
#25663=EDGE_CURVE ( 'NONE', #27164, #10703, #3047, .T. ) ;
#25670=CARTESIAN_POINT ( 'NONE',  ( 11.09056211382000079, -2.710928475574999830, 5.109860994294000314 ) ) ;
#25671=CARTESIAN_POINT ( 'NONE',  ( 10.32823945355000106, -3.233612306621999721, -4.570995416535999389 ) ) ;
#25683=ORIENTED_EDGE ( 'NONE', *, *, #35059, .T. ) ;
#25688=DIRECTION ( 'NONE',  ( 0.9993918455886502406, 0.000000000000000000, -0.03487031647277825247 ) ) ;
#25689=CARTESIAN_POINT ( 'NONE',  ( 11.09999999999999964, -1.406666666667000021, 10.45580168561000001 ) ) ;
#25691=CARTESIAN_POINT ( 'NONE',  ( 9.520528907821001141, -2.899999999999999911, 6.152188490330000370 ) ) ;
#25699=CARTESIAN_POINT ( 'NONE',  ( 10.46085355684000007, -5.403406918566000527, 7.721809917403000156 ) ) ;
#25702=CARTESIAN_POINT ( 'NONE',  ( 8.700644353210000403, -5.212258818969000451, 6.157189191035000064 ) ) ;
#25711=ORIENTED_EDGE ( 'NONE', *, *, #65506, .F. ) ;
#25712=CARTESIAN_POINT ( 'NONE',  ( 10.71756905878999966, -3.040221764047000175, 8.808455607108001573 ) ) ;
#25716=CARTESIAN_POINT ( 'NONE',  ( 10.73506343560000076, -5.202499304193000107, -8.441414596927000247 ) ) ;
#25727=CARTESIAN_POINT ( 'NONE',  ( 9.792562654643999664, -3.463427761954999795, 6.184385360914999907 ) ) ;
#25729=ADVANCED_FACE ( 'NONE', ( #43056 ), #5304, .T. ) ;
#25732=EDGE_LOOP ( 'NONE', ( #11805, #65177, #40388 ) ) ;
#25735=B_SPLINE_CURVE_WITH_KNOTS ( 'NONE', 3,
 ( #4833, #63567, #25826, #15680, #69159, #57633, #26870, #52739, #14989, #26175 ),
 .UNSPECIFIED., .F., .F.,
 ( 4, 1, 1, 1, 1, 1, 1, 4 ),
 ( 0.000000000000000000, 0.1608394309853999893, 0.3216792337757999887, 0.4825190365663000192, 0.6433588393567000185, 0.8041986421472000490, 0.9650384449376000484, 1.000000000000000000 ),
 .UNSPECIFIED. ) ;
#25736=VECTOR ( 'NONE', #62226, 1000.000000000000000 ) ;
#25750=CARTESIAN_POINT ( 'NONE',  ( 7.330275273710999961, -4.426925773067000414, 9.293310812901001583 ) ) ;
#25762=CARTESIAN_POINT ( 'NONE',  ( 8.090519353209000286, -5.342173944271999986, 8.432314172168000610 ) ) ;
#25764=CARTESIAN_POINT ( 'NONE',  ( 9.716851002543000604, -2.832432432432000269, 6.822293592207000934 ) ) ;
#25775=CARTESIAN_POINT ( 'NONE',  ( 7.953520338486511854, -5.020965158977404030, 6.510618665280695438 ) ) ;
#25777=VERTEX_POINT ( 'NONE', #37464 ) ;
#25780=CARTESIAN_POINT ( 'NONE',  ( 8.288236139519369772, -4.758661544608824734, 9.065029047955855290 ) ) ;
#25790=EDGE_CURVE ( 'NONE', #43366, #2324, #57515, .T. ) ;
#25795=CARTESIAN_POINT ( 'NONE',  ( 8.633274456858801571, -5.179562484155885826, 6.206446419389337166 ) ) ;
#25798=VERTEX_POINT ( 'NONE', #68580 ) ;
#25800=CARTESIAN_POINT ( 'NONE',  ( 7.454683059621999952, -2.138201851198999748, 6.814774777484000623 ) ) ;
#25802=ORIENTED_EDGE ( 'NONE', *, *, #6042, .T. ) ;
#25815=SURFACE_STYLE_USAGE ( .BOTH. , #57624 ) ;
#25820=CARTESIAN_POINT ( 'NONE',  ( 10.80160188108999897, -2.805072368922999715, -8.157282064671999677 ) ) ;
#25826=CARTESIAN_POINT ( 'NONE',  ( 10.33542413490000023, -4.762105522783999234, -4.627036157596999821 ) ) ;
#25841=VERTEX_POINT ( 'NONE', #33269 ) ;
#25854=ORIENTED_EDGE ( 'NONE', *, *, #21910, .T. ) ;
#25859=CARTESIAN_POINT ( 'NONE',  ( 7.320269353207000229, -2.466384407480000096, 6.935560677555000275 ) ) ;
#25862=CARTESIAN_POINT ( 'NONE',  ( 10.14206215041809678, -3.293869621293440630, 8.705460445251572921 ) ) ;
#25863=CARTESIAN_POINT ( 'NONE',  ( 10.34267055962000015, -5.750479631840000216, -8.094412205797999249 ) ) ;
#25864=CARTESIAN_POINT ( 'NONE',  ( 7.477637590078199281, -2.363906917100113692, 6.907238326532012529 ) ) ;
#25868=DIRECTION ( 'NONE',  ( -0.03487031647297116066, -1.485878521854048177E-07, -0.9993918455886323660 ) ) ;
#25874=EDGE_CURVE ( 'NONE', #6365, #20862, #61608, .T. ) ;
#25881=B_SPLINE_CURVE_WITH_KNOTS ( 'NONE', 3,
 ( #31185, #47254, #20679, #42010 ),
 .UNSPECIFIED., .F., .F.,
 ( 4, 4 ),
 ( 0.000000000000000000, 1.000000000000000000 ),
 .UNSPECIFIED. ) ;
#25892=B_SPLINE_CURVE_WITH_KNOTS ( 'NONE', 3,
 ( #4975, #52182, #30188, #35767 ),
 .UNSPECIFIED., .F., .F.,
 ( 4, 4 ),
 ( 0.000000000000000000, 1.000000000000000000 ),
 .UNSPECIFIED. ) ;
#25896=CARTESIAN_POINT ( 'NONE',  ( 10.18909467608999897, -5.907859813488999912, 7.801539220053999912 ) ) ;
#25900=CARTESIAN_POINT ( 'NONE',  ( 10.67500447327561908, -2.650284540010996004, 7.500001951671615430 ) ) ;
#25908=CARTESIAN_POINT ( 'NONE',  ( 9.260912867475999732, -4.901383038209000453, 9.090314591495999963 ) ) ;
#25915=CARTESIAN_POINT ( 'NONE',  ( 10.49785673611999925, -3.776281940467000275, 5.717636230565000588 ) ) ;
#25921=PLANE ( 'NONE',  #40450 ) ;
#25933=VECTOR ( 'NONE', #56370, 1000.000000000000114 ) ;
#25937=CARTESIAN_POINT ( 'NONE',  ( 9.571967469951999874, -4.084684048989999816, 8.946621592834999248 ) ) ;
#25946=CARTESIAN_POINT ( 'NONE',  ( 9.814967517147769271, -2.649990781018497721, -7.499998108648967765 ) ) ;
#25953=FACE_OUTER_BOUND ( 'NONE', #45755, .T. ) ;
#25954=CARTESIAN_POINT ( 'NONE',  ( 11.07691935321000010, -3.101896674955000321, -8.926549689995999515 ) ) ;
#25957=EDGE_CURVE ( 'NONE', #24787, #56474, #49981, .T. ) ;
#25958=CARTESIAN_POINT ( 'NONE',  ( 10.90454231406000041, -5.099691312770999296, -5.130383474399000221 ) ) ;
#25961=CARTESIAN_POINT ( 'NONE',  ( 9.202182965154866778, -2.714244241233930044, 7.027734220012900934 ) ) ;
#25971=ORIENTED_EDGE ( 'NONE', *, *, #67630, .F. ) ;
#25982=ORIENTED_EDGE ( 'NONE', *, *, #35614, .F. ) ;
#25984=AXIS2_PLACEMENT_3D ( 'NONE', #8085, #66808, #3180 ) ;
#25996=CARTESIAN_POINT ( 'NONE',  ( 7.976886985233528904, -5.078974948772455811, 8.328785302375353083 ) ) ;
#26000=CARTESIAN_POINT ( 'NONE',  ( 9.766127544684000128, -4.735430008785999512, -8.791396910319001279 ) ) ;
#26004=ADVANCED_FACE ( 'NONE', ( #43331 ), #17087, .F. ) ;
#26006=DIRECTION ( 'NONE',  ( -0.7660444431221081762, 4.730466324156050957E-08, -0.6427876096828072372 ) ) ;
#26014=CARTESIAN_POINT ( 'NONE',  ( 7.540373275913000661, -2.929987504175003199, 6.557984262489997995 ) ) ;
#26017=CARTESIAN_POINT ( 'NONE',  ( 10.33329075818000042, -3.361960872129000411, -4.712792984770999283 ) ) ;
#26020=CARTESIAN_POINT ( 'NONE',  ( 10.68403590588000007, -5.436611040123999317, 8.578433628717998971 ) ) ;
#26024=CARTESIAN_POINT ( 'NONE',  ( 7.591287949680001645, -4.587787988499997915, 6.499994349715005448 ) ) ;
#26052=CARTESIAN_POINT ( 'NONE',  ( 7.601545473805123798, -3.171576391775400516, 8.578950414869172647 ) ) ;
#26053=CARTESIAN_POINT ( 'NONE',  ( 8.855418146794999501, -5.633481712366999794, 7.451234046297000368 ) ) ;
#26061=CARTESIAN_POINT ( 'NONE',  ( 10.37373728961999930, -2.215269876326000364, 7.703982265807999497 ) ) ;
#26062=AXIS2_PLACEMENT_3D ( 'NONE', #19612, #20292, #57011 ) ;
#26064=CYLINDRICAL_SURFACE ( 'NONE', #53945, 1.350000000000000089 ) ;
#26068=CARTESIAN_POINT ( 'NONE',  ( 10.99245660749474141, -5.807287262094808611, -4.970960764622379457 ) ) ;
#26069=EDGE_LOOP ( 'NONE', ( #11767, #59169, #42308, #68160, #5689, #276 ) ) ;
#26073=FACE_OUTER_BOUND ( 'NONE', #62716, .T. ) ;
#26075=DIRECTION ( 'NONE',  ( -3.254772980312840162E-06, -0.9999999999757510638, -6.156644133330701524E-06 ) ) ;
#26078=CARTESIAN_POINT ( 'NONE',  ( 7.750036073563001615, -5.085252754069001568, 6.546627699621002883 ) ) ;
#26083=DIRECTION ( 'NONE',  ( 0.000000000000000000, -0.1333333333333049098, 0.9910712498212373989 ) ) ;
#26096=CARTESIAN_POINT ( 'NONE',  ( 7.512831853207000421, -5.524126964933000927, 6.910359834012999691 ) ) ;
#26107=CARTESIAN_POINT ( 'NONE',  ( 8.855418146794999501, -5.633481712366999794, 7.451234046297000368 ) ) ;
#26108=CARTESIAN_POINT ( 'NONE',  ( 9.221802827889566956, -2.874603711571219744, 6.749639981086952290 ) ) ;
#26111=VERTEX_POINT ( 'NONE', #38592 ) ;
#26118=DIRECTION ( 'NONE',  ( 0.000000000000000000, 0.000000000000000000, -1.000000000000000000 ) ) ;
#26127=CARTESIAN_POINT ( 'NONE',  ( 8.097451241187362925, -4.501375107734432390, 5.833995739002847181 ) ) ;
#26129=CARTESIAN_POINT ( 'NONE',  ( 11.01512623398999935, -8.057018824736999818, 6.941559373591999815 ) ) ;
#26139=CARTESIAN_POINT ( 'NONE',  ( 9.578311703535998589, -4.818302824158000597, -8.808202952968999355 ) ) ;
#26140=CARTESIAN_POINT ( 'NONE',  ( 10.39070086100999823, -3.082125293506999597, -4.654000461396999633 ) ) ;
#26150=CARTESIAN_POINT ( 'NONE',  ( 9.385311019873999072, -4.135077143711000325, 9.175520401071999288 ) ) ;
#26163=VERTEX_POINT ( 'NONE', #2234 ) ;
#26164=ORIENTED_EDGE ( 'NONE', *, *, #50321, .T. ) ;
#26167=CARTESIAN_POINT ( 'NONE',  ( 10.27427156480999848, -3.399999787207999447, 4.944156960757000618 ) ) ;
#26175=CARTESIAN_POINT ( 'NONE',  ( 10.98768521492000083, -5.299565686336999981, -4.945211137252000455 ) ) ;
#26186=VECTOR ( 'NONE', #22955, 1000.000000000000000 ) ;
#26191=CARTESIAN_POINT ( 'NONE',  ( 9.217200371204294029, -2.656565280586873357, 7.632967396875749877 ) ) ;
#26201=CARTESIAN_POINT ( 'NONE',  ( 10.26763456158959009, -5.237072593125339459, 8.927049273773194571 ) ) ;
#26205=DIRECTION ( 'NONE',  ( 1.000000000000000000, 0.000000000000000000, 0.000000000000000000 ) ) ;
#26210=FACE_OUTER_BOUND ( 'NONE', #16583, .T. ) ;
#26211=CARTESIAN_POINT ( 'NONE',  ( 9.053331853208000268, -5.618388245857000030, 7.727743016644000207 ) ) ;
#26217=CARTESIAN_POINT ( 'NONE',  ( 7.600254814611190568, -4.545917558585252038, 5.846023085849561873 ) ) ;
#26220=ORIENTED_EDGE ( 'NONE', *, *, #16130, .F. ) ;
#26235=CARTESIAN_POINT ( 'NONE',  ( 9.061090930683000977, -5.103946207352000108, -6.635696954776999945 ) ) ;
#26240=VECTOR ( 'NONE', #61700, 1000.000000000000000 ) ;
#26245=CARTESIAN_POINT ( 'NONE',  ( 9.611390067472999732, -3.334847606888000193, 5.869121315726000709 ) ) ;
#26247=B_SPLINE_CURVE_WITH_KNOTS ( 'NONE', 3,
 ( #21568, #64212, #43248, #33458, #32083, #38341, #22261, #5497, #17012, #37995, #54425, #54077, #38696, #6527, #27870, #64899, #600, #11087 ),
 .UNSPECIFIED., .F., .F.,
 ( 4, 2, 2, 2, 2, 2, 2, 2, 4 ),
 ( 0.000000000000000000, 0.1250000000000001665, 0.2500000000000003331, 0.3750000000000001665, 0.5000000000000000000, 0.6249999999999996669, 0.7499999999999994449, 0.8749999999999996669, 1.000000000000000000 ),
 .UNSPECIFIED. ) ;
#26254=CARTESIAN_POINT ( 'NONE',  ( 10.85685100254000091, -2.832432432432000269, -6.822293592207000934 ) ) ;
#26258=CARTESIAN_POINT ( 'NONE',  ( 9.260955151160263910, -2.777201709903842186, 6.918164468165489467 ) ) ;
#26264=CARTESIAN_POINT ( 'NONE',  ( 10.28315099603999982, -2.387772357283999725, 7.684266429524000408 ) ) ;
#26317=ORIENTED_EDGE ( 'NONE', *, *, #23600, .T. ) ;
#26322=CARTESIAN_POINT ( 'NONE',  ( 8.559020380274406037, -4.705862675926076655, 8.704770267039673826 ) ) ;
#26326=DIRECTION ( 'NONE',  ( 0.000000000000000000, 1.000000000000000000, 0.000000000000000000 ) ) ;
#26341=ORIENTED_EDGE ( 'NONE', *, *, #27795, .F. ) ;
#26348=CARTESIAN_POINT ( 'NONE',  ( 10.09454055528000005, -5.362855569781999954, -7.550030734599999960 ) ) ;
#26350=EDGE_CURVE ( 'NONE', #29839, #64219, #18994, .T. ) ;
#26354=FACE_OUTER_BOUND ( 'NONE', #26381, .T. ) ;
#26366=CARTESIAN_POINT ( 'NONE',  ( 8.332046967449000974, -2.867486995832002616, 6.314275746166007508 ) ) ;
#26369=CARTESIAN_POINT ( 'NONE',  ( 10.46432358320999967, -2.042767395367000027, 7.723698102088000006 ) ) ;
#26380=CARTESIAN_POINT ( 'NONE',  ( 7.749580121866000759, -3.139119547898000295, 6.460040744864000040 ) ) ;
#26381=EDGE_LOOP ( 'NONE', ( #37566, #24361, #62777, #27427, #17352, #45340, #35270, #63319, #67127, #49783, #48314, #12207, #32026, #6677, #37762 ) ) ;
#26384=CARTESIAN_POINT ( 'NONE',  ( 8.216851002544000693, -2.832432432432000269, 6.822293592207000934 ) ) ;
#26387=ORIENTED_EDGE ( 'NONE', *, *, #3989, .F. ) ;
#26392=LINE ( 'NONE', #21475, #45500 ) ;
#26395=ORIENTED_EDGE ( 'NONE', *, *, #55406, .T. ) ;
#26396=CARTESIAN_POINT ( 'NONE',  ( 9.687876499438001332, -5.912252057206999645, 7.772299417761000306 ) ) ;
#26400=CARTESIAN_POINT ( 'NONE',  ( 9.406706853206999952, -3.705847642455000202, 9.096432253453999195 ) ) ;
#26407=CARTESIAN_POINT ( 'NONE',  ( 10.98768491210000064, -8.067891622241001315, 6.818837029638999958 ) ) ;
#26410=CARTESIAN_POINT ( 'NONE',  ( 9.939319226872999735, -2.638101016021999978, 6.328632621050000573 ) ) ;
#26415=FACE_OUTER_BOUND ( 'NONE', #50151, .T. ) ;
#26424=VERTEX_POINT ( 'NONE', #10221 ) ;
#26426=ORIENTED_EDGE ( 'NONE', *, *, #59507, .F. ) ;
#26437=ORIENTED_EDGE ( 'NONE', *, *, #58779, .T. ) ;
#26443=CARTESIAN_POINT ( 'NONE',  ( 8.566230646795000681, -5.212258818969000451, 6.157189191035000064 ) ) ;
#26447=LINE ( 'NONE', #63489, #6807 ) ;
#26453=CARTESIAN_POINT ( 'NONE',  ( 7.866206853207000194, -4.580607464247000493, 9.213361409141999303 ) ) ;
#26458=EDGE_LOOP ( 'NONE', ( #4032, #32854, #5025, #30353 ) ) ;
#26468=CARTESIAN_POINT ( 'NONE',  ( 7.204799779090437006, -2.684882381560841580, 7.854227636469309992 ) ) ;
#26474=CARTESIAN_POINT ( 'NONE',  ( 8.473482780583216467, -2.321348858116770941, 6.962478315320627331 ) ) ;
#26489=CARTESIAN_POINT ( 'NONE',  ( 8.784973378479026707, -4.855539494230036723, 9.057509731918708340 ) ) ;
#26493=EDGE_LOOP ( 'NONE', ( #30054, #34886, #26632 ) ) ;
#26495=CARTESIAN_POINT ( 'NONE',  ( 7.839808059622000336, -3.084082018960999871, 9.259837032825000591 ) ) ;
#26507=ORIENTED_EDGE ( 'NONE', *, *, #28063, .F. ) ;
#26522=EDGE_CURVE ( 'NONE', #11630, #22321, #45152, .T. ) ;
#26534=AXIS2_PLACEMENT_3D ( 'NONE', #55832, #55485, #39062 ) ;
#26536=B_SPLINE_SURFACE_WITH_KNOTS ( 'NONE', 3, 3, ( 
 ( #40718, #8225, #7525, #23609 ),
 ( #44951, #19744, #66255, #14163 ),
 ( #18376, #24299, #29572, #39698 ),
 ( #50874, #2971, #8906, #66940 ),
 ( #13819, #29912, #35488, #3648 ),
 ( #51550, #24985, #46317, #41067 ),
 ( #12785, #5027, #63053, #4337 ),
 ( #62386, #25325, #67969, #25671 ),
 ( #35822, #42101, #26017, #9237 ),
 ( #20424, #15528, #21448, #31959 ),
 ( #14841, #68652, #47003, #36163 ) ),
 .UNSPECIFIED., .F., .F., .F.,
 ( 4, 1, 1, 1, 1, 1, 1, 1, 4 ),
 ( 4, 4 ),
 ( 0.5665910773458999738, 0.6250000000000000000, 0.6875000000000000000, 0.7500000000000000000, 0.8125000000000000000, 0.8750000000000000000, 0.9375000000000000000, 1.000000000000000000, 1.014356664780999839 ),
 ( -0.1686987264388999930, 1.168651125902999910 ),
 .UNSPECIFIED. ) ;
#26547=EDGE_CURVE ( 'NONE', #21198, #41719, #8087, .T. ) ;
#26556=CARTESIAN_POINT ( 'NONE',  ( 9.869049086607999399, -5.575175898444999945, 7.724300702620999104 ) ) ;
#26557=CARTESIAN_POINT ( 'NONE',  ( 7.165495559622000243, -2.688354259407999880, 8.140021027181001401 ) ) ;
#26563=CARTESIAN_POINT ( 'NONE',  ( 7.706178870840924233, -5.757700323609271642, 7.628119760989433118 ) ) ;
#26567=ORIENTED_EDGE ( 'NONE', *, *, #65651, .F. ) ;
#26571=AXIS2_PLACEMENT_3D ( 'NONE', #62568, #41940, #52076 ) ;
#26574=B_SPLINE_CURVE_WITH_KNOTS ( 'NONE', 3,
 ( #1600, #65909, #22228, #11388 ),
 .UNSPECIFIED., .F., .F.,
 ( 4, 4 ),
 ( 0.7873984553934968433, 1.000000000000000000 ),
 .UNSPECIFIED. ) ;
#26592=CARTESIAN_POINT ( 'NONE',  ( 9.555699158955999195, -2.440755924888999839, 6.680881588809999272 ) ) ;
#26609=ORIENTED_EDGE ( 'NONE', *, *, #57098, .F. ) ;
#26614=CARTESIAN_POINT ( 'NONE',  ( 9.758146639703001668, -2.901368778958000050, 6.555068849476000103 ) ) ;
#26632=ORIENTED_EDGE ( 'NONE', *, *, #9246, .T. ) ;
#26633=AXIS2_PLACEMENT_3D ( 'NONE', #67923, #30881, #3602 ) ;
#26646=CARTESIAN_POINT ( 'NONE',  ( 9.742016541512397154, -3.170522872755219712, -8.579511628985352800 ) ) ;
#26653=FACE_OUTER_BOUND ( 'NONE', #4977, .T. ) ;
#26654=CARTESIAN_POINT ( 'NONE',  ( 10.87274555961999845, -5.407608219159000029, -8.698392243238998844 ) ) ;
#26664=ORIENTED_EDGE ( 'NONE', *, *, #73, .T. ) ;
#26679=VERTEX_POINT ( 'NONE', #46522 ) ;
#26688=CARTESIAN_POINT ( 'NONE',  ( 8.475341021510246264, -5.350570349241358770, 7.499981640446112152 ) ) ;
#26698=CARTESIAN_POINT ( 'NONE',  ( 9.937415816209998809, -3.510658118802999716, -6.227041669085999764 ) ) ;
#26702=CARTESIAN_POINT ( 'NONE',  ( 8.191498616105999275, -3.399962740672999750, 6.146646623957999545 ) ) ;
#26704=CARTESIAN_POINT ( 'NONE',  ( 10.99698817424124364, -5.185245244840650081, 5.073517292121563216 ) ) ;
#26719=CARTESIAN_POINT ( 'NONE',  ( 11.27109998545999936, -5.469594811916000054, 8.504700858852999090 ) ) ;
#26720=CARTESIAN_POINT ( 'NONE',  ( 8.433148997460000018, -5.167567567567999731, 6.822293592207000934 ) ) ;
#26732=CARTESIAN_POINT ( 'NONE',  ( 5.500000000595999694, -0.4999999994045000173, 3.150000007847999939 ) ) ;
#26743=EDGE_LOOP ( 'NONE', ( #52653, #67465, #44739, #61912, #67836, #56786, #39941, #19513 ) ) ;
#26744=CARTESIAN_POINT ( 'NONE',  ( 10.13340376756999994, -5.653635692335999607, 6.501829690795999817 ) ) ;
#26747=CARTESIAN_POINT ( 'NONE',  ( 7.000000000000000000, -9.186881099820000784, 5.186879182879000183 ) ) ;
#26748=CARTESIAN_POINT ( 'NONE',  ( 8.443894353209000059, -2.905864338704999827, 8.940687151810998046 ) ) ;
#26751=ORIENTED_EDGE ( 'NONE', *, *, #54290, .T. ) ;
#26757=CARTESIAN_POINT ( 'NONE',  ( 8.156333095604772154, -3.177195612464926100, 6.222100672065804083 ) ) ;
#26759=CARTESIAN_POINT ( 'NONE',  ( 10.77962878203999963, -2.397503436487000261, 7.755423856053000442 ) ) ;
#26761=B_SPLINE_CURVE_WITH_KNOTS ( 'NONE', 3,
 ( #30529, #67569, #62337, #19343, #19695, #8857, #14454, #35774, #51842, #25278, #67918, #41363, #62672, #14792 ),
 .UNSPECIFIED., .F., .F.,
 ( 4, 2, 2, 2, 2, 2, 4 ),
 ( 0.1252897476283257872, 0.3125851014321937016, 0.4998804552360616160, 0.5935281321379953789, 0.6871758090399291419, 0.7808234859418630158, 0.8744711628437967788 ),
 .UNSPECIFIED. ) ;
#26765=ORIENTED_EDGE ( 'NONE', *, *, #53572, .T. ) ;
#26767=CARTESIAN_POINT ( 'NONE',  ( 10.84160444037999937, -2.641264320582999758, -7.444904971031999885 ) ) ;
#26776=EDGE_LOOP ( 'NONE', ( #27811, #61653, #12450, #49470, #61255 ) ) ;
#26784=CARTESIAN_POINT ( 'NONE',  ( 10.90000000000000036, -0.2999999999999999889, 9.662944685757000940 ) ) ;
#26792=CARTESIAN_POINT ( 'NONE',  ( 9.208105646793001142, -5.057079407184000175, 8.967634647348999621 ) ) ;
#26795=CARTESIAN_POINT ( 'NONE',  ( 7.844724262280000637, -4.719412258162999585, 6.357657668295000342 ) ) ;
#26797=CARTESIAN_POINT ( 'NONE',  ( 10.99999999997000089, -4.000000000000000000, -7.500000000000000000 ) ) ;
#26805=CARTESIAN_POINT ( 'NONE',  ( 8.379706853209000883, -4.282999948634999221, 9.286791354293999490 ) ) ;
#26822=CARTESIAN_POINT ( 'NONE',  ( 8.544290774020575796, -3.362597475556388105, 5.881642975893083936 ) ) ;
#26833=EDGE_CURVE ( 'NONE', #57248, #12470, #54048, .T. ) ;
#26850=CARTESIAN_POINT ( 'NONE',  ( 10.11501430098003773, -5.350017391163235381, -7.499999134156934311 ) ) ;
#26859=DIRECTION ( 'NONE',  ( 0.000000000000000000, 1.000000000000000000, 0.000000000000000000 ) ) ;
#26870=CARTESIAN_POINT ( 'NONE',  ( 10.77088239901999955, -5.264131025895999905, -4.839453784185999474 ) ) ;
#26874=B_SPLINE_CURVE_WITH_KNOTS ( 'NONE', 3,
 ( #36161, #25324, #4335, #25670, #20423 ),
 .UNSPECIFIED., .F., .F.,
 ( 4, 1, 4 ),
 ( 0.000000000000000000, 0.5000000000000000000, 1.000000000000000000 ),
 .UNSPECIFIED. ) ;
#26883=CARTESIAN_POINT ( 'NONE',  ( 10.17905590578999941, -2.899999999999999911, 6.571291218949999902 ) ) ;
#26895=CARTESIAN_POINT ( 'NONE',  ( 10.85685100254000091, -2.832432432432000269, -6.822293592207000934 ) ) ;
#26901=CARTESIAN_POINT ( 'NONE',  ( 9.423521818475000700, -4.993993578306000103, 8.578110568283999982 ) ) ;
#26902=CARTESIAN_POINT ( 'NONE',  ( 7.384456853207000293, -3.346260729029000291, 6.002247316312999459 ) ) ;
#26906=CARTESIAN_POINT ( 'NONE',  ( 10.75101814679000078, -2.478465696309000155, -7.438303690845000204 ) ) ;
#26907=CARTESIAN_POINT ( 'NONE',  ( 7.754585461271813251, -5.335985935492750798, 8.613681351317808321 ) ) ;
#26908=CARTESIAN_POINT ( 'NONE',  ( 10.24961784311999935, -4.184221496660999406, 9.286877953065999947 ) ) ;
#26925=VECTOR ( 'NONE', #29366, 1000.000000000000000 ) ;
#26932=CARTESIAN_POINT ( 'NONE',  ( 11.03855816545999957, -2.974093234901999949, 8.716125417860000724 ) ) ;
#26934=AXIS2_PLACEMENT_3D ( 'NONE', #30246, #51216, #13481 ) ;
#26939=ADVANCED_FACE ( 'NONE', ( #36981 ), #4454, .F. ) ;
#26946=AXIS2_PLACEMENT_3D ( 'NONE', #1724, #12219, #55212 ) ;
#26949=CARTESIAN_POINT ( 'NONE',  ( 9.243268584279421773, -2.683782748811717855, 7.201188049543101322 ) ) ;
#26969=CARTESIAN_POINT ( 'NONE',  ( 10.90000000164000049, -2.899999999992999733, 5.160242739040000082 ) ) ;
#26972=DIRECTION ( 'NONE',  ( 1.000000000000000000, 0.000000000000000000, 0.000000000000000000 ) ) ;
#26975=DIRECTION ( 'NONE',  ( 1.000000000000000000, 0.000000000000000000, 0.000000000000000000 ) ) ;
#26991=CARTESIAN_POINT ( 'NONE',  ( 10.14521814679000045, -3.576528389491000048, -8.962725485696999783 ) ) ;
#26995=EDGE_CURVE ( 'NONE', #52199, #59620, #19403, .T. ) ;
#26997=EDGE_CURVE ( 'NONE', #33729, #7601, #11106, .T. ) ;
#27004=EDGE_LOOP ( 'NONE', ( #37241, #66283, #2785, #12883, #16038 ) ) ;
#27015=B_SPLINE_CURVE_WITH_KNOTS ( 'NONE', 3,
 ( #34850, #66302, #55481, #6884 ),
 .UNSPECIFIED., .F., .F.,
 ( 4, 4 ),
 ( 0.000000000000000000, 1.000000000000000000 ),
 .UNSPECIFIED. ) ;
#27021=ORIENTED_EDGE ( 'NONE', *, *, #21765, .T. ) ;
#27026=CARTESIAN_POINT ( 'NONE',  ( 10.90437356726000040, -2.900476673752999890, 5.132566153004000320 ) ) ;
#27028=CARTESIAN_POINT ( 'NONE',  ( 8.331682137624000006, -5.101289325373999262, 6.607176193198000647 ) ) ;
#27040=CARTESIAN_POINT ( 'NONE',  ( 10.44486180556999955, -4.964082081645000422, -9.083599939499999110 ) ) ;
#27053=ORIENTED_EDGE ( 'NONE', *, *, #7400, .F. ) ;
#27055=CARTESIAN_POINT ( 'NONE',  ( 9.256662271119999730, -4.025830307267999508, 9.295859242339000517 ) ) ;
#27056=EDGE_CURVE ( 'NONE', #49271, #20862, #60368, .T. ) ;
#27059=CARTESIAN_POINT ( 'NONE',  ( 5.600000000706000236, 0.8000000000000000444, 3.149999999999999911 ) ) ;
#27060=CARTESIAN_POINT ( 'NONE',  ( 9.409308287954999628, -2.634700736117999931, 8.920302460802998823 ) ) ;
#27067=DIRECTION ( 'NONE',  ( -0.03487031647297116066, 1.485882206239048391E-07, -0.9993918455886323660 ) ) ;
#27071=CARTESIAN_POINT ( 'NONE',  ( 8.220491098714299838, -2.863432619444471250, 6.768885785334203931 ) ) ;
#27079=CARTESIAN_POINT ( 'NONE',  ( 5.500000000000000000, -1.300000000000000044, -9.662944685757000940 ) ) ;
#27080=CARTESIAN_POINT ( 'NONE',  ( 7.975339216757299177, -5.350090185752664595, 7.499980949462679014 ) ) ;
#27081=CYLINDRICAL_SURFACE ( 'NONE', #56289, 0.5000000000000000000 ) ;
#27083=AXIS2_PLACEMENT_3D ( 'NONE', #23201, #48740, #497 ) ;
#27086=CARTESIAN_POINT ( 'NONE',  ( 10.50244460374000077, -2.268915328469999881, 7.824865002012999504 ) ) ;
#27090=CARTESIAN_POINT ( 'NONE',  ( 8.983793146794999629, -3.979464503892999439, 9.134080454305001595 ) ) ;
#27098=CARTESIAN_POINT ( 'NONE',  ( 9.910792656537999790, -3.869344906782000049, 5.882544796414999944 ) ) ;
#27105=ORIENTED_EDGE ( 'NONE', *, *, #64563, .T. ) ;
#27113=CARTESIAN_POINT ( 'NONE',  ( 7.000000000000000000, 0.000000000000000000, 0.000000000000000000 ) ) ;
#27116=CARTESIAN_POINT ( 'NONE',  ( 9.314550945856780118, -4.223514815909876319, 9.228465502814891863 ) ) ;
#27126=CARTESIAN_POINT ( 'NONE',  ( 9.400463768223922045, -5.265153800075048629, -8.707768634079092962 ) ) ;
#27132=CARTESIAN_POINT ( 'NONE',  ( 9.250897313459001126, -4.135077143711000325, 9.175520401071999288 ) ) ;
#27144=CARTESIAN_POINT ( 'NONE',  ( 8.572269353210000276, -2.606998386752999775, 6.345764833140000505 ) ) ;
#27157=CARTESIAN_POINT ( 'NONE',  ( 7.215222283847193552, -2.650817894710479905, 7.677089056594191163 ) ) ;
#27162=CARTESIAN_POINT ( 'NONE',  ( 8.427572861040259156, -2.321778634991549239, 7.972824082824569558 ) ) ;
#27164=VERTEX_POINT ( 'NONE', #39388 ) ;
#27170=DIRECTION ( 'NONE',  ( 0.000000000000000000, -1.000000000000000000, 0.000000000000000000 ) ) ;
#27174=CARTESIAN_POINT ( 'NONE',  ( 8.767879976495999372, -3.394455611366999914, -6.293427637271999942 ) ) ;
#27178=ORIENTED_EDGE ( 'NONE', *, *, #19823, .F. ) ;
#27185=ORIENTED_EDGE ( 'NONE', *, *, #19282, .F. ) ;
#27187=EDGE_CURVE ( 'NONE', #49213, #16713, #28564, .T. ) ;
#27200=DIRECTION ( 'NONE',  ( -1.000000000000000000, 3.552713678845000257E-14, -5.329070518267999577E-14 ) ) ;
#27203=CARTESIAN_POINT ( 'NONE',  ( 10.68375832677999959, -4.547311397465000127, -8.749131152219000285 ) ) ;
#27207=ORIENTED_EDGE ( 'NONE', *, *, #42791, .F. ) ;
#27213=CIRCLE ( 'NONE', #12695, 1.549999999999999600 ) ;
#27240=CARTESIAN_POINT ( 'NONE',  ( 10.92717634842000152, -5.023656093247000243, 8.718039182945998888 ) ) ;
#27241=CARTESIAN_POINT ( 'NONE',  ( 8.951355646795001064, -2.821866379289000193, 6.127148604720000336 ) ) ;
#27243=CARTESIAN_POINT ( 'NONE',  ( 9.003209435575312725, -2.902877702503883661, 6.186420784434704778 ) ) ;
#27245=LINE ( 'NONE', #17441, #20976 ) ;
#27246=CARTESIAN_POINT ( 'NONE',  ( 10.01676935320999995, -4.324998011277000565, -9.154075058362000306 ) ) ;
#27247=CARTESIAN_POINT ( 'NONE',  ( 7.897386357334326590, -2.614547605125981722, 8.551323849536911936 ) ) ;
#27248=CARTESIAN_POINT ( 'NONE',  ( 10.52638330645999964, -2.451090818816000105, 6.282756943804999494 ) ) ;
#27255=VERTEX_POINT ( 'NONE', #14201 ) ;
#27265=CARTESIAN_POINT ( 'NONE',  ( 7.726441940376999717, -2.630475685621000093, 6.995953627589999613 ) ) ;
#27274=CARTESIAN_POINT ( 'NONE',  ( 9.520803773887999810, -3.270557529354000348, 5.711489293131999823 ) ) ;
#27283=AXIS2_PLACEMENT_3D ( 'NONE', #68256, #31226, #15482 ) ;
#27308=CARTESIAN_POINT ( 'NONE',  ( 11.10000000009000054, -5.300000000088999741, -6.571291220400000022 ) ) ;
#27313=CIRCLE ( 'NONE', #23968, 1.549999999999999156 ) ;
#27321=ORIENTED_EDGE ( 'NONE', *, *, #13551, .F. ) ;
#27325=CARTESIAN_POINT ( 'NONE',  ( 9.700348830567069314, -3.823367932526878121, -8.850089092130223989 ) ) ;
#27333=CARTESIAN_POINT ( 'NONE',  ( 10.41025564679000048, -4.690690303276999984, -6.142863315966000215 ) ) ;
#27338=B_SPLINE_CURVE_WITH_KNOTS ( 'NONE', 3,
 ( #8811, #30152, #40970, #62294 ),
 .UNSPECIFIED., .F., .F.,
 ( 4, 4 ),
 ( 0.8746820087829817458, 1.000000000000000000 ),
 .UNSPECIFIED. ) ;
#27354=EDGE_CURVE ( 'NONE', #26163, #4537, #56922, .T. ) ;
#27355=CARTESIAN_POINT ( 'NONE',  ( 10.74708735964999917, -5.603138702306000418, -6.963343193308999979 ) ) ;
#27379=CARTESIAN_POINT ( 'NONE',  ( 10.05204995789999955, -2.669899884077999719, -8.791535702747999892 ) ) ;
#27383=PLANE ( 'NONE',  #48641 ) ;
#27387=EDGE_CURVE ( 'NONE', #67334, #23850, #67317, .T. ) ;
#27392=CARTESIAN_POINT ( 'NONE',  ( 9.209122513651813335, -5.100000000000000533, 6.320295141290149132 ) ) ;
#27395=CARTESIAN_POINT ( 'NONE',  ( 10.46432358320999967, -2.042767395367000027, 7.723698102088000006 ) ) ;
#27398=CARTESIAN_POINT ( 'NONE',  ( 10.15402496696000156, -5.267980706381999667, 5.992344456606999437 ) ) ;
#27399=DIRECTION ( 'NONE',  ( -6.259113923818999724E-11, 6.259176727233999437E-11, 1.000000000000000000 ) ) ;
#27405=B_SPLINE_SURFACE_WITH_KNOTS ( 'NONE', 3, 3, ( 
 ( #35534, #56854, #8951, #25031, #30292, #30975, #36553, #51595, #46016, #46363, #16510, #436, #32269, #19789, #24693, #58818, #21750, #30626, #62431, #4033, #3692, #19441, #35869, #25372, #14207, #46709, #14887, #59160, #51937, #10925, #41459, #68013, #20130, #43084, #64389 ),
 ( #37839, #62766, #52287, #20470, #36208, #57525, #11264, #4381, #25716, #32601, #47050, #67323, #40765, #62087, #33643, #6359, #60896, #39225, #43441, #13012, #43783, #11602, #32945, #48677, #18250, #27705, #17559, #66131, #54959, #44828, #16852, #38175, #59504, #49022, #54257 ),
 ( #28750, #60550, #12657, #7061, #1128, #55307, #17907, #49358, #65079, #39572, #27355, #22096, #22442, #23489, #1820, #34340, #38529, #28397, #782, #17199, #28049, #59851, #11958, #65783, #7404, #49713, #6015, #64737, #6709, #23140, #44490, #33295, #60207, #33988, #44137 ),
 ( #54611, #50065, #1472, #2173, #22789, #65436, #38885, #12310, #45851, #56690, #14387, #8789, #46195, #50754, #3199, #35029, #62600, #67160, #29098, #45170, #67506, #40263, #39926, #50408, #61244, #61583, #51774, #24867, #57024, #2508, #9124, #29447, #35707, #19272, #30463 ) ),
 .UNSPECIFIED., .F., .F., .F.,
 ( 4, 4 ),
 ( 4, 1, 1, 1, 1, 1, 1, 1, 1, 1, 1, 1, 1, 1, 1, 1, 1, 1, 1, 1, 1, 1, 1, 1, 1, 1, 1, 1, 1, 1, 1, 1, 4 ),
 ( -0.1039086239011999951, 1.103908623900999864 ),
 ( 0.1942321073450000157, 0.2199060843169000079, 0.2455800612886999967, 0.2712540382605999612, 0.2969280152323999777, 0.3226019922043000254, 0.3482759691761000420, 0.3739499461479999787, 0.3996239231197999953, 0.4252979000916999874, 0.4509718770635000040, 0.4766458540353999962, 0.5023198310072000128, 0.5279938079791000050, 0.5536677849509000771, 0.5793417619227999582, 0.6050157388945999193, 0.6306897158665000225, 0.6563636928382999836, 0.6820376698101999757, 0.7077116467820000478, 0.7333856237539000400, 0.7590596007256998901, 0.7847335776975999933, 0.8104075546693999543, 0.8360815316413000575, 0.8617555086131000186, 0.8874294855850000108, 0.9131034625568000829, 0.9387774395286999640, 0.9644514165004999251, 0.9901253934722999972, 1.015799370444000038 ),
 .UNSPECIFIED. ) ;
#27425=CARTESIAN_POINT ( 'NONE',  ( 10.52324012719000024, -3.325647021086999722, 5.689999163383999026 ) ) ;
#27427=ORIENTED_EDGE ( 'NONE', *, *, #35668, .T. ) ;
#27429=CARTESIAN_POINT ( 'NONE',  ( 8.096558059622999792, -5.061720701958000390, 5.824087910811999613 ) ) ;
#27432=ORIENTED_EDGE ( 'NONE', *, *, #4718, .T. ) ;
#27434=B_SPLINE_CURVE_WITH_KNOTS ( 'NONE', 3,
 ( #40870, #62194, #14314, #69155, #59016 ),
 .UNSPECIFIED., .F., .F.,
 ( 4, 1, 4 ),
 ( 0.000000000000000000, 0.5000000000000000000, 1.000000000000000000 ),
 .UNSPECIFIED. ) ;
#27439=CARTESIAN_POINT ( 'NONE',  ( 10.44080359545000114, -5.435731278187999393, 7.303630150377999009 ) ) ;
#27453=CARTESIAN_POINT ( 'NONE',  ( 9.327002446946540459, -3.954584633155211915, 9.239083166430416938 ) ) ;
#27455=CARTESIAN_POINT ( 'NONE',  ( 5.700000000000000178, 1.250000000000000000, 0.000000000000000000 ) ) ;
#27461=CARTESIAN_POINT ( 'NONE',  ( 10.65050275296000137, -5.200029647236999786, 5.937716681140000397 ) ) ;
#27465=VERTEX_POINT ( 'NONE', #13179 ) ;
#27468=CARTESIAN_POINT ( 'NONE',  ( 9.882266086202999844, -4.932716797830999589, 6.390980246320999925 ) ) ;
#27472=CARTESIAN_POINT ( 'NONE',  ( 7.667605646792000407, -5.638700495537999124, 8.266402903491000487 ) ) ;
#27485=CARTESIAN_POINT ( 'NONE',  ( 11.09461754388281740, -3.670987266758758416, -9.018203014671000162 ) ) ;
#27486=CARTESIAN_POINT ( 'NONE',  ( 8.641808059624999316, -2.933824946949000090, 8.496487880080000110 ) ) ;
#27490=CARTESIAN_POINT ( 'NONE',  ( 9.660601868375998436, -2.901236202253999696, -6.151180522693000086 ) ) ;
#27491=EDGE_CURVE ( 'NONE', #29320, #3964, #57516, .T. ) ;
#27494=ORIENTED_EDGE ( 'NONE', *, *, #62179, .T. ) ;
#27503=CARTESIAN_POINT ( 'NONE',  ( 8.386090224810864413, -2.789003059333644341, 8.749111205124165735 ) ) ;
#27507=B_SPLINE_CURVE_WITH_KNOTS ( 'NONE', 3,
 ( #28052, #11961, #55659, #22793, #39928, #54616, #34687, #2175, #50758, #39574, #29449, #44141, #65439, #17562, #60209, #38888, #66135, #7758, #33645 ),
 .UNSPECIFIED., .F., .F.,
 ( 4, 2, 2, 1, 2, 2, 2, 2, 2, 4 ),
 ( 0.000000000000000000, 0.1250000000000042188, 0.1875000000000060507, 0.2187500000000067168, 0.2343750000000068556, 0.2500000000000069944, 0.3750000000000019984, 0.4375000000000018874, 0.5000000000000017764, 1.000000000000000000 ),
 .UNSPECIFIED. ) ;
#27514=ORIENTED_EDGE ( 'NONE', *, *, #42100, .F. ) ;
#27516=CARTESIAN_POINT ( 'NONE',  ( 9.857734298427807573, -2.650109589709913838, -7.624707963951017575 ) ) ;
#27535=EDGE_CURVE ( 'NONE', #31977, #9447, #68344, .T. ) ;
#27541=VERTEX_POINT ( 'NONE', #53318 ) ;
#27545=CARTESIAN_POINT ( 'NONE',  ( 11.06133683778999988, -2.503914237677999921, -6.712780725818999983 ) ) ;
#27557=EDGE_CURVE ( 'NONE', #56639, #9679, #4374, .T. ) ;
#27565=LINE ( 'NONE', #26883, #21969 ) ;
#27570=EDGE_LOOP ( 'NONE', ( #21288, #2722, #13123, #15631 ) ) ;
#27583=CARTESIAN_POINT ( 'NONE',  ( 9.792562654643999664, -3.463427761954999795, 6.184385360914999907 ) ) ;
#27588=CARTESIAN_POINT ( 'NONE',  ( 10.43325685320999874, -5.596199512734999715, -8.042023143828998855 ) ) ;
#27589=CARTESIAN_POINT ( 'NONE',  ( 7.754496970723887550, -5.337279552285365547, 8.612131160001228025 ) ) ;
#27591=DIRECTION ( 'NONE',  ( 1.000000000000000000, 0.000000000000000000, 0.000000000000000000 ) ) ;
#27605=CYLINDRICAL_SURFACE ( 'NONE', #14883, 1.350000000000000089 ) ;
#27607=CARTESIAN_POINT ( 'NONE',  ( 9.266941940380000631, -3.049610585291000042, 6.392533570808999421 ) ) ;
#27610=CARTESIAN_POINT ( 'NONE',  ( 10.02887352605975124, -2.739120126747620620, -8.716523496102675850 ) ) ;
#27623=EDGE_CURVE ( 'NONE', #18837, #9447, #25365, .T. ) ;
#27632=CARTESIAN_POINT ( 'NONE',  ( 10.90000000000000036, -0.2999999999999999889, 4.902439024389999567 ) ) ;
#27642=CYLINDRICAL_SURFACE ( 'NONE', #24790, 1.350000000000000089 ) ;
#27685=CARTESIAN_POINT ( 'NONE',  ( 10.47111935320999976, -5.170637620872999385, -8.712950754783999940 ) ) ;
#27687=B_SPLINE_SURFACE_WITH_KNOTS ( 'NONE', 3, 3, ( 
 ( #56445, #8550, #40702, #62029, #14145, #19727, #8892, #30228, #3632, #24969, #62372, #10261, #36839, #9917, #52916, #113, #30907, #58158, #41733, #9567, #57459, #46646, #26348, #15514, #68634, #37177, #26698, #47331, #68988, #20755, #42083, #31595, #68289, #20408, #5359 ),
 ( #21430, #5013, #4320, #47677, #63038, #25655, #31942, #42766, #36488, #21101, #52220, #41396, #64074, #15847, #52565, #42426, #4661, #46987, #48013, #63734, #58498, #10601, #53254, #16193, #31255, #37516, #58841, #15165, #57809, #10949, #51875, #3971, #25308, #26000, #67953 ),
 ( #20069, #63392, #62704, #14824, #36147, #6384, #1848, #23165, #37863, #44513, #60233, #33321, #38205, #48705, #59187, #28425, #28073, #49384, #1499, #65106, #54639, #59533, #22817, #6733, #808, #22124, #11983, #33668, #44165, #12336, #53938, #65808, #43811, #64414, #17231 ),
 ( #38554, #43467, #27735, #17933, #39251, #11288, #60576, #54987, #65461, #11629, #64760, #59876, #17584, #32293, #7083, #5698, #53601, #38910, #49739, #16878, #27040, #48351, #458, #21775, #32969, #54282, #43111, #16537, #32629, #6041, #27379, #49047, #1155, #22464, #20587 ) ),
 .UNSPECIFIED., .F., .F., .F.,
 ( 4, 4 ),
 ( 4, 1, 1, 1, 1, 1, 1, 1, 1, 1, 1, 1, 1, 1, 1, 1, 1, 1, 1, 1, 1, 1, 1, 1, 1, 1, 1, 1, 1, 1, 1, 1, 4 ),
 ( -0.1039086239011999951, 1.103908623900999864 ),
 ( 0.1942321073450000157, 0.2199060843169000079, 0.2455800612886999967, 0.2712540382605999612, 0.2969280152323999777, 0.3226019922043000254, 0.3482759691761000420, 0.3739499461479999787, 0.3996239231197999953, 0.4252979000916999874, 0.4509718770635000040, 0.4766458540353999962, 0.5023198310072000128, 0.5279938079791000050, 0.5536677849509000771, 0.5793417619227999582, 0.6050157388945999193, 0.6306897158665000225, 0.6563636928382999836, 0.6820376698101999757, 0.7077116467820000478, 0.7333856237539000400, 0.7590596007256998901, 0.7847335776975999933, 0.8104075546693999543, 0.8360815316413000575, 0.8617555086131000186, 0.8874294855850000108, 0.9131034625568000829, 0.9387774395286999640, 0.9644514165004999251, 0.9901253934722999972, 1.015799370444000038 ),
 .UNSPECIFIED. ) ;
#27688=CARTESIAN_POINT ( 'NONE',  ( 9.707733921870000060, -2.624754973437999794, -6.486841649805000110 ) ) ;
#27690=FACE_OUTER_BOUND ( 'NONE', #2008, .T. ) ;
#27692=CARTESIAN_POINT ( 'NONE',  ( 11.03776249210999971, -8.050323671732000363, -6.914613055281999543 ) ) ;
#27705=CARTESIAN_POINT ( 'NONE',  ( 10.06728329455999926, -4.192861215955000276, -5.985050974557999837 ) ) ;
#27709=EDGE_CURVE ( 'NONE', #66543, #12955, #57783, .T. ) ;
#27712=B_SPLINE_CURVE_WITH_KNOTS ( 'NONE', 3,
 ( #63426, #57157, #10295, #9601 ),
 .UNSPECIFIED., .F., .F.,
 ( 4, 4 ),
 ( 0.000000000000000000, 1.000000000000000000 ),
 .UNSPECIFIED. ) ;
#27719=FACE_OUTER_BOUND ( 'NONE', #56002, .T. ) ;
#27721=CARTESIAN_POINT ( 'NONE',  ( 10.51654446536000087, -4.930670681812999945, 8.573593359022000371 ) ) ;
#27722=VECTOR ( 'NONE', #64766, 1000.000000000000000 ) ;
#27727=DIRECTION ( 'NONE',  ( 0.000000000000000000, 1.000000000000000000, 0.000000000000000000 ) ) ;
#27735=CARTESIAN_POINT ( 'NONE',  ( 11.15192313136999935, -2.359310578948000003, -6.636692315558000210 ) ) ;
#27738=FACE_OUTER_BOUND ( 'NONE', #25418, .T. ) ;
#27740=DIRECTION ( 'NONE',  ( 1.000000000000000000, 0.000000000000000000, 0.000000000000000000 ) ) ;
#27746=CARTESIAN_POINT ( 'NONE',  ( 11.04200385643000182, -2.754971892945000000, 5.031215070518999966 ) ) ;
#27751=CARTESIAN_POINT ( 'NONE',  ( 9.843726350706999639, -4.115123626494000320, 9.466607949400000166 ) ) ;
#27754=CARTESIAN_POINT ( 'NONE',  ( 9.199609130449999839, -2.551382302226000487, 7.536606162076999738 ) ) ;
#27764=DIRECTION ( 'NONE',  ( -1.000000000000000000, -4.609710477022999584E-09, -1.269678721256999984E-09 ) ) ;
#27782=ORIENTED_EDGE ( 'NONE', *, *, #5762, .T. ) ;
#27783=CARTESIAN_POINT ( 'NONE',  ( 11.04783424078000031, -2.764605797469000148, 5.041477660832000218 ) ) ;
#27793=CARTESIAN_POINT ( 'NONE',  ( 6.799999999999999822, 0.000000000000000000, 0.000000000000000000 ) ) ;
#27795=EDGE_CURVE ( 'NONE', #61758, #28902, #34682, .T. ) ;
#27811=ORIENTED_EDGE ( 'NONE', *, *, #58396, .F. ) ;
#27819=CARTESIAN_POINT ( 'NONE',  ( 11.25041341105000114, -5.730771985297000271, 8.122672103119001008 ) ) ;
#27828=CARTESIAN_POINT ( 'NONE',  ( 10.31668414895000119, -3.819528725844000494, 6.062183754159999438 ) ) ;
#27831=DIRECTION ( 'NONE',  ( -0.7071067811865605623, 0.09428090767661463645, 0.7007932009142605612 ) ) ;
#27853=CARTESIAN_POINT ( 'NONE',  ( 10.22514748322304534, -2.649941783575446408, 7.500008211948054004 ) ) ;
#27859=CARTESIAN_POINT ( 'NONE',  ( 8.461280570003118839, -2.261174139539910311, 7.238226757569249159 ) ) ;
#27864=CARTESIAN_POINT ( 'NONE',  ( 10.01532628870999986, -4.946995631616999844, 8.559221361189001342 ) ) ;
#27870=CARTESIAN_POINT ( 'NONE',  ( 10.33455242540051522, -5.771779017986490068, -7.375668094431187427 ) ) ;
#27871=CARTESIAN_POINT ( 'NONE',  ( 8.829015684063998393, -3.399013800391000206, -6.242130679267000382 ) ) ;
#27873=CARTESIAN_POINT ( 'NONE',  ( 8.886105992892519012, -2.780583821594381888, 8.755311148983734526 ) ) ;
#27874=CARTESIAN_POINT ( 'NONE',  ( 9.428197172113431890, -5.125396288428772706, 6.749639981086940743 ) ) ;
#27877=EDGE_CURVE ( 'NONE', #9091, #26424, #55188, .T. ) ;
#27900=CARTESIAN_POINT ( 'NONE',  ( 10.81362580514000094, -3.876947229615999913, -9.022210119840998743 ) ) ;
#27913=B_SPLINE_CURVE_WITH_KNOTS ( 'NONE', 3,
 ( #67623, #14845, #36167, #13487, #51222 ),
 .UNSPECIFIED., .F., .F.,
 ( 4, 1, 4 ),
 ( 0.000000000000000000, 0.5000000000000000000, 1.000000000000000000 ),
 .UNSPECIFIED. ) ;
#27916=EDGE_LOOP ( 'NONE', ( #35808, #50644, #61867, #68399, #12045 ) ) ;
#27922=ORIENTED_EDGE ( 'NONE', *, *, #68032, .T. ) ;
#27934=CARTESIAN_POINT ( 'NONE',  ( 10.20319453770999907, -3.421758889707999796, 6.017729046583999875 ) ) ;
#27939=CARTESIAN_POINT ( 'NONE',  ( 9.978906853208000527, -5.007779786185999171, -8.772596342864998675 ) ) ;
#27941=CARTESIAN_POINT ( 'NONE',  ( 7.746254512012610505, -5.449976221991329695, 8.461014486623254172 ) ) ;
#27942=CARTESIAN_POINT ( 'NONE',  ( 10.89874164595999950, -2.834836218627000193, 9.088455567997000273 ) ) ;
#27949=ORIENTED_EDGE ( 'NONE', *, *, #38538, .T. ) ;
#27957=CARTESIAN_POINT ( 'NONE',  ( 11.09999999999999964, -6.519062740977999759, -5.524218123981000872 ) ) ;
#27963=CARTESIAN_POINT ( 'NONE',  ( 10.03827017495050100, -2.603767608621661900, -8.557743501763278360 ) ) ;
#27965=CARTESIAN_POINT ( 'NONE',  ( 11.08729972629000038, -2.258669075224000178, -7.034582301298999418 ) ) ;
#28023=DIRECTION ( 'NONE',  ( 1.000000000000000000, 0.000000000000000000, 0.000000000000000000 ) ) ;
#28032=CARTESIAN_POINT ( 'NONE',  ( 10.39539435320999949, -5.667179153637999178, -7.250689665673000661 ) ) ;
#28036=ORIENTED_EDGE ( 'NONE', *, *, #42391, .T. ) ;
#28045=DIRECTION ( 'NONE',  ( 0.000000000000000000, 1.000000000000000000, 0.000000000000000000 ) ) ;
#28049=CARTESIAN_POINT ( 'NONE',  ( 10.35427551197999918, -4.879111827962000270, -8.944027914303999793 ) ) ;
#28052=CARTESIAN_POINT ( 'NONE',  ( 10.90453766415000025, -2.900310535872000273, -5.130381900875999435 ) ) ;
#28057=CARTESIAN_POINT ( 'NONE',  ( 10.42861756900999914, -5.068632498314999069, 4.618459570084000099 ) ) ;
#28059=CARTESIAN_POINT ( 'NONE',  ( 10.27427156480999848, -3.399999787207999447, 4.944156960757000618 ) ) ;
#28063=EDGE_CURVE ( 'NONE', #51958, #53568, #65353, .T. ) ;
#28073=CARTESIAN_POINT ( 'NONE',  ( 10.51140025105000042, -2.326718149302000160, -7.741209600718000239 ) ) ;
#28077=CARTESIAN_POINT ( 'NONE',  ( 10.87751262143000019, -2.899999999999999911, 6.466455373849333554 ) ) ;
#28085=CARTESIAN_POINT ( 'NONE',  ( 9.317462135714000837, -5.100000000000000533, 6.571291218949999902 ) ) ;
#28088=CARTESIAN_POINT ( 'NONE',  ( 11.02286109245999945, -2.398753588646000079, 6.352476128646999065 ) ) ;
#28092=CARTESIAN_POINT ( 'NONE',  ( 10.19256470245000123, -2.560274838243000062, 7.664550593243999899 ) ) ;
#28093=CARTESIAN_POINT ( 'NONE',  ( 9.629471092178999214, -5.100000000000000533, 6.152188490330000370 ) ) ;
#28109=CARTESIAN_POINT ( 'NONE',  ( 7.496528476645853090, -5.315361133063865928, 7.854106854282135508 ) ) ;
#28116=LINE ( 'NONE', #50470, #532 ) ;
#28130=CARTESIAN_POINT ( 'NONE',  ( 9.758146639703001668, -2.901368778958000050, 6.555068849476000103 ) ) ;
#28146=CARTESIAN_POINT ( 'NONE',  ( 8.057875016312998184, -4.641725571029997610, 6.225038937488997171 ) ) ;
#28148=CARTESIAN_POINT ( 'NONE',  ( 8.267706852541074625, -5.045576645684537453, 6.407495147014386383 ) ) ;
#28152=DIRECTION ( 'NONE',  ( -0.9999999999999997780, -1.366956391494999762E-09, 2.239632587909999191E-08 ) ) ;
#28161=CARTESIAN_POINT ( 'NONE',  ( 10.68904248846000016, -2.568964727443000307, 7.728094434513999467 ) ) ;
#28163=CARTESIAN_POINT ( 'NONE',  ( 8.411456853209999807, -3.882020254083999866, 5.870054788755000530 ) ) ;
#28167=FACE_OUTER_BOUND ( 'NONE', #27916, .T. ) ;
#28181=CARTESIAN_POINT ( 'NONE',  ( 10.21160513988073149, -3.634030556546635093, -8.817876221680798210 ) ) ;
#28187=ORIENTED_EDGE ( 'NONE', *, *, #58349, .T. ) ;
#28195=ADVANCED_FACE ( 'NONE', ( #63885 ), #64573, .F. ) ;
#28197=CARTESIAN_POINT ( 'NONE',  ( 9.096071945540000314, -5.102479135096000817, -6.621020973615999061 ) ) ;
#28204=CARTESIAN_POINT ( 'NONE',  ( 9.957462135714001406, -5.100000000000000533, -6.571291218949999902 ) ) ;
#28211=CARTESIAN_POINT ( 'NONE',  ( 10.90000000011000125, -5.100000000110999743, 6.571291220762999430 ) ) ;
#28236=CARTESIAN_POINT ( 'NONE',  ( 10.99693800072000016, -2.980603239157999962, -6.418614998350999912 ) ) ;
#28239=CARTESIAN_POINT ( 'NONE',  ( 10.90000000000000036, -4.000000000000000000, -7.500000000000000000 ) ) ;
#28240=ORIENTED_EDGE ( 'NONE', *, *, #15162, .F. ) ;
#28244=CARTESIAN_POINT ( 'NONE',  ( 10.31905590579000176, -2.899999999999999911, -6.571291218949999902 ) ) ;
#28254=CARTESIAN_POINT ( 'NONE',  ( 7.758191940376999440, -5.797088532631000213, 8.340479314546998424 ) ) ;
#28255=CARTESIAN_POINT ( 'NONE',  ( 9.573145925901000552, -2.133039813254999917, -7.346564890486999566 ) ) ;
#28268=ORIENTED_EDGE ( 'NONE', *, *, #15501, .F. ) ;
#28272=CARTESIAN_POINT ( 'NONE',  ( 9.945535518573000999, -2.906050966242999856, 8.880386511481999534 ) ) ;
#28273=CARTESIAN_POINT ( 'NONE',  ( 8.834370559623998531, -4.141908960411000429, 6.047561724438000219 ) ) ;
#28277=CARTESIAN_POINT ( 'NONE',  ( 10.96333185321000059, -5.283547384770999500, -8.592770849731000027 ) ) ;
#28278=CARTESIAN_POINT ( 'NONE',  ( 8.089012611369920336, -4.321942129502657437, 5.789925683486281116 ) ) ;
#28279=AXIS2_PLACEMENT_3D ( 'NONE', #23309, #18069, #12472 ) ;
#28280=CARTESIAN_POINT ( 'NONE',  ( 9.533427734455999669, -2.564762519363000148, 6.150594768287000136 ) ) ;
#28281=CARTESIAN_POINT ( 'NONE',  ( 9.951054409601857387, -5.324155905473885397, 7.941945900372265221 ) ) ;
#28296=ORIENTED_EDGE ( 'NONE', *, *, #21304, .T. ) ;
#28305=CARTESIAN_POINT ( 'NONE',  ( 11.00589466765999802, -3.012766713855000056, 5.961506477028999385 ) ) ;
#28326=VERTEX_POINT ( 'NONE', #52717 ) ;
#28329=CARTESIAN_POINT ( 'NONE',  ( 8.455992358812000731, -5.100000000000000533, 6.571291218949999902 ) ) ;
#28331=AXIS2_PLACEMENT_3D ( 'NONE', #36305, #57622, #9725 ) ;
#28334=ORIENTED_EDGE ( 'NONE', *, *, #67572, .T. ) ;
#28336=VECTOR ( 'NONE', #66320, 1000.000000000000000 ) ;
#28347=CARTESIAN_POINT ( 'NONE',  ( 10.99999999997000089, -4.000000000000000000, 7.500000000000000000 ) ) ;
#28349=B_SPLINE_CURVE_WITH_KNOTS ( 'NONE', 3,
 ( #51524, #46290, #19717, #11276 ),
 .UNSPECIFIED., .F., .F.,
 ( 4, 4 ),
 ( 0.000000000000000000, 1.000000000000000000 ),
 .UNSPECIFIED. ) ;
#28367=DIRECTION ( 'NONE',  ( 0.5000000000000169864, 0.000000000000000000, 0.8660254037844288266 ) ) ;
#28370=EDGE_LOOP ( 'NONE', ( #58672, #18991, #16529, #55354 ) ) ;
#28373=LINE ( 'NONE', #53887, #49835 ) ;
#28376=DIRECTION ( 'NONE',  ( 0.000000000000000000, -0.1333333333333049375, -0.9910712498212375099 ) ) ;
#28377=CARTESIAN_POINT ( 'NONE',  ( 11.05391814679000184, -5.159486550382999859, -8.487149456222999433 ) ) ;
#28391=CARTESIAN_POINT ( 'NONE',  ( 9.679055905794999859, -2.899999999999999911, 6.571291218949999902 ) ) ;
#28396=CARTESIAN_POINT ( 'NONE',  ( 10.71685100253999856, -2.832432432432000269, 6.822293592207000934 ) ) ;
#28397=CARTESIAN_POINT ( 'NONE',  ( 10.47211906628000122, -2.640759929160000130, -8.505246563374999624 ) ) ;
#28411=CARTESIAN_POINT ( 'NONE',  ( 11.09424907396999949, -2.431867116603999790, 7.769513708858000633 ) ) ;
#28412=ORIENTED_EDGE ( 'NONE', *, *, #12892, .T. ) ;
#28418=CARTESIAN_POINT ( 'NONE',  ( 10.42499241036559532, -5.349775919985432004, 7.500001834605715345 ) ) ;
#28424=CARTESIAN_POINT ( 'NONE',  ( 8.331682137624000006, -5.101289325373999262, 6.607176193198000647 ) ) ;
#28425=CARTESIAN_POINT ( 'NONE',  ( 10.55068143582000140, -2.412180768165999911, -6.919582641217999708 ) ) ;
#28426=CARTESIAN_POINT ( 'NONE',  ( 7.000000000000000000, -9.186881182980000560, -5.186879035586000164 ) ) ;
#28427=LINE ( 'NONE', #49050, #8074 ) ;
#28429=CARTESIAN_POINT ( 'NONE',  ( 9.010799540956998754, -4.699533657262000119, -6.366989705700999203 ) ) ;
#28440=CARTESIAN_POINT ( 'NONE',  ( 7.443695762906002322, -3.525420668437998728, 6.642224720921002579 ) ) ;
#28443=CARTESIAN_POINT ( 'NONE',  ( 9.414314870535999802, -3.941041813398000304, 5.878346364186999295 ) ) ;
#28444=CARTESIAN_POINT ( 'NONE',  ( 9.857064864738445564, -3.288037737649794234, 9.126893253094490177 ) ) ;
#28449=B_SPLINE_CURVE_WITH_KNOTS ( 'NONE', 3,
 ( #9114, #36376, #9449, #31828 ),
 .UNSPECIFIED., .F., .F.,
 ( 4, 4 ),
 ( 0.000000000000000000, 1.000000000000000000 ),
 .UNSPECIFIED. ) ;
#28451=CARTESIAN_POINT ( 'NONE',  ( 9.856851002545999663, -2.832432432432000269, -6.822293592207000934 ) ) ;
#28452=DIRECTION ( 'NONE',  ( -1.000000000000000000, 0.000000000000000000, 0.000000000000000000 ) ) ;
#28455=LINE ( 'NONE', #7117, #20547 ) ;
#28459=CARTESIAN_POINT ( 'NONE',  ( 9.700159544970999193, -4.268950419651999617, -8.781589108989999559 ) ) ;
#28461=EDGE_LOOP ( 'NONE', ( #7559, #69043, #56208, #43583, #7110, #3347, #45717, #6645, #28867, #9739 ) ) ;
#28465=CARTESIAN_POINT ( 'NONE',  ( 9.970944094204998720, -5.100000000000000533, 6.571291218949999902 ) ) ;
#28480=CARTESIAN_POINT ( 'NONE',  ( 11.09166666666872203, -2.528771982360623838, 6.972956482935448896 ) ) ;
#28482=CARTESIAN_POINT ( 'NONE',  ( 11.08992739829000129, -5.210546653347999602, 8.327600405525998895 ) ) ;
#28499=CARTESIAN_POINT ( 'NONE',  ( 9.382379370190513157, -2.850576913252966360, 8.805889684294008646 ) ) ;
#28519=CARTESIAN_POINT ( 'NONE',  ( 9.117519353207999444, -4.954907757874000396, 8.825780921426000347 ) ) ;
#28522=CARTESIAN_POINT ( 'NONE',  ( 11.07127482541000063, -5.550092857035999749, 5.077717152805000467 ) ) ;
#28528=CARTESIAN_POINT ( 'NONE',  ( 11.09999999999999964, -5.299999999999999822, 6.469505845987999493 ) ) ;
#28531=CARTESIAN_POINT ( 'NONE',  ( 8.802620559624999785, -3.975070057433999438, 9.483761758588999058 ) ) ;
#28544=CARTESIAN_POINT ( 'NONE',  ( 11.07928355765999839, -7.977355694624001181, -6.935622273774999513 ) ) ;
#28545=EDGE_CURVE ( 'NONE', #22085, #65709, #68267, .T. ) ;
#28548=ORIENTED_EDGE ( 'NONE', *, *, #36095, .T. ) ;
#28551=CARTESIAN_POINT ( 'NONE',  ( 8.559591719171793400, -3.670668999121442955, 5.791868630734976264 ) ) ;
#28554=ORIENTED_EDGE ( 'NONE', *, *, #46050, .T. ) ;
#28555=DIRECTION ( 'NONE',  ( 0.000000000000000000, 1.000000000000000000, 0.000000000000000000 ) ) ;
#28557=CARTESIAN_POINT ( 'NONE',  ( 9.493541411000029129, -4.876956592064014551, 8.526784707585971290 ) ) ;
#28561=CARTESIAN_POINT ( 'NONE',  ( 10.48692887490000025, -8.228405771565000748, 6.845561203178999854 ) ) ;
#28564=LINE ( 'NONE', #54774, #66629 ) ;
#28572=VERTEX_POINT ( 'NONE', #25689 ) ;
#28573=CARTESIAN_POINT ( 'NONE',  ( 10.08712270112374121, -5.286531262339795312, -7.026829543710682024 ) ) ;
#28575=CARTESIAN_POINT ( 'NONE',  ( 10.95950272614480880, -2.825896501487262569, -6.683764319341896964 ) ) ;
#28577=CARTESIAN_POINT ( 'NONE',  ( 11.09999999999999964, -4.000000000000000000, 7.500000000000000000 ) ) ;
#28582=EDGE_CURVE ( 'NONE', #25195, #26111, #36525, .T. ) ;
#28591=CARTESIAN_POINT ( 'NONE',  ( 10.05525937050999907, -5.223866772223000332, -6.898311956607000361 ) ) ;
#28611=CARTESIAN_POINT ( 'NONE',  ( 8.014941940377999785, -2.280579276705999803, 6.510290672242000198 ) ) ;
#28612=CARTESIAN_POINT ( 'NONE',  ( 10.10633213213999859, -4.301175052434000001, -8.935144319903001175 ) ) ;
#28628=CARTESIAN_POINT ( 'NONE',  ( 9.298040139821001304, -4.087076480742000584, 9.429402848390999736 ) ) ;
#28632=B_SPLINE_CURVE_WITH_KNOTS ( 'NONE', 3,
 ( #26850, #11100, #28573, #2680 ),
 .UNSPECIFIED., .F., .F.,
 ( 4, 4 ),
 ( 0.8745849735171273842, 1.000000000000000000 ),
 .UNSPECIFIED. ) ;
#28633=CARTESIAN_POINT ( 'NONE',  ( 11.22022944037999892, -3.883088694641999794, -8.854817792072001481 ) ) ;
#28634=CARTESIAN_POINT ( 'NONE',  ( 7.933152249316766103, -2.298782909427148358, 7.863666461026288523 ) ) ;
#28635=CARTESIAN_POINT ( 'NONE',  ( 10.71756905878999966, -3.040221764047000175, 8.808455607108001573 ) ) ;
#28645=ORIENTED_EDGE ( 'NONE', *, *, #29687, .T. ) ;
#28648=DIRECTION ( 'NONE',  ( -1.000000000000000000, 0.000000000000000000, 0.000000000000000000 ) ) ;
#28654=CARTESIAN_POINT ( 'NONE',  ( 7.416894353206999746, -3.448181789123000218, 9.222458996124998976 ) ) ;
#28662=CARTESIAN_POINT ( 'NONE',  ( 8.027701659444524296, -5.080332885338415316, 8.330387188616123595 ) ) ;
#28688=B_SPLINE_CURVE_WITH_KNOTS ( 'NONE', 3,
 ( #56064, #23218, #17981, #49433 ),
 .UNSPECIFIED., .F., .F.,
 ( 4, 4 ),
 ( 0.000000000000000000, 1.000000000000000000 ),
 .UNSPECIFIED. ) ;
#28699=CARTESIAN_POINT ( 'NONE',  ( 8.625066940379999991, -3.117370956513999758, 8.662188901935000018 ) ) ;
#28715=DIRECTION ( 'NONE',  ( -1.000000000000000000, -3.552713678732000035E-14, 3.552713678732000035E-14 ) ) ;
#28726=EDGE_CURVE ( 'NONE', #10649, #20272, #22607, .T. ) ;
#28727=EDGE_CURVE ( 'NONE', #68990, #53568, #34930, .T. ) ;
#28728=CARTESIAN_POINT ( 'NONE',  ( 8.640591541102308426, -5.000946319700332765, 6.106569738443371698 ) ) ;
#28729=CARTESIAN_POINT ( 'NONE',  ( 9.392900668365001593, -2.713627063504739478, -7.026974105800378290 ) ) ;
#28731=CARTESIAN_POINT ( 'NONE',  ( 10.98956486188273551, -6.636233809049309151, 5.388476118166376061 ) ) ;
#28745=LINE ( 'NONE', #50061, #57695 ) ;
#28749=CIRCLE ( 'NONE', #35422, 1.350000000000000533 ) ;
#28750=CARTESIAN_POINT ( 'NONE',  ( 11.10061802256000085, -3.093055606601000207, -6.153681532251999542 ) ) ;
#28756=CARTESIAN_POINT ( 'NONE',  ( 11.04677151279999947, -2.764386413791999786, -5.039776830043000366 ) ) ;
#28760=CARTESIAN_POINT ( 'NONE',  ( 10.33385424252000107, -4.803082529331999417, 5.018848833410999966 ) ) ;
#28764=CARTESIAN_POINT ( 'NONE',  ( 10.89228096335999929, -3.998355205482000851, 9.261304730013998565 ) ) ;
#28770=CARTESIAN_POINT ( 'NONE',  ( 10.67500447327561908, -2.650284540010996004, 7.500001951671615430 ) ) ;
#28772=DIRECTION ( 'NONE',  ( 0.000000000000000000, 0.8648648648648720183, 0.5020047465136825426 ) ) ;
#28783=CARTESIAN_POINT ( 'NONE',  ( 9.480151033051999576, -4.233164088428999605, -6.141918726850000176 ) ) ;
#28789=CARTESIAN_POINT ( 'NONE',  ( 10.42441090035999984, -2.988250767850000322, 4.759068290708999172 ) ) ;
#28794=CARTESIAN_POINT ( 'NONE',  ( 9.877259503622999759, -2.207992199716000137, 7.624813542847999059 ) ) ;
#28799=CARTESIAN_POINT ( 'NONE',  ( 9.910792656537999790, -3.869344906782000049, 5.882544796414999944 ) ) ;
#28803=ORIENTED_EDGE ( 'NONE', *, *, #40122, .F. ) ;
#28810=EDGE_CURVE ( 'NONE', #55718, #62373, #8690, .T. ) ;
#28813=CARTESIAN_POINT ( 'NONE',  ( 9.482733921870000415, -2.757678812098000254, -6.584768124342000206 ) ) ;
#28814=CARTESIAN_POINT ( 'NONE',  ( 9.725191424783300675, -2.649754699899359522, 7.500009801425228773 ) ) ;
#28836=CARTESIAN_POINT ( 'NONE',  ( 11.04166666666869467, -2.793604566011342882, 8.411630010703568416 ) ) ;
#28837=ORIENTED_EDGE ( 'NONE', *, *, #51525, .T. ) ;
#28854=CARTESIAN_POINT ( 'NONE',  ( 7.682876674207999912, -9.044797463044000452, -5.468325094282000087 ) ) ;
#28855=VERTEX_POINT ( 'NONE', #8160 ) ;
#28860=VECTOR ( 'NONE', #21439, 1000.000000000000000 ) ;
#28862=CARTESIAN_POINT ( 'NONE',  ( 9.657547180956999711, -5.333447643521000536, 6.049925825719999928 ) ) ;
#28867=ORIENTED_EDGE ( 'NONE', *, *, #30253, .F. ) ;
#28872=CARTESIAN_POINT ( 'NONE',  ( 8.924956853209002006, -4.158911960977000000, 5.873536005760000123 ) ) ;
#28875=CARTESIAN_POINT ( 'NONE',  ( 10.96239535880000027, -5.423117484767999485, 4.905496954963999734 ) ) ;
#28876=CARTESIAN_POINT ( 'NONE',  ( 11.04384236319999957, -5.374509385214000012, 5.035088906224999938 ) ) ;
#28877=VERTEX_POINT ( 'NONE', #29506 ) ;
#28880=FACE_OUTER_BOUND ( 'NONE', #67165, .T. ) ;
#28881=CARTESIAN_POINT ( 'NONE',  ( 10.90145123840999908, -5.099999999122000638, 5.151026147719999670 ) ) ;
#28886=CARTESIAN_POINT ( 'NONE',  ( 7.775620559622000272, -4.636725880537000855, 9.378965771357000492 ) ) ;
#28887=DIRECTION ( 'NONE',  ( -0.7071067751363951936, 0.7071067872366950668, -8.276005153174941152E-08 ) ) ;
#28899=CARTESIAN_POINT ( 'NONE',  ( 10.90437356726000040, -2.900476673752999890, 5.132566153004000320 ) ) ;
#28902=VERTEX_POINT ( 'NONE', #28814 ) ;
#28907=CARTESIAN_POINT ( 'NONE',  ( 8.563725384270323815, -3.755834718894938806, 5.775588430088804515 ) ) ;
#28914=CARTESIAN_POINT ( 'NONE',  ( 9.490131905446967053, -4.919265557633711872, 8.488500456889612522 ) ) ;
#28929=ORIENTED_EDGE ( 'NONE', *, *, #42473, .F. ) ;
#28945=CARTESIAN_POINT ( 'NONE',  ( 10.17310292480999934, -4.709171320598000143, -8.664883863910000983 ) ) ;
#28948=LINE ( 'NONE', #55498, #43961 ) ;
#28949=CARTESIAN_POINT ( 'NONE',  ( 10.45746213570999927, -5.100000000000000533, -6.571291218949999902 ) ) ;
#28951=EDGE_CURVE ( 'NONE', #34621, #49491, #52521, .T. ) ;
#28955=CARTESIAN_POINT ( 'NONE',  ( 10.71922080291932033, -4.353435520373503564, -8.814860677227310148 ) ) ;
#28966=CARTESIAN_POINT ( 'NONE',  ( 8.849379440379999906, -3.975070057433999438, 9.483761758588999058 ) ) ;
#28976=ADVANCED_FACE ( 'NONE', ( #30863 ), #30151, .F. ) ;
#28980=CARTESIAN_POINT ( 'NONE',  ( 10.11260824411999870, -3.359889198679999911, 5.859131457670000209 ) ) ;
#28985=EDGE_CURVE ( 'NONE', #52849, #51171, #62796, .T. ) ;
#28986=CARTESIAN_POINT ( 'NONE',  ( 10.53870444038000009, -5.103398787993000063, -6.705198626796000205 ) ) ;
#28987=CARTESIAN_POINT ( 'NONE',  ( 7.966450313383576010, -2.301798426562205790, 7.124576740443179901 ) ) ;
#28988=CARTESIAN_POINT ( 'NONE',  ( 10.90374822854000136, -3.726845778959999578, 5.900452123196999743 ) ) ;
#28997=CARTESIAN_POINT ( 'NONE',  ( 9.311718600414000235, -4.588307032459999490, -5.987050435448999508 ) ) ;
#29000=FACE_OUTER_BOUND ( 'NONE', #18665, .T. ) ;
#29006=AXIS2_PLACEMENT_3D ( 'NONE', #12019, #38237, #7121 ) ;
#29009=CARTESIAN_POINT ( 'NONE',  ( 8.957394353210000659, -2.678334737187000325, 8.735278777293000729 ) ) ;
#29015=CARTESIAN_POINT ( 'NONE',  ( 10.22908305962000064, -4.838492992840000007, -5.852445959518000507 ) ) ;
#29023=VERTEX_POINT ( 'NONE', #55290 ) ;
#29025=CARTESIAN_POINT ( 'NONE',  ( 27.64127793187000037, -2.399999999999999911, -6.571291218949999902 ) ) ;
#29029=CARTESIAN_POINT ( 'NONE',  ( 11.09999999999999964, -4.000000000000000000, -9.049999999995968381 ) ) ;
#29043=DIRECTION ( 'NONE',  ( 1.000000000000000000, 0.000000000000000000, 0.000000000000000000 ) ) ;
#29047=CARTESIAN_POINT ( 'NONE',  ( 10.80231684603725917, -4.484370860713429607, 9.173854975331316552 ) ) ;
#29061=CARTESIAN_POINT ( 'NONE',  ( 9.817462135711998883, -5.100000000000000533, 6.571291218949999902 ) ) ;
#29062=CARTESIAN_POINT ( 'NONE',  ( 9.383148997457999130, -5.167567567567999731, 6.822293592207000934 ) ) ;
#29067=EDGE_CURVE ( 'NONE', #68446, #66560, #60455, .T. ) ;
#29070=CARTESIAN_POINT ( 'NONE',  ( 7.688565988106098814, -2.650624002730362250, 7.262809006051590188 ) ) ;
#29074=CARTESIAN_POINT ( 'NONE',  ( 10.83824331590383672, -5.765061639177475605, -7.465997195058596603 ) ) ;
#29078=CARTESIAN_POINT ( 'NONE',  ( 10.65229194037999960, -4.944342461481999962, -8.478476072358999360 ) ) ;
#29087=EDGE_LOOP ( 'NONE', ( #30219, #40632, #40983, #34749 ) ) ;
#29098=CARTESIAN_POINT ( 'NONE',  ( 10.52342417510000061, -3.209670667763000029, -9.177087527572998837 ) ) ;
#29110=CARTESIAN_POINT ( 'NONE',  ( 9.667080975990000269, -4.541622198376999542, 5.824041840233000755 ) ) ;
#29125=CARTESIAN_POINT ( 'NONE',  ( 9.612156140204000110, -5.332339947063000629, -7.851654145788001138 ) ) ;
#29131=CARTESIAN_POINT ( 'NONE',  ( 10.33390208397999999, -3.197011589206999904, 5.018836569371999623 ) ) ;
#29134=AXIS2_PLACEMENT_3D ( 'NONE', #2439, #29373, #50687 ) ;
#29136=CARTESIAN_POINT ( 'NONE',  ( 10.84168850528999961, -2.681008214828000114, 6.554752254946000889 ) ) ;
#29140=CARTESIAN_POINT ( 'NONE',  ( 9.352255147285999826, -2.817754448466000206, 6.388456890282999900 ) ) ;
#29141=DIRECTION ( 'NONE',  ( 0.000000000000000000, 1.000000000000000000, 0.000000000000000000 ) ) ;
#29153=CARTESIAN_POINT ( 'NONE',  ( 9.309310001151999359, -5.531435376468999188, -8.256621485025000595 ) ) ;
#29164=CARTESIAN_POINT ( 'NONE',  ( 9.354620317202259727, -2.650257996360415369, -7.676659957281179558 ) ) ;
#29167=EDGE_CURVE ( 'NONE', #25033, #42399, #20287, .T. ) ;
#29175=CARTESIAN_POINT ( 'NONE',  ( 11.03333333333535293, -2.969278270712975676, 8.594189652917078703 ) ) ;
#29177=CARTESIAN_POINT ( 'NONE',  ( 8.679055905797000037, -2.899999999999999911, 6.571291218949999902 ) ) ;
#29181=CARTESIAN_POINT ( 'NONE',  ( 11.02938691836999929, -8.053295335382999909, 6.898627764883999980 ) ) ;
#29182=ORIENTED_EDGE ( 'NONE', *, *, #63198, .T. ) ;
#29190=CARTESIAN_POINT ( 'NONE',  ( 9.382598168139042016, -2.846997224034427898, 8.802713852305345199 ) ) ;
#29191=ORIENTED_EDGE ( 'NONE', *, *, #66488, .T. ) ;
#29197=CARTESIAN_POINT ( 'NONE',  ( 9.034116535116000435, -4.695350938297000454, 8.660677768253002284 ) ) ;
#29208=CARTESIAN_POINT ( 'NONE',  ( 9.292149251564818968, -4.685486125476070463, 9.106491892308623548 ) ) ;
#29222=CARTESIAN_POINT ( 'NONE',  ( 11.13226790813000022, -5.329954231730000380, 5.054493266885999425 ) ) ;
#29225=EDGE_CURVE ( 'NONE', #29433, #10252, #22045, .T. ) ;
#29228=CARTESIAN_POINT ( 'NONE',  ( 8.361422056298998484, -5.126342729456004221, 6.365321850284000327 ) ) ;
#29236=AXIS2_PLACEMENT_3D ( 'NONE', #59824, #11572, #16820 ) ;
#29244=CARTESIAN_POINT ( 'NONE',  ( 8.576404413402933358, -4.033774881259239997, 5.760694017649135468 ) ) ;
#29253=CARTESIAN_POINT ( 'NONE',  ( 7.533879440377999614, -4.623636604834999275, 8.651469651195000665 ) ) ;
#29255=ORIENTED_EDGE ( 'NONE', *, *, #39228, .T. ) ;
#29282=CARTESIAN_POINT ( 'NONE',  ( 10.13061232742999884, -2.189322372303999842, -7.101642112140999608 ) ) ;
#29284=CARTESIAN_POINT ( 'NONE',  ( 9.042738649950948115, -4.892150455714567414, 8.513356723856825070 ) ) ;
#29286=ADVANCED_FACE ( 'NONE', ( #20197 ), #51668, .T. ) ;
#29287=ORIENTED_EDGE ( 'NONE', *, *, #27056, .T. ) ;
#29292=DIRECTION ( 'NONE',  ( 0.000000000000000000, -0.1333333333333049930, -0.9910712498212376209 ) ) ;
#29305=CARTESIAN_POINT ( 'NONE',  ( 9.170316940378999249, -5.558929022707999046, 6.272984818914999927 ) ) ;
#29318=CARTESIAN_POINT ( 'NONE',  ( 9.444317341922999987, -2.927260449021000355, 8.897015448164999896 ) ) ;
#29320=VERTEX_POINT ( 'NONE', #68423 ) ;
#29324=CARTESIAN_POINT ( 'NONE',  ( 7.948545716009685513, -2.259334748069345977, 7.519046407094909235 ) ) ;
#29325=CARTESIAN_POINT ( 'NONE',  ( 9.137549407199999862, -2.995696424181999884, 8.544763501938000161 ) ) ;
#29328=ORIENTED_EDGE ( 'NONE', *, *, #45625, .F. ) ;
#29333=EDGE_CURVE ( 'NONE', #65921, #17154, #62496, .T. ) ;
#29336=CARTESIAN_POINT ( 'NONE',  ( 9.575728814717999526, -3.111669560323000017, -8.958991988670002016 ) ) ;
#29344=ORIENTED_EDGE ( 'NONE', *, *, #39476, .T. ) ;
#29348=CARTESIAN_POINT ( 'NONE',  ( 7.866206853207000194, -4.580607464247000493, 9.213361409141999303 ) ) ;
#29363=ORIENTED_EDGE ( 'NONE', *, *, #61088, .F. ) ;
#29366=DIRECTION ( 'NONE',  ( -1.000000000000000000, 5.329070518330000258E-14, -1.243449787610000074E-13 ) ) ;
#29372=EDGE_CURVE ( 'NONE', #50410, #9350, #43907, .T. ) ;
#29373=DIRECTION ( 'NONE',  ( -1.000000000000000000, 0.000000000000000000, 0.000000000000000000 ) ) ;
#29374=EDGE_CURVE ( 'NONE', #31101, #50410, #31388, .T. ) ;
#29375=EDGE_CURVE ( 'NONE', #25798, #21322, #4590, .T. ) ;
#29395=CARTESIAN_POINT ( 'NONE',  ( 7.571668146791999732, -2.531197775378000170, 8.216705951490000714 ) ) ;
#29412=CARTESIAN_POINT ( 'NONE',  ( 8.245293146793999384, -4.282999948634999221, 9.286791354293999490 ) ) ;
#29416=CARTESIAN_POINT ( 'NONE',  ( 7.433354534967393512, -2.295543244304647512, 7.846514096336020927 ) ) ;
#29421=CARTESIAN_POINT ( 'NONE',  ( 10.98973493139468793, -3.461032840053388515, -9.181186645308331506 ) ) ;
#29433=VERTEX_POINT ( 'NONE', #15644 ) ;
#29441=CARTESIAN_POINT ( 'NONE',  ( 10.47706399772000019, -8.232249776294999322, 6.630938099616999537 ) ) ;
#29445=CARTESIAN_POINT ( 'NONE',  ( 9.869049086607999399, -5.575175898444999945, 7.724300702620999104 ) ) ;
#29447=CARTESIAN_POINT ( 'NONE',  ( 10.01276877312999858, -3.440626575163999945, -9.267592337498999910 ) ) ;
#29449=CARTESIAN_POINT ( 'NONE',  ( 10.64946917938723558, -2.962827107629537604, -5.047145064087899868 ) ) ;
#29459=CARTESIAN_POINT ( 'NONE',  ( 9.778462793022999477, -5.743713977826000239, 7.748300060190000060 ) ) ;
#29481=EDGE_CURVE ( 'NONE', #17007, #2520, #2867, .T. ) ;
#29488=MANIFOLD_SOLID_BREP ( 'Stock-MAS-678-1', #3474 ) ;
#29491=CARTESIAN_POINT ( 'NONE',  ( 10.74609562913000005, -4.263104965433000437, 9.276976808608999647 ) ) ;
#29501=CARTESIAN_POINT ( 'NONE',  ( 11.04839869688000142, -2.759396991474999616, 5.061364986604000471 ) ) ;
#29505=CARTESIAN_POINT ( 'NONE',  ( 9.927916723342999461, -5.290169207169999943, -8.858081286661999343 ) ) ;
#29506=CARTESIAN_POINT ( 'NONE',  ( 8.433148997460000018, -5.167567567567999731, 6.822293592207000934 ) ) ;
#29507=EDGE_CURVE ( 'NONE', #61617, #25033, #43734, .T. ) ;
#29508=VERTEX_POINT ( 'NONE', #21569 ) ;
#29509=CARTESIAN_POINT ( 'NONE',  ( 11.09999999999999964, -5.449702613288000208, -5.124965750789000296 ) ) ;
#29513=CARTESIAN_POINT ( 'NONE',  ( 10.05091168077847108, -5.349831496875363968, -7.263252183692045172 ) ) ;
#29520=CARTESIAN_POINT ( 'NONE',  ( 9.292123497980924185, -3.170553882200173756, -8.579481765757963174 ) ) ;
#29528=CARTESIAN_POINT ( 'NONE',  ( 9.316292271078561171, -5.056976493916715221, -6.220632899828596685 ) ) ;
#29546=CARTESIAN_POINT ( 'NONE',  ( 9.382540076676905372, -2.847952239995268808, 8.803561693506937402 ) ) ;
#29551=CARTESIAN_POINT ( 'NONE',  ( 9.933148997456999751, -5.167567567567999731, 6.822293592207000934 ) ) ;
#29554=CARTESIAN_POINT ( 'NONE',  ( 10.18755811987000115, -5.387486580809999204, 8.640943191857999750 ) ) ;
#29557=VERTEX_POINT ( 'NONE', #949 ) ;
#29567=CARTESIAN_POINT ( 'NONE',  ( 11.01665874711000015, -5.432796194138000523, 4.991871746747999161 ) ) ;
#29568=CARTESIAN_POINT ( 'NONE',  ( 8.226385565605996320, -4.797071061338999520, -6.615828105123995329 ) ) ;
#29572=CARTESIAN_POINT ( 'NONE',  ( 10.92160119059999879, -2.751730582352999832, -4.977179449700000369 ) ) ;
#29578=LINE ( 'NONE', #61026, #49668 ) ;
#29599=CARTESIAN_POINT ( 'NONE',  ( 9.500008250440000523, -2.279684233303000074, 7.877691491255999878 ) ) ;
#29601=CARTESIAN_POINT ( 'NONE',  ( 9.905375278050065901, -5.100000000000000533, -6.445686799065932782 ) ) ;
#29602=CARTESIAN_POINT ( 'NONE',  ( 7.662254440376999653, -2.688354259407999880, 8.140021027181001401 ) ) ;
#29608=CARTESIAN_POINT ( 'NONE',  ( 8.878359312501501677, -5.126777126186120803, 6.752018918873290865 ) ) ;
#29618=EDGE_LOOP ( 'NONE', ( #42313, #57527, #65404, #25971, #25683 ) ) ;
#29619=CARTESIAN_POINT ( 'NONE',  ( 11.09999999999999964, -5.299999999999999822, 5.160242713806000303 ) ) ;
#29623=CARTESIAN_POINT ( 'NONE',  ( 7.903235257726999308, -5.126111038912999796, 6.730858764360999835 ) ) ;
#29626=EDGE_LOOP ( 'NONE', ( #46694, #11889, #20875, #51997 ) ) ;
#29627=ADVANCED_FACE ( 'NONE', ( #38697 ), #44986, .F. ) ;
#29629=ADVANCED_FACE ( 'NONE', ( #66639 ), #67287, .T. ) ;
#29636=CARTESIAN_POINT ( 'NONE',  ( 10.44486180556999955, -4.964082081645000422, -9.083599939499999110 ) ) ;
#29643=CARTESIAN_POINT ( 'NONE',  ( 10.65673534980114923, -5.179482957637668861, -8.179835726794200568 ) ) ;
#29644=CARTESIAN_POINT ( 'NONE',  ( 7.950754440378000609, -2.095727472214000020, 8.056487497515000484 ) ) ;
#29657=CARTESIAN_POINT ( 'NONE',  ( 7.229683059621999419, -2.630475685621000093, 6.995953627589999613 ) ) ;
#29671=CARTESIAN_POINT ( 'NONE',  ( 9.351499161061999743, -4.821938821912000073, 8.950150764319998231 ) ) ;
#29675=CARTESIAN_POINT ( 'NONE',  ( 10.50084194037999907, -4.616788958496999662, -6.288071994190999270 ) ) ;
#29676=CARTESIAN_POINT ( 'NONE',  ( 7.925145711943240023, -2.342924674265735696, 8.034557503593903860 ) ) ;
#29678=CARTESIAN_POINT ( 'NONE',  ( 9.724613486786999772, -2.928302463146000179, 8.718481221599999387 ) ) ;
#29687=EDGE_CURVE ( 'NONE', #7601, #65525, #19456, .T. ) ;
#29696=VERTEX_POINT ( 'NONE', #2668 ) ;
#29699=CARTESIAN_POINT ( 'NONE',  ( 8.085168146793000332, -2.431397064767999439, 7.958394431095000776 ) ) ;
#29701=ORIENTED_EDGE ( 'NONE', *, *, #25874, .F. ) ;
#29703=VECTOR ( 'NONE', #29792, 1000.000000000000000 ) ;
#29705=CARTESIAN_POINT ( 'NONE',  ( 10.50898185320999900, -4.485028460808000439, -9.114431591966999591 ) ) ;
#29708=CARTESIAN_POINT ( 'NONE',  ( 7.325000000000000178, -4.000000000000000000, 9.239711431703000244 ) ) ;
#29716=CARTESIAN_POINT ( 'NONE',  ( 8.435453087375249126, -3.606524746037642615, 6.005799303653357235 ) ) ;
#29742=CARTESIAN_POINT ( 'NONE',  ( 8.047379440378000126, -4.468370631666999770, 8.882152684713000568 ) ) ;
#29743=CARTESIAN_POINT ( 'NONE',  ( 11.04384236319999957, -7.396937235950000300, -6.274987567768999241 ) ) ;
#29756=CARTESIAN_POINT ( 'NONE',  ( 7.950754440378000609, -2.095727472214000020, 8.056487497515000484 ) ) ;
#29761=CARTESIAN_POINT ( 'NONE',  ( 10.68360729283869581, -2.821290678668196161, 8.178873955024902997 ) ) ;
#29771=CARTESIAN_POINT ( 'NONE',  ( 9.674960421382822418, -2.650268802167429438, 7.499999178247414910 ) ) ;
#29772=CARTESIAN_POINT ( 'NONE',  ( 9.378950334184001036, -2.649999999999999911, -7.263338156157796988 ) ) ;
#29782=CARTESIAN_POINT ( 'NONE',  ( 10.26537527815838580, -5.100000000000000533, 6.445686799303629755 ) ) ;
#29792=DIRECTION ( 'NONE',  ( -1.000000000000000000, 2.350993083155999923E-10, 3.098106116599000021E-09 ) ) ;
#29799=FACE_OUTER_BOUND ( 'NONE', #32413, .T. ) ;
#29805=CARTESIAN_POINT ( 'NONE',  ( 10.83659005484000026, -5.133183563847000030, 8.848364935581999546 ) ) ;
#29815=CARTESIAN_POINT ( 'NONE',  ( 8.928197172114431979, -5.125396288428769154, 6.749639981086935414 ) ) ;
#29832=CARTESIAN_POINT ( 'NONE',  ( 10.09697182628999990, -5.253379538902000156, 8.530665717066000298 ) ) ;
#29834=CARTESIAN_POINT ( 'NONE',  ( 10.91620964606000044, -2.818413279081999789, -6.814156272943999504 ) ) ;
#29839=VERTEX_POINT ( 'NONE', #40412 ) ;
#29845=CARTESIAN_POINT ( 'NONE',  ( 9.041568618727998441, -2.868050178059002420, -6.343697345132999210 ) ) ;
#29848=CARTESIAN_POINT ( 'NONE',  ( 9.661323620223001285, -4.289037785427000316, -5.816478295321999781 ) ) ;
#29850=ORIENTED_EDGE ( 'NONE', *, *, #34124, .F. ) ;
#29887=DIRECTION ( 'NONE',  ( 0.000000000000000000, -1.000000000000000000, 0.000000000000000000 ) ) ;
#29888=ORIENTED_EDGE ( 'NONE', *, *, #64295, .T. ) ;
#29892=CONICAL_SURFACE ( 'NONE', #49986, 0.8999999994071996579, 0.7853981633972997312 ) ;
#29911=CARTESIAN_POINT ( 'NONE',  ( 8.486008579191000933, -3.399999999999999911, 5.976611076844000614 ) ) ;
#29912=CARTESIAN_POINT ( 'NONE',  ( 10.60232725808000076, -2.940669124847000049, -4.956116633172999997 ) ) ;
#29913=CARTESIAN_POINT ( 'NONE',  ( 9.487725409950000355, -4.905858243509999106, -8.948175900338000588 ) ) ;
#29927=CARTESIAN_POINT ( 'NONE',  ( 7.773264358664000007, -2.859518314699000197, 6.768377407145999669 ) ) ;
#29928=DIRECTION ( 'NONE',  ( -1.000000000000000000, 0.000000000000000000, 0.000000000000000000 ) ) ;
#29938=CARTESIAN_POINT ( 'NONE',  ( 9.580795537697266440, -5.100000000000000533, -6.662590550601107608 ) ) ;
#29943=CARTESIAN_POINT ( 'NONE',  ( 11.24052627608000066, -2.774025043188999895, 6.782107572692000375 ) ) ;
#29945=CARTESIAN_POINT ( 'NONE',  ( 8.476294715524065992, -3.031386904610626765, 6.154469090921128149 ) ) ;
#29946=CARTESIAN_POINT ( 'NONE',  ( 7.635855646791999796, -2.466384407480000096, 6.935560677555000275 ) ) ;
#29950=CARTESIAN_POINT ( 'NONE',  ( 11.02214804248387203, -5.404890988668177521, -8.010352125886161190 ) ) ;
#29954=ORIENTED_EDGE ( 'NONE', *, *, #61529, .F. ) ;
#29955=CARTESIAN_POINT ( 'NONE',  ( 8.716851002545999094, -2.832432432432000269, 6.822293592207000934 ) ) ;
#29960=CARTESIAN_POINT ( 'NONE',  ( 5.699999999554000496, -0.3000000004460000036, 9.662944681662999358 ) ) ;
#29965=CARTESIAN_POINT ( 'NONE',  ( 10.94975213449457208, -2.829972217754548325, -6.705091429376293100 ) ) ;
#29967=DIRECTION ( 'NONE',  ( -1.000000000000000000, 0.000000000000000000, 0.000000000000000000 ) ) ;
#29974=B_SPLINE_CURVE_WITH_KNOTS ( 'NONE', 3,
 ( #58749, #30816, #10855, #47927, #26, #16101, #58072, #37091, #26949, #32201, #52129, #52825, #26258, #4231 ),
 .UNSPECIFIED., .F., .F.,
 ( 4, 2, 1, 1, 2, 2, 2, 4 ),
 ( 0.8006037889120940498, 0.8504528416840665406, 0.8629151048770596910, 0.8691462364735562662, 0.8722618022718046094, 0.8753773680700528415, 0.9003018944560425840, 1.000000000000000000 ),
 .UNSPECIFIED. ) ;
#29978=CARTESIAN_POINT ( 'NONE',  ( 10.16989351219999982, -2.594225604561000154, -6.291264536816999708 ) ) ;
#29980=CARTESIAN_POINT ( 'NONE',  ( 9.039567739507649691, -4.932484926559381755, 8.476014846726219076 ) ) ;
#29999=CARTESIAN_POINT ( 'NONE',  ( 7.422245559621999611, -5.361050935357000391, 6.973449182446000094 ) ) ;
#30016=CYLINDRICAL_SURFACE ( 'NONE', #17650, 2.000000000000000444 ) ;
#30017=EDGE_CURVE ( 'NONE', #64705, #35912, #36543, .T. ) ;
#30018=EDGE_CURVE ( 'NONE', #46752, #52724, #17857, .T. ) ;
#30019=CARTESIAN_POINT ( 'NONE',  ( 10.17270027370999941, -4.650151116117000605, -8.655526539784000661 ) ) ;
#30020=CARTESIAN_POINT ( 'NONE',  ( 8.127894995188555072, -5.076156598471832204, 6.133170389101868736 ) ) ;
#30028=VECTOR ( 'NONE', #55499, 1000.000000000000000 ) ;
#30030=CARTESIAN_POINT ( 'NONE',  ( 9.910492310842998975, -4.686746084135999801, -9.174865097765998456 ) ) ;
#30039=CARTESIAN_POINT ( 'NONE',  ( 8.727043146794999373, -3.882020254083999866, 5.870054788755000530 ) ) ;
#30045=CARTESIAN_POINT ( 'NONE',  ( 10.54684435321000002, -3.691674321452999674, -9.157280075569998345 ) ) ;
#30050=SHAPE_REPRESENTATION ( 'Positive Post', ( #9676 ), #16178 ) ;
#30054=ORIENTED_EDGE ( 'NONE', *, *, #38801, .T. ) ;
#30056=CARTESIAN_POINT ( 'NONE',  ( 10.27194008929999924, -4.567480829194999536, 4.846795848580000232 ) ) ;
#30065=EDGE_LOOP ( 'NONE', ( #41797, #43243, #9234, #4169, #26567 ) ) ;
#30079=ORIENTED_EDGE ( 'NONE', *, *, #2489, .T. ) ;
#30083=CARTESIAN_POINT ( 'NONE',  ( 7.854816940377000734, -4.561648098548999997, 6.153050355516999304 ) ) ;
#30091=CARTESIAN_POINT ( 'NONE',  ( 9.564964385875493136, -5.350010280223940207, -7.500002129152480101 ) ) ;
#30097=CARTESIAN_POINT ( 'NONE',  ( 7.501441940376999185, -2.138201851198999748, 6.814774777484000623 ) ) ;
#30102=CARTESIAN_POINT ( 'NONE',  ( 7.325000000000000178, -4.000000000000000000, 9.239711431703000244 ) ) ;
#30109=CARTESIAN_POINT ( 'NONE',  ( 10.64360935987385659, -5.049157587798284830, 5.054580113003310338 ) ) ;
#30112=CARTESIAN_POINT ( 'NONE',  ( 11.18236694037999968, -4.516641106826999597, -8.757887038823000125 ) ) ;
#30130=FACE_OUTER_BOUND ( 'NONE', #26743, .T. ) ;
#30134=CARTESIAN_POINT ( 'NONE',  ( 10.90379229492000057, -5.099791907704999794, -5.134764377744000186 ) ) ;
#30137=DIRECTION ( 'NONE',  ( 1.000000000000000000, 0.000000000000000000, 0.000000000000000000 ) ) ;
#30151=B_SPLINE_SURFACE_WITH_KNOTS ( 'NONE', 3, 3, ( 
 ( #36444, #51832, #4971, #9872, #10217, #21056, #14782, #26654, #47632, #57079, #42385, #52178, #63344, #3927, #15470, #63691, #57417, #15806, #4278, #21390, #25265, #25613, #46941, #31898, #68244, #53210, #46604, #36796, #5312, #47971, #67908, #20025, #41351, #62662, #20365 ),
 ( #41689, #62995, #57761, #4620, #25954, #54593, #43421, #53891, #11579, #11936, #32923, #38867, #60187, #6335, #53557, #65057, #49693, #6689, #54235, #16148, #27685, #17178, #28032, #16490, #38507, #64716, #48656, #7042, #1110, #59481, #760, #64366, #22423, #49340, #21727 ),
 ( #43765, #48999, #59831, #33276, #1454, #22769, #5993, #28377, #1802, #5650, #59139, #11243, #42723, #44120, #65416, #32581, #38154, #17537, #48307, #12293, #58798, #22074, #33623, #16830, #27333, #54941, #64027, #37818, #37471, #10903, #32248, #26991, #414, #43062, #67141 ),
 ( #34315, #13679, #39207, #65764, #55638, #18230, #30112, #45829, #13341, #24508, #45493, #35008, #61225, #24158, #2488, #66457, #39553, #44471, #33967, #35348, #29078, #60877, #19252, #23813, #56323, #23118, #12992, #2830, #50734, #51076, #34664, #50389, #17889, #2153, #45148 ) ),
 .UNSPECIFIED., .F., .F., .F.,
 ( 4, 4 ),
 ( 4, 1, 1, 1, 1, 1, 1, 1, 1, 1, 1, 1, 1, 1, 1, 1, 1, 1, 1, 1, 1, 1, 1, 1, 1, 1, 1, 1, 1, 1, 1, 1, 4 ),
 ( -0.1039086239011999951, 1.103908623900999864 ),
 ( 0.2233333333344000027, 0.2480800653604999795, 0.2728267973865999840, 0.2975735294126999886, 0.3223202614387999931, 0.3470669934649999733, 0.3718137254910999778, 0.3965604575171999824, 0.4213071895433000424, 0.4460539215694000470, 0.4708006535954999960, 0.4955473856216000006, 0.5202941176476999496, 0.5450408496738000652, 0.5697875816999000698, 0.5945343137260000743, 0.6192810457521999989, 0.6440277777783000035, 0.6687745098044000081, 0.6935212418305000126, 0.7182679738566000172, 0.7430147058827000217, 0.7677614379088000263, 0.7925081699349000308, 0.8172549019609999243, 0.8420016339870999289, 0.8667483660132000445, 0.8914950980394000801, 0.9162418300655000847, 0.9409885620915999782, 0.9657352941176999828, 0.9904820261437999873, 1.015228758169999912 ),
 .UNSPECIFIED. ) ;
#30152=CARTESIAN_POINT ( 'NONE',  ( 10.23921655905610528, -2.650856495401338275, 7.263814070341720885 ) ) ;
#30157=CARTESIAN_POINT ( 'NONE',  ( 10.83253786428999987, -2.899999999999999911, 6.571291218949999902 ) ) ;
#30158=CARTESIAN_POINT ( 'NONE',  ( 19.01453011999999987, 0.8000000000000000444, 3.149999999999999911 ) ) ;
#30169=CARTESIAN_POINT ( 'NONE',  ( 10.71756905878999966, -3.040221764047000175, 8.808455607108001573 ) ) ;
#30172=CARTESIAN_POINT ( 'NONE',  ( 10.93728138146000006, -5.425439422033999648, 7.240583766112999697 ) ) ;
#30177=CARTESIAN_POINT ( 'NONE',  ( 10.67701940544685790, -5.048701884080403879, -5.056137651350367079 ) ) ;
#30183=CARTESIAN_POINT ( 'NONE',  ( 9.218723707566001124, -5.383415012847999392, -8.183490493635000362 ) ) ;
#30185=CARTESIAN_POINT ( 'NONE',  ( 9.704564187634451500, -2.648431596117190256, 7.852956029643703317 ) ) ;
#30188=CARTESIAN_POINT ( 'NONE',  ( 8.270987825454401587, -2.867662898289943918, 6.761597767506805745 ) ) ;
#30210=ORIENTED_EDGE ( 'NONE', *, *, #9823, .T. ) ;
#30212=ORIENTED_EDGE ( 'NONE', *, *, #28545, .T. ) ;
#30219=ORIENTED_EDGE ( 'NONE', *, *, #53147, .T. ) ;
#30227=CARTESIAN_POINT ( 'NONE',  ( 9.679055905794999859, -2.899999999999999911, 6.571291218949999902 ) ) ;
#30228=CARTESIAN_POINT ( 'NONE',  ( 10.68375832677999959, -4.547311397465000127, -8.749131152219000285 ) ) ;
#30230=VERTEX_POINT ( 'NONE', #57693 ) ;
#30243=CARTESIAN_POINT ( 'NONE',  ( 8.285673191594010945, -4.510969308813000289, -6.771077081157996780 ) ) ;
#30246=CARTESIAN_POINT ( 'NONE',  ( 27.64127793187000037, -2.399999999999999911, -6.571291218949999902 ) ) ;
#30248=CARTESIAN_POINT ( 'NONE',  ( 9.265134009212999899, -5.494586520014999920, -6.370782351137999733 ) ) ;
#30253=EDGE_CURVE ( 'NONE', #41719, #29839, #6065, .T. ) ;
#30254=CARTESIAN_POINT ( 'NONE',  ( 7.674540706797001732, -4.591334964886001124, 6.448517731106997886 ) ) ;
#30273=CARTESIAN_POINT ( 'NONE',  ( 11.07345355053000091, -3.998673159585000025, 8.920828114954002075 ) ) ;
#30278=CARTESIAN_POINT ( 'NONE',  ( 9.074379440379999551, -3.981661727120999750, 8.959239802162999311 ) ) ;
#30287=CARTESIAN_POINT ( 'NONE',  ( 8.172783018424818025, -2.939287716552612562, 6.492393787938203431 ) ) ;
#30289=CARTESIAN_POINT ( 'NONE',  ( 10.40226385995999969, -2.765692573780999641, 9.035345396600000356 ) ) ;
#30292=CARTESIAN_POINT ( 'NONE',  ( 10.80160188108999897, -2.805072368922999715, -8.157282064671999677 ) ) ;
#30302=CARTESIAN_POINT ( 'NONE',  ( 7.935252636294002571, -4.895109672515001620, 6.296391117214003685 ) ) ;
#30308=CARTESIAN_POINT ( 'NONE',  ( 8.767879976495999372, -3.394455611366999914, -6.293427637271999942 ) ) ;
#30330=CARTESIAN_POINT ( 'NONE',  ( 7.678995559621999867, -2.599231861044000169, 7.909347897884000389 ) ) ;
#30332=ADVANCED_FACE ( 'NONE', ( #59763 ), #45053, .T. ) ;
#30336=EDGE_CURVE ( 'NONE', #1683, #37807, #58707, .T. ) ;
#30343=CARTESIAN_POINT ( 'NONE',  ( 9.227780634805492710, -4.987352003971340153, -6.146612417831175179 ) ) ;
#30350=CARTESIAN_POINT ( 'NONE',  ( 8.122344632841924650, -4.980189395210384617, 6.061431015808207867 ) ) ;
#30353=ORIENTED_EDGE ( 'NONE', *, *, #3488, .F. ) ;
#30354=CARTESIAN_POINT ( 'NONE',  ( 10.37168190983000038, -4.576053486415999849, -5.010430378404000074 ) ) ;
#30359=CARTESIAN_POINT ( 'NONE',  ( 10.10891502095999961, -5.332339947063000629, -7.851654145788001138 ) ) ;
#30368=CARTESIAN_POINT ( 'NONE',  ( 7.903995559621998623, -2.095727472214000020, 8.056487497515000484 ) ) ;
#30374=CARTESIAN_POINT ( 'NONE',  ( 10.41025564679000048, -4.690690303276999984, -6.142863315966000215 ) ) ;
#30396=ORIENTED_EDGE ( 'NONE', *, *, #36095, .F. ) ;
#30407=CARTESIAN_POINT ( 'NONE',  ( 9.222206812071494397, -2.649920440492297136, 7.547755730313211231 ) ) ;
#30412=FACE_OUTER_BOUND ( 'NONE', #66209, .T. ) ;
#30419=EDGE_CURVE ( 'NONE', #14644, #67945, #28632, .T. ) ;
#30429=CARTESIAN_POINT ( 'NONE',  ( 7.924355646793000751, -2.432121990576000314, 6.597519606637999523 ) ) ;
#30433=CARTESIAN_POINT ( 'NONE',  ( 10.60770805961999841, -2.392337812398999564, -6.587351599745000286 ) ) ;
#30434=CARTESIAN_POINT ( 'NONE',  ( 7.634776897685090269, -5.200043634672757875, 6.239116708909331344 ) ) ;
#30443=CARTESIAN_POINT ( 'NONE',  ( 8.473304831784332691, -5.100000000000000533, 6.564173320837334735 ) ) ;
#30453=ORIENTED_EDGE ( 'NONE', *, *, #48802, .T. ) ;
#30460=CARTESIAN_POINT ( 'NONE',  ( 10.14750362918999826, -2.602959084636999876, 6.738575912023000214 ) ) ;
#30463=CARTESIAN_POINT ( 'NONE',  ( 9.934206403597999113, -5.120430559539999926, -8.883390070891001855 ) ) ;
#30478=EDGE_CURVE ( 'NONE', #40213, #8185, #14509, .T. ) ;
#30483=EDGE_CURVE ( 'NONE', #42097, #31041, #38648, .T. ) ;
#30488=DIRECTION ( 'NONE',  ( 0.000000000000000000, 0.000000000000000000, 1.000000000000000000 ) ) ;
#30497=EDGE_CURVE ( 'NONE', #65921, #6365, #27015, .T. ) ;
#30499=CYLINDRICAL_SURFACE ( 'NONE', #19551, 1.350000000000000089 ) ;
#30502=DIRECTION ( 'NONE',  ( 1.000000000000000000, 0.000000000000000000, 0.000000000000000000 ) ) ;
#30516=B_SPLINE_CURVE_WITH_KNOTS ( 'NONE', 3,
 ( #34332, #33638, #12305, #29441, #2168 ),
 .UNSPECIFIED., .F., .F.,
 ( 4, 1, 4 ),
 ( 0.000000000000000000, 0.6268453884324000080, 1.000000000000000000 ),
 .UNSPECIFIED. ) ;
#30518=CARTESIAN_POINT ( 'NONE',  ( 11.04862408378999916, -2.758083014511000020, -5.064624117739000120 ) ) ;
#30529=CARTESIAN_POINT ( 'NONE',  ( 8.674830025576039105, -2.649890579813208191, 7.499988935010342139 ) ) ;
#30546=ORIENTED_EDGE ( 'NONE', *, *, #57050, .T. ) ;
#30555=CARTESIAN_POINT ( 'NONE',  ( 8.091573680993423778, -3.319738643651890531, 8.680038712423783664 ) ) ;
#30573=CARTESIAN_POINT ( 'NONE',  ( 8.366396006187004630, -4.495298813396003013, -6.688382266309997881 ) ) ;
#30578=CARTESIAN_POINT ( 'NONE',  ( 11.09999999999999964, -6.350523631572000838, 5.385484235140999942 ) ) ;
#30579=CARTESIAN_POINT ( 'NONE',  ( 9.661149330668999724, -3.300107492866999781, -5.762405935562999737 ) ) ;
#30583=CARTESIAN_POINT ( 'NONE',  ( 11.13119666232000071, -5.321218240682999756, 5.002382960257000022 ) ) ;
#30591=ORIENTED_EDGE ( 'NONE', *, *, #17695, .F. ) ;
#30605=CONICAL_SURFACE ( 'NONE', #53012, 1.449999999966000264, 0.7853981633972997312 ) ;
#30606=CARTESIAN_POINT ( 'NONE',  ( 10.31457635473999979, -5.362146312020000138, 6.677778992223999843 ) ) ;
#30609=CARTESIAN_POINT ( 'NONE',  ( 7.571668146791999732, -2.531197775378000170, 8.216705951490000714 ) ) ;
#30618=EDGE_CURVE ( 'NONE', #46265, #68830, #56165, .T. ) ;
#30621=CARTESIAN_POINT ( 'NONE',  ( 9.967845797207999681, -2.034786297409000078, 7.636877353231999344 ) ) ;
#30626=CARTESIAN_POINT ( 'NONE',  ( 10.29094647910999782, -2.903513699412000104, -8.310923036409999298 ) ) ;
#30627=CONICAL_SURFACE ( 'NONE', #25074, 1.199999999294000252, 0.7853981633972997312 ) ;
#30633=CARTESIAN_POINT ( 'NONE',  ( 10.90000000000000036, -2.899999999999999911, 6.414037451299000381 ) ) ;
#30638=CARTESIAN_POINT ( 'NONE',  ( 8.328787166962994704, -5.102611464338999703, 6.655261220345003004 ) ) ;
#30645=CARTESIAN_POINT ( 'NONE',  ( 10.79839246847000034, -5.269358106415999110, -6.148714306659999629 ) ) ;
#30651=CARTESIAN_POINT ( 'NONE',  ( 11.09999999999999964, -2.338960882173506839, -6.969127111924879436 ) ) ;
#30655=AXIS2_PLACEMENT_3D ( 'NONE', #27079, #37218, #157 ) ;
#30667=CARTESIAN_POINT ( 'NONE',  ( 7.191894353207000101, -3.501517589953999643, 9.055975309745999624 ) ) ;
#30673=AXIS2_PLACEMENT_3D ( 'NONE', #64487, #42500, #5434 ) ;
#30686=CARTESIAN_POINT ( 'NONE',  ( 8.106698381332673620, -4.688446296872112562, 5.897672128492101429 ) ) ;
#30689=CARTESIAN_POINT ( 'NONE',  ( 10.95570209549000040, -5.337917385706000495, -4.890560488315999876 ) ) ;
#30694=CYLINDRICAL_SURFACE ( 'NONE', #61000, 1.350000000000000089 ) ;
#30708=B_SPLINE_SURFACE_WITH_KNOTS ( 'NONE', 3, 3, ( 
 ( #46506, #40563, #61547, #50720, #30097, #4181, #24144, #3833, #57323, #2814, #9424, #29756, #14688, #19589, #30767, #51401, #45815, #67464, #67809, #8413, #61890, #3497, #45475, #68152, #55961, #19933, #40910, #34992, #36007, #15027, #14006, #52077, #3162, #41254, #66792 ),
 ( #19236, #62906, #25520, #46848, #24833, #9090, #35335, #46160, #24492, #8068, #13663, #20271, #30429, #56649, #62569, #51739, #41597, #29412, #67126, #35673, #56307, #51060, #8755, #62232, #14349, #25171, #5221, #16051, #27241, #36351, #48565, #9772, #37044, #58023, #64626 ),
 ( #321, #37382, #31457, #5560, #25859, #26902, #4523, #5899, #57666, #52426, #63249, #31123, #669, #68493, #21981, #47192, #43322, #20617, #58359, #10125, #41941, #59052, #21637, #42972, #58704, #52775, #48214, #15374, #64279, #36703, #4870, #26211, #47539, #68844, #20962 ),
 ( #53467, #42300, #16396, #26557, #37723, #47884, #63598, #15716, #10461, #31803, #53119, #11154, #32489, #69188, #53802, #21300, #32151, #42630, #63940, #10807, #6938, #48910, #39454, #6242, #12888, #60773, #1354, #43668, #1018, #28273, #17790, #44712, #39108, #7289, #11836 ) ),
 .UNSPECIFIED., .F., .F., .F.,
 ( 4, 4 ),
 ( 4, 1, 1, 1, 1, 1, 1, 1, 1, 1, 1, 1, 1, 1, 1, 1, 1, 1, 1, 1, 1, 1, 1, 1, 1, 1, 1, 1, 1, 1, 1, 1, 4 ),
 ( -0.1039086239011999951, 1.103908623900999864 ),
 ( -0.02000000000000000042, 0.01250000000000000069, 0.04499999999999999833, 0.07749999999999999944, 0.1100000000000000006, 0.1424999999999999878, 0.1749999999999999889, 0.2074999999999999900, 0.2399999999999999911, 0.2725000000000000200, 0.3049999999999999933, 0.3375000000000000222, 0.3699999999999999956, 0.4025000000000000244, 0.4349999999999999978, 0.4675000000000000266, 0.5000000000000000000, 0.5324999999999999734, 0.5649999999999999467, 0.5975000000000000311, 0.6300000000000000044, 0.6624999999999999778, 0.6949999999999999512, 0.7275000000000000355, 0.7600000000000000089, 0.7924999999999999822, 0.8249999999999999556, 0.8575000000000000400, 0.8900000000000000133, 0.9224999999999999867, 0.9549999999999999600, 0.9875000000000000444, 1.020000000000000018 ),
 .UNSPECIFIED. ) ;
#30711=CARTESIAN_POINT ( 'NONE',  ( 10.43325685320999874, -5.596199512734999715, -8.042023143828998855 ) ) ;
#30733=VERTEX_POINT ( 'NONE', #22798 ) ;
#30746=CARTESIAN_POINT ( 'NONE',  ( 9.074999999999999289, -4.417172942406000224, 8.783926296998000538 ) ) ;
#30761=CARTESIAN_POINT ( 'NONE',  ( 5.599999999407000217, -1.300000000000000044, -9.662944685757000940 ) ) ;
#30766=CARTESIAN_POINT ( 'NONE',  ( 11.08757144985999865, -2.712428550139000194, 6.571291218949999902 ) ) ;
#30767=CARTESIAN_POINT ( 'NONE',  ( 8.143316940379001778, -5.061720701958000390, 5.824087910811999613 ) ) ;
#30772=CARTESIAN_POINT ( 'NONE',  ( 7.645452918061504732, -5.358307434801091063, 6.413801445279267988 ) ) ;
#30782=CARTESIAN_POINT ( 'NONE',  ( 8.472124462996665883, -5.100000000000000533, 6.567732269893666874 ) ) ;
#30784=ADVANCED_FACE ( 'NONE', ( #43792 ), #19529, .F. ) ;
#30789=CARTESIAN_POINT ( 'NONE',  ( 10.12947109217999930, -5.100000000000000533, 6.152188490330000370 ) ) ;
#30799=CARTESIAN_POINT ( 'NONE',  ( 10.18239901426000138, -2.607725299334000102, 7.783410967795999724 ) ) ;
#30806=CARTESIAN_POINT ( 'NONE',  ( 11.07074853682000004, -5.433602701969999949, -5.078288957662000058 ) ) ;
#30809=LINE ( 'NONE', #11882, #5750 ) ;
#30815=ORIENTED_EDGE ( 'NONE', *, *, #12235, .T. ) ;
#30816=CARTESIAN_POINT ( 'NONE',  ( 9.227927892482222560, -2.649889402541718120, 7.452433127320587936 ) ) ;
#30822=CARTESIAN_POINT ( 'NONE',  ( 9.476374593785998002, -5.098398394707999159, 6.305533045879999854 ) ) ;
#30829=CARTESIAN_POINT ( 'NONE',  ( 10.56498513754060653, -5.349957030113857925, -7.500000808964294663 ) ) ;
#30843=CARTESIAN_POINT ( 'NONE',  ( 9.199609130449999839, -2.551382302226000487, 7.536606162076999738 ) ) ;
#30857=CARTESIAN_POINT ( 'NONE',  ( 11.04390222146000156, -2.755558049443999735, 5.185384772327999769 ) ) ;
#30860=B_SPLINE_CURVE_WITH_KNOTS ( 'NONE', 3,
 ( #36875, #58191, #10293, #37211 ),
 .UNSPECIFIED., .F., .F.,
 ( 4, 4 ),
 ( 0.000000000000000000, 1.000000000000000000 ),
 .UNSPECIFIED. ) ;
#30862=CARTESIAN_POINT ( 'NONE',  ( 10.95934425691999792, -2.844530299042999921, -5.120733195709999741 ) ) ;
#30863=FACE_OUTER_BOUND ( 'NONE', #17549, .T. ) ;
#30869=ADVANCED_FACE ( 'NONE', ( #41551 ), #14979, .T. ) ;
#30881=DIRECTION ( 'NONE',  ( 1.000000000000000000, 0.000000000000000000, 0.000000000000000000 ) ) ;
#30882=CARTESIAN_POINT ( 'NONE',  ( 8.517351160491482887, -5.205057563154263711, 8.206039936683175995 ) ) ;
#30897=CARTESIAN_POINT ( 'NONE',  ( 10.36409408021999923, -4.600000090830000943, -4.954046131267999087 ) ) ;
#30907=CARTESIAN_POINT ( 'NONE',  ( 10.33022766388000058, -2.650179121646999647, -7.694581537458001108 ) ) ;
#30914=LINE ( 'NONE', #4666, #41344 ) ;
#30924=CARTESIAN_POINT ( 'NONE',  ( 7.736994134724001881, -2.836597362165000913, 6.822571831264003350 ) ) ;
#30926=EDGE_CURVE ( 'NONE', #34621, #55729, #15243, .T. ) ;
#30944=CARTESIAN_POINT ( 'NONE',  ( 9.152739834416941278, -2.899999737737819050, -6.597244613339529273 ) ) ;
#30945=ORIENTED_EDGE ( 'NONE', *, *, #13105, .T. ) ;
#30948=EDGE_CURVE ( 'NONE', #21776, #20897, #18255, .T. ) ;
#30950=CARTESIAN_POINT ( 'NONE',  ( 11.10000000011999965, -5.340540540232000311, -6.721892642141000351 ) ) ;
#30953=ORIENTED_EDGE ( 'NONE', *, *, #20481, .F. ) ;
#30954=AXIS2_PLACEMENT_3D ( 'NONE', #18277, #60922, #17586 ) ;
#30956=CARTESIAN_POINT ( 'NONE',  ( 11.20563089100999932, -3.509133048232999652, 6.118191305996999674 ) ) ;
#30959=CARTESIAN_POINT ( 'NONE',  ( 8.919605646795000453, -5.165500668528999917, 8.645534272955000432 ) ) ;
#30969=EDGE_LOOP ( 'NONE', ( #17360, #40098, #15572, #62101, #47444 ) ) ;
#30973=DIRECTION ( 'NONE',  ( -1.000000000000000000, 2.479407037994000336E-10, -2.337936169761000217E-09 ) ) ;
#30975=CARTESIAN_POINT ( 'NONE',  ( 10.76232069631999977, -3.259150589222000072, -8.644998763029001054 ) ) ;
#30978=ORIENTED_EDGE ( 'NONE', *, *, #8362, .T. ) ;
#30996=CARTESIAN_POINT ( 'NONE',  ( 8.881891561744774677, -3.585076488109216974, -6.197760796822787910 ) ) ;
#31000=ORIENTED_EDGE ( 'NONE', *, *, #26522, .F. ) ;
#31020=CARTESIAN_POINT ( 'NONE',  ( 7.293870559621999483, -3.416208448044999901, 6.162501393933999871 ) ) ;
#31039=CARTESIAN_POINT ( 'NONE',  ( 8.126493406597699476, -5.052135485929927228, 6.114372266853107085 ) ) ;
#31041=VERTEX_POINT ( 'NONE', #8583 ) ;
#31042=CARTESIAN_POINT ( 'NONE',  ( 10.35160840458000031, -4.633672799139000098, -4.861358447487999612 ) ) ;
#31044=VERTEX_POINT ( 'NONE', #14523 ) ;
#31048=CARTESIAN_POINT ( 'NONE',  ( 10.18225119159999892, -4.505165106450999879, -8.732017808253001334 ) ) ;
#31057=CARTESIAN_POINT ( 'NONE',  ( 9.342519353207999089, -5.057079407184000175, 8.967634647348999621 ) ) ;
#31086=CARTESIAN_POINT ( 'NONE',  ( 8.661263445375622538, -4.848494725308105657, -6.449848855944013692 ) ) ;
#31100=CARTESIAN_POINT ( 'NONE',  ( 9.218545854265867590, -2.654504660436530994, 7.609872343353834445 ) ) ;
#31101=VERTEX_POINT ( 'NONE', #3158 ) ;
#31110=ORIENTED_EDGE ( 'NONE', *, *, #58868, .T. ) ;
#31117=DIRECTION ( 'NONE',  ( 0.000000000000000000, -1.000000000000000000, 0.000000000000000000 ) ) ;
#31123=CARTESIAN_POINT ( 'NONE',  ( 7.769581853207999877, -2.431397064767999439, 7.958394431095000776 ) ) ;
#31129=CARTESIAN_POINT ( 'NONE',  ( 7.645048706201956534, -5.352880121026291071, 6.407055433046042303 ) ) ;
#31137=CARTESIAN_POINT ( 'NONE',  ( 6.953052440528999512, -9.233022020364000326, -5.200634764108000851 ) ) ;
#31149=ORIENTED_EDGE ( 'NONE', *, *, #54528, .T. ) ;
#31153=CARTESIAN_POINT ( 'NONE',  ( 10.98768553379999879, -5.299329486732999861, 4.945210549701000602 ) ) ;
#31158=CARTESIAN_POINT ( 'NONE',  ( 11.20563089100999932, -3.509133048232999652, 6.118191305996999674 ) ) ;
#31170=CARTESIAN_POINT ( 'NONE',  ( 10.74600376124999990, -5.242711034443999552, 8.978690688221998784 ) ) ;
#31178=CARTESIAN_POINT ( 'NONE',  ( 10.09697182628999990, -5.253379538902000156, 8.530665717066000298 ) ) ;
#31185=CARTESIAN_POINT ( 'NONE',  ( 10.71685100253999856, -2.832432432432000269, 6.822293592207000934 ) ) ;
#31198=CARTESIAN_POINT ( 'NONE',  ( 10.31668414895000119, -3.819528725844000494, 6.062183754159999438 ) ) ;
#31208=DIRECTION ( 'NONE',  ( 0.000000000000000000, -1.000000000000000000, 0.000000000000000000 ) ) ;
#31215=CARTESIAN_POINT ( 'NONE',  ( 11.04413069183000040, -2.755289458307000228, -5.175229826689999868 ) ) ;
#31217=CARTESIAN_POINT ( 'NONE',  ( 9.007644528443009335, -4.705791426005293765, 8.704816259181081151 ) ) ;
#31226=DIRECTION ( 'NONE',  ( 1.000000000000000000, 0.000000000000000000, 0.000000000000000000 ) ) ;
#31236=ORIENTED_EDGE ( 'NONE', *, *, #17808, .F. ) ;
#31248=EDGE_LOOP ( 'NONE', ( #40615, #64550, #61465 ) ) ;
#31251=CARTESIAN_POINT ( 'NONE',  ( 8.164556123749317607, -2.650750344902491840, 7.676799495579008870 ) ) ;
#31255=CARTESIAN_POINT ( 'NONE',  ( 10.10656447933000024, -4.887648864398999926, -6.257283015674000026 ) ) ;
#31256=EDGE_LOOP ( 'NONE', ( #30945, #57013, #43234, #7510 ) ) ;
#31268=DIRECTION ( 'NONE',  ( 0.000000000000000000, 0.000000000000000000, -1.000000000000000000 ) ) ;
#31271=CARTESIAN_POINT ( 'NONE',  ( 7.909525359152002721, -3.174976509417001491, 6.234240719816002141 ) ) ;
#31274=CARTESIAN_POINT ( 'NONE',  ( 10.43579701286999928, -2.587605342384000195, 6.390039770907999461 ) ) ;
#31301=CARTESIAN_POINT ( 'NONE',  ( 10.63462194421999918, -5.668721490782999695, 6.527259573254000635 ) ) ;
#31304=CARTESIAN_POINT ( 'NONE',  ( 7.283516392955999841, -4.426925773067000414, 9.293310812901001583 ) ) ;
#31312=CARTESIAN_POINT ( 'NONE',  ( 9.442841440870999747, -2.691258483914000355, 6.269525829285999663 ) ) ;
#31316=DIRECTION ( 'NONE',  ( 1.000000000000000000, 0.000000000000000000, 0.000000000000000000 ) ) ;
#31317=VERTEX_POINT ( 'NONE', #8999 ) ;
#31327=CARTESIAN_POINT ( 'NONE',  ( 11.01776264201000011, -4.914128622650000722, 8.587713430305999651 ) ) ;
#31345=CARTESIAN_POINT ( 'NONE',  ( 7.239688980126000040, -4.389298280625000714, 9.135255728583000945 ) ) ;
#31357=CARTESIAN_POINT ( 'NONE',  ( 8.534480646793999981, -3.011617647609999615, 8.801438026873999121 ) ) ;
#31362=ORIENTED_EDGE ( 'NONE', *, *, #29375, .T. ) ;
#31370=CARTESIAN_POINT ( 'NONE',  ( 9.190027038535603765, -5.045605306419576941, -6.289499010756019359 ) ) ;
#31377=CARTESIAN_POINT ( 'NONE',  ( 8.221162047634791747, -5.672745506483112266, 7.976212191220952263 ) ) ;
#31382=ORIENTED_EDGE ( 'NONE', *, *, #3165, .F. ) ;
#31387=CARTESIAN_POINT ( 'NONE',  ( 9.624896294737000702, -5.235394649229000663, -8.110359502241001550 ) ) ;
#31388=LINE ( 'NONE', #57250, #14850 ) ;
#31391=CARTESIAN_POINT ( 'NONE',  ( 8.709123917668916803, -5.736648055247994371, 7.709653903676097819 ) ) ;
#31396=CARTESIAN_POINT ( 'NONE',  ( 8.866808059624998961, -2.550589632307000088, 8.854674225901000284 ) ) ;
#31398=EDGE_LOOP ( 'NONE', ( #63004, #25854, #27949, #28645 ) ) ;
#31407=ADVANCED_FACE ( 'NONE', ( #67375 ), #45387, .F. ) ;
#31417=CARTESIAN_POINT ( 'NONE',  ( 10.90635170712999980, -3.089674976714000376, -6.534319251717000121 ) ) ;
#31424=ORIENTED_EDGE ( 'NONE', *, *, #30336, .F. ) ;
#31436=CARTESIAN_POINT ( 'NONE',  ( 9.162712628445618179, -3.042358984555600276, 8.452211083226405464 ) ) ;
#31457=CARTESIAN_POINT ( 'NONE',  ( 7.191894353207000101, -3.501517589953999643, 9.055975309745999624 ) ) ;
#31462=CARTESIAN_POINT ( 'NONE',  ( 7.587133471837959497, -4.278447414270965865, 5.782523221580097683 ) ) ;
#31488=CARTESIAN_POINT ( 'NONE',  ( 9.444317341922999987, -2.927260449021000355, 8.897015448164999896 ) ) ;
#31502=CARTESIAN_POINT ( 'NONE',  ( 10.63462194421999918, -5.668721490782999695, 6.527259573254000635 ) ) ;
#31505=ORIENTED_EDGE ( 'NONE', *, *, #48866, .F. ) ;
#31510=CARTESIAN_POINT ( 'NONE',  ( 10.03491210303999992, -5.615910465798999773, 7.351455544018000943 ) ) ;
#31518=CARTESIAN_POINT ( 'NONE',  ( 9.927916723342999461, -5.290169207169999943, -8.858081286661999343 ) ) ;
#31528=DIRECTION ( 'NONE',  ( 0.000000000000000000, 1.000000000000000000, 0.000000000000000000 ) ) ;
#31532=CARTESIAN_POINT ( 'NONE',  ( 9.323728576950999880, -3.947350124452999598, 6.051857392047999440 ) ) ;
#31552=LINE ( 'NONE', #58801, #43126 ) ;
#31557=B_SPLINE_CURVE_WITH_KNOTS ( 'NONE', 3,
 ( #28424, #55682, #33667, #2529 ),
 .UNSPECIFIED., .F., .F.,
 ( 4, 4 ),
 ( 0.000000000000000000, 1.000000000000000000 ),
 .UNSPECIFIED. ) ;
#31558=VERTEX_POINT ( 'NONE', #16568 ) ;
#31581=ORIENTED_EDGE ( 'NONE', *, *, #30483, .T. ) ;
#31586=CARTESIAN_POINT ( 'NONE',  ( 10.16052890781999984, -2.899999999999999911, -6.152188490330000370 ) ) ;
#31589=CARTESIAN_POINT ( 'NONE',  ( 9.769471092180999960, -5.100000000000000533, -6.152188490330000370 ) ) ;
#31595=CARTESIAN_POINT ( 'NONE',  ( 9.741009892375998902, -3.588529236307000048, -8.800227248412999970 ) ) ;
#31598=CARTESIAN_POINT ( 'NONE',  ( 10.22180282788866812, -2.874603711589704957, 6.749639981055104876 ) ) ;
#31606=CARTESIAN_POINT ( 'NONE',  ( 8.325003570449004187, -2.868532950405002779, 6.316175323229005656 ) ) ;
#31610=CARTESIAN_POINT ( 'NONE',  ( 8.076856445596000356, -2.879480170456998778, 6.727212843387002650 ) ) ;
#31612=FACE_OUTER_BOUND ( 'NONE', #859, .T. ) ;
#31613=CARTESIAN_POINT ( 'NONE',  ( 9.256662271119999730, -4.025830307267999508, 9.295859242339000517 ) ) ;
#31616=CARTESIAN_POINT ( 'NONE',  ( 10.77706886429733402, -2.899999999999999911, -6.444141223373583749 ) ) ;
#31633=LINE ( 'NONE', #47715, #56729 ) ;
#31640=CARTESIAN_POINT ( 'NONE',  ( 10.02202195053999922, -3.298019507654999849, 5.700533868754000366 ) ) ;
#31642=ORIENTED_EDGE ( 'NONE', *, *, #27491, .F. ) ;
#31644=CARTESIAN_POINT ( 'NONE',  ( 7.994581853207999522, -2.263562268490999951, 8.007440964304000985 ) ) ;
#31646=EDGE_LOOP ( 'NONE', ( #37461, #41255, #33171, #31236 ) ) ;
#31653=CARTESIAN_POINT ( 'NONE',  ( 9.662553763536999796, -4.094830574823999925, 9.119950378356000087 ) ) ;
#31671=CARTESIAN_POINT ( 'NONE',  ( 7.612571400991003046, -4.588494467460999537, 6.486759529251004075 ) ) ;
#31672=VERTEX_POINT ( 'NONE', #36274 ) ;
#31676=CARTESIAN_POINT ( 'NONE',  ( 10.90000000000000036, -8.091325576830000088, 7.077637346582999811 ) ) ;
#31688=CARTESIAN_POINT ( 'NONE',  ( 9.143918146793000190, -5.791549888895000109, 7.752110689268000954 ) ) ;
#31695=B_SPLINE_SURFACE_WITH_KNOTS ( 'NONE', 3, 3, ( 
 ( #38637, #895, #12419, #1237, #7507, #65544, #64844, #28862, #37944, #16619, #60653, #54719, #17667, #22549, #50170, #11369, #32709, #54020, #43891, #49124, #6122, #49819, #38991, #27461, #65193, #6471, #60311, #12070, #48787, #23252, #38288, #44594, #39333, #27819, #22207 ),
 ( #16955, #59615, #33051, #17312, #33402, #55066, #7167, #12767, #2610, #61683, #18699, #60998, #13119, #66580, #61344, #36405, #40032, #29554, #13462, #50509, #19033, #34785, #25915, #68203, #2950, #56094, #20322, #50856, #36758, #40360, #58079, #8205, #47246, #10182, #41649 ),
 ( #52482, #9479, #35129, #62956, #24283, #45617, #15431, #30822, #52134, #68549, #15080, #52831, #57722, #4929, #4236, #9830, #31510, #31178, #4579, #23941, #26264, #56443, #20671, #25576, #46902, #41999, #66923, #13799, #18357, #66238, #63304, #39679, #34448, #55761, #7863 ),
 ( #45274, #29197, #68901, #47594, #43381, #58413, #6298, #65020, #17137, #64681, #63653, #59444, #10517, #26614, #21691, #59103, #47933, #21017, #374, #1072, #16109, #32207, #723, #53857, #54553, #33234, #37778, #15770, #32886, #48268, #31857, #5956, #37099, #53172, #53521 ) ),
 .UNSPECIFIED., .F., .F., .F.,
 ( 4, 4 ),
 ( 4, 1, 1, 1, 1, 1, 1, 1, 1, 1, 1, 1, 1, 1, 1, 1, 1, 1, 1, 1, 1, 1, 1, 1, 1, 1, 1, 1, 1, 1, 1, 1, 4 ),
 ( -0.1039086239011999951, 1.103908623900999864 ),
 ( -0.01933701211302999920, 0.01208563257065999909, 0.04350827725433999843, 0.07493092193802000645, 0.1063535666217000075, 0.1377762113054000204, 0.1691988559891000055, 0.2006215006727000150, 0.2320441453564000001, 0.2634667900400999851, 0.2948894347238000258, 0.3263120794074999553, 0.3577347240911999959, 0.3891573687748000054, 0.4205800134584999905, 0.4520026581421999756, 0.4834253028259000162, 0.5148479475096000568, 0.5462705921932000663, 0.5776932368768999959, 0.6091158815606000365, 0.6405385262443000771, 0.6719611709280000067, 0.7033838156117000473, 0.7348064602953000568, 0.7662291049789999864, 0.7976517496627000270, 0.8290743943464000676, 0.8604970390300999972, 0.8919196837138000378, 0.9233423283974000473, 0.9547649730810999769, 0.9861876177648000175 ),
 .UNSPECIFIED. ) ;
#31699=CARTESIAN_POINT ( 'NONE',  ( 8.662855646795000197, -2.741638482234999952, 6.457327039244000311 ) ) ;
#31705=ORIENTED_EDGE ( 'NONE', *, *, #27387, .T. ) ;
#31713=CARTESIAN_POINT ( 'NONE',  ( 9.166037027449048580, -5.069767017855149938, -6.374457060939750619 ) ) ;
#31715=CARTESIAN_POINT ( 'NONE',  ( 7.100000000000000533, -4.000000000000000000, 8.849999999999999645 ) ) ;
#31720=CARTESIAN_POINT ( 'NONE',  ( 8.414009964596925073, -2.427229585700388270, 8.242459441677670640 ) ) ;
#31723=ORIENTED_EDGE ( 'NONE', *, *, #22466, .F. ) ;
#31726=ORIENTED_EDGE ( 'NONE', *, *, #1566, .F. ) ;
#31732=CARTESIAN_POINT ( 'NONE',  ( 9.837291465645295219, -2.697790585206812697, -7.971620370481231177 ) ) ;
#31734=VECTOR ( 'NONE', #27067, 1000.000000000000114 ) ;
#31736=CARTESIAN_POINT ( 'NONE',  ( 8.616995677562000466, -4.876077402042000131, 5.996974966533000106 ) ) ;
#31756=EDGE_LOOP ( 'NONE', ( #33817, #1213, #18060, #35864, #9030 ) ) ;
#31757=ORIENTED_EDGE ( 'NONE', *, *, #68210, .F. ) ;
#31768=ORIENTED_EDGE ( 'NONE', *, *, #55444, .F. ) ;
#31769=CARTESIAN_POINT ( 'NONE',  ( 10.11501430098003773, -5.350017391163235381, -7.499999134156934311 ) ) ;
#31780=CARTESIAN_POINT ( 'NONE',  ( 9.084331191192241306, -4.271986494075218133, 8.830896599738281338 ) ) ;
#31781=ORIENTED_EDGE ( 'NONE', *, *, #21380, .F. ) ;
#31791=CARTESIAN_POINT ( 'NONE',  ( 10.51013099342176282, -2.732991197599094590, 6.289013820405174648 ) ) ;
#31797=ORIENTED_EDGE ( 'NONE', *, *, #701, .T. ) ;
#31802=CARTESIAN_POINT ( 'NONE',  ( 10.42595817177000050, -5.042180160032999403, 8.702227297563000619 ) ) ;
#31803=CARTESIAN_POINT ( 'NONE',  ( 7.550620559621999739, -4.468370631666999770, 8.882152684713000568 ) ) ;
#31807=CARTESIAN_POINT ( 'NONE',  ( 10.53198305961999992, -2.323723769066000422, -8.279488812962998878 ) ) ;
#31808=CARTESIAN_POINT ( 'NONE',  ( 7.610024113606670859, -4.741952135465052010, 5.926164387956666779 ) ) ;
#31826=ORIENTED_EDGE ( 'NONE', *, *, #39187, .F. ) ;
#31828=CARTESIAN_POINT ( 'NONE',  ( 9.610944094206999466, -5.100000000000000533, -6.571291218949999902 ) ) ;
#31833=CARTESIAN_POINT ( 'NONE',  ( 10.52462472184161157, -2.899999999999999911, -6.445686799303610215 ) ) ;
#31836=CARTESIAN_POINT ( 'NONE',  ( 9.242349231304000767, -5.206700957550999931, 8.808818370147001531 ) ) ;
#31846=ADVANCED_FACE ( 'NONE', ( #39731 ), #61049, .F. ) ;
#31857=CARTESIAN_POINT ( 'NONE',  ( 10.81316193496000011, -3.756072284922999938, 6.071597915422999314 ) ) ;
#31866=DIRECTION ( 'NONE',  ( -1.000000000000000000, 0.000000000000000000, 0.000000000000000000 ) ) ;
#31879=CARTESIAN_POINT ( 'NONE',  ( 10.97865453029000093, -5.273142482194999481, 7.958032781726000593 ) ) ;
#31886=CARTESIAN_POINT ( 'NONE',  ( 9.518359312500532354, -5.126777126183463373, -6.752018918868714970 ) ) ;
#31888=ADVANCED_FACE ( 'NONE', ( #23639 ), #50201, .T. ) ;
#31892=CARTESIAN_POINT ( 'NONE',  ( 9.710765758303409712, -3.646727114448458984, -8.814525660484084923 ) ) ;
#31898=CARTESIAN_POINT ( 'NONE',  ( 10.26694555961999988, -5.500014128486999887, -6.419508248405999318 ) ) ;
#31915=CARTESIAN_POINT ( 'NONE',  ( 9.849204462306733632, -2.899999999999999911, -6.662590550601113826 ) ) ;
#31918=CARTESIAN_POINT ( 'NONE',  ( 7.000000000000000888, -7.162101251533245616, -3.226271710805416415 ) ) ;
#31920=ORIENTED_EDGE ( 'NONE', *, *, #35696, .T. ) ;
#31942=CARTESIAN_POINT ( 'NONE',  ( 10.81362580514000094, -3.876947229615999913, -9.022210119840998743 ) ) ;
#31959=CARTESIAN_POINT ( 'NONE',  ( 10.31664229535000032, -3.425746660654999776, -4.565089086486000092 ) ) ;
#31962=ADVANCED_FACE ( 'NONE', ( #22510 ), #30627, .F. ) ;
#31963=CARTESIAN_POINT ( 'NONE',  ( 9.719606904206999687, -5.967761543230999166, 7.406644089178000101 ) ) ;
#31972=VECTOR ( 'NONE', #9507, 1000.000000000000000 ) ;
#31977=VERTEX_POINT ( 'NONE', #64807 ) ;
#31979=CARTESIAN_POINT ( 'NONE',  ( 10.02462472190973486, -2.899999999999999911, -6.445686799157789082 ) ) ;
#31993=CARTESIAN_POINT ( 'NONE',  ( 10.83659005484000026, -5.133183563847000030, 8.848364935581999546 ) ) ;
#31997=CARTESIAN_POINT ( 'NONE',  ( 7.737831853206999178, -5.687202994508999687, 6.847270485579000088 ) ) ;
#32000=LINE ( 'NONE', #37232, #58745 ) ;
#32007=CARTESIAN_POINT ( 'NONE',  ( 10.49785673611999925, -3.776281940467000275, 5.717636230565000588 ) ) ;
#32010=ORIENTED_EDGE ( 'NONE', *, *, #67909, .T. ) ;
#32013=CARTESIAN_POINT ( 'NONE',  ( 11.25809194037999994, -3.275508415657999883, -8.650784343212000849 ) ) ;
#32026=ORIENTED_EDGE ( 'NONE', *, *, #59174, .T. ) ;
#32039=CARTESIAN_POINT ( 'NONE',  ( 8.758793146794999984, -3.977267280662000193, 9.308921106447000327 ) ) ;
#32049=CARTESIAN_POINT ( 'NONE',  ( 8.791230646795000325, -5.095088356574999366, 6.286978111459999852 ) ) ;
#32050=CARTESIAN_POINT ( 'NONE',  ( 9.026933059621999433, -4.852736108563000528, 8.683927195503999386 ) ) ;
#32052=EDGE_CURVE ( 'NONE', #68446, #11689, #32570, .T. ) ;
#32060=ORIENTED_EDGE ( 'NONE', *, *, #744, .T. ) ;
#32064=CARTESIAN_POINT ( 'NONE',  ( 7.929178192470822673, -4.758525843572996905, 6.310451091254675404 ) ) ;
#32071=CARTESIAN_POINT ( 'NONE',  ( 8.414772878883319152, -2.420192783774375300, 8.227318774112935884 ) ) ;
#32074=ORIENTED_EDGE ( 'NONE', *, *, #52554, .T. ) ;
#32078=EDGE_CURVE ( 'NONE', #18362, #56639, #26761, .T. ) ;
#32080=CARTESIAN_POINT ( 'NONE',  ( 7.720433716083946685, -2.879779226720537100, 6.726083684511015015 ) ) ;
#32083=CARTESIAN_POINT ( 'NONE',  ( 10.57899597767938360, -2.241951334100745985, -7.748279897758227008 ) ) ;
#32088=ORIENTED_EDGE ( 'NONE', *, *, #39228, .F. ) ;
#32090=ORIENTED_EDGE ( 'NONE', *, *, #13105, .F. ) ;
#32096=DIRECTION ( 'NONE',  ( -8.896584015454000239E-13, 1.000000000000000000, -2.557804911864000007E-11 ) ) ;
#32104=CARTESIAN_POINT ( 'NONE',  ( 11.12372457444999974, -5.764773383430000564, -5.184664793151999795 ) ) ;
#32105=ORIENTED_EDGE ( 'NONE', *, *, #44390, .F. ) ;
#32116=ORIENTED_EDGE ( 'NONE', *, *, #62502, .T. ) ;
#32140=VERTEX_POINT ( 'NONE', #25624 ) ;
#32142=CARTESIAN_POINT ( 'NONE',  ( 9.293536308086499886, -2.899999999999999911, 6.665341197412895546 ) ) ;
#32150=CARTESIAN_POINT ( 'NONE',  ( 11.27765354842000001, -3.273798832483999721, 6.368296067120999382 ) ) ;
#32151=CARTESIAN_POINT ( 'NONE',  ( 7.999933059623999476, -5.198566224659999513, 8.332559954171999905 ) ) ;
#32154=CARTESIAN_POINT ( 'NONE',  ( 9.975298369746534277, -5.350379160513648813, 7.499985214262776978 ) ) ;
#32155=CARTESIAN_POINT ( 'NONE',  ( 10.77401935321000082, -3.826867196099999813, -5.823197386290999589 ) ) ;
#32156=CARTESIAN_POINT ( 'NONE',  ( 7.785931005785818648, -4.810406945106828758, 9.044821997675690284 ) ) ;
#32157=CARTESIAN_POINT ( 'NONE',  ( 9.905786073958001481, -2.698967003257000119, 8.979227319929000473 ) ) ;
#32183=CARTESIAN_POINT ( 'NONE',  ( 10.22399006116000031, -5.507891002176999784, 6.589804341508000540 ) ) ;
#32194=CARTESIAN_POINT ( 'NONE',  ( 9.214598350273000449, -3.399999999999999911, -6.571291218959999902 ) ) ;
#32198=ADVANCED_FACE ( 'NONE', ( #4288 ), #9884, .T. ) ;
#32201=CARTESIAN_POINT ( 'NONE',  ( 9.245061313321260243, -2.690435683193665550, 7.172319517079158935 ) ) ;
#32207=CARTESIAN_POINT ( 'NONE',  ( 10.25462442569999943, -2.860634389522000109, 6.604605425112000994 ) ) ;
#32212=CARTESIAN_POINT ( 'NONE',  ( 7.752942703112657874, -2.713880210350901656, 7.026314146705725072 ) ) ;
#32247=CARTESIAN_POINT ( 'NONE',  ( 10.31905590579000176, -2.899999999999999911, -6.571291218949999902 ) ) ;
#32248=CARTESIAN_POINT ( 'NONE',  ( 10.18308064679000147, -2.953580299898999950, -8.606287508253000595 ) ) ;
#32257=CARTESIAN_POINT ( 'NONE',  ( 11.09999999999999964, -4.000000000000000000, 7.500000000000000000 ) ) ;
#32269=CARTESIAN_POINT ( 'NONE',  ( 10.48735240295000004, -4.351290250877999810, -6.182246784057000788 ) ) ;
#32284=ADVANCED_FACE ( 'NONE', ( #15134 ), #64038, .F. ) ;
#32288=CARTESIAN_POINT ( 'NONE',  ( 9.824592608787908077, -5.732646222183269025, -7.158320533632580585 ) ) ;
#32293=CARTESIAN_POINT ( 'NONE',  ( 10.71983009893999927, -3.571743996388999864, -5.696159701115999674 ) ) ;
#32294=ORIENTED_EDGE ( 'NONE', *, *, #40342, .F. ) ;
#32298=CARTESIAN_POINT ( 'NONE',  ( 8.642330585105490570, -3.079257296649804410, -6.512589459674783754 ) ) ;
#32299=CARTESIAN_POINT ( 'NONE',  ( 8.579946306764748343, -2.950101199909312744, 6.243999687575779944 ) ) ;
#32305=CARTESIAN_POINT ( 'NONE',  ( 8.200208800211990834, -2.889590298673998081, 6.692105494707000446 ) ) ;
#32307=CARTESIAN_POINT ( 'NONE',  ( 8.221178267935991713, -3.443155653785000769, 6.131664341583003441 ) ) ;
#32309=FACE_OUTER_BOUND ( 'NONE', #4769, .T. ) ;
#32310=CARTESIAN_POINT ( 'NONE',  ( 10.31167756636999933, -2.874479384703000129, 8.900026329558999194 ) ) ;
#32323=CARTESIAN_POINT ( 'NONE',  ( 6.826133408972999916, -9.284776586335999227, -5.366079628331000606 ) ) ;
#32337=CARTESIAN_POINT ( 'NONE',  ( 10.94797187187000098, -2.864324950622999744, 8.846246404612999825 ) ) ;
#32339=VERTEX_POINT ( 'NONE', #54433 ) ;
#32341=CARTESIAN_POINT ( 'NONE',  ( 9.304730646793998972, -5.284133759825000887, 6.489273023403000273 ) ) ;
#32345=CARTESIAN_POINT ( 'NONE',  ( 11.09999999999999964, -2.649999999999999911, 7.500000000000000000 ) ) ;
#32348=CARTESIAN_POINT ( 'NONE',  ( 9.215289122285998502, -4.861979632688999686, 8.938813901364000003 ) ) ;
#32353=CARTESIAN_POINT ( 'NONE',  ( 7.744301838472999577, -3.130384865731000055, 6.467396727560999814 ) ) ;
#32369=DIRECTION ( 'NONE',  ( 1.000000000000000000, 0.000000000000000000, 0.000000000000000000 ) ) ;
#32382=CARTESIAN_POINT ( 'NONE',  ( 8.913566940379999082, -2.550589632307000088, 8.854674225901000284 ) ) ;
#32393=CARTESIAN_POINT ( 'NONE',  ( 9.342519353207999089, -5.057079407184000175, 8.967634647348999621 ) ) ;
#32406=DIRECTION ( 'NONE',  ( 0.000000000000000000, -1.000000000000000000, 0.000000000000000000 ) ) ;
#32411=CARTESIAN_POINT ( 'NONE',  ( 8.384287192004888922, -2.818189082097684039, 8.777095765030843211 ) ) ;
#32413=EDGE_LOOP ( 'NONE', ( #39891, #68148, #61598, #66430 ) ) ;
#32422=CARTESIAN_POINT ( 'NONE',  ( 11.03483424351999886, -8.048618767883999325, 7.048979873803999929 ) ) ;
#32442=B_SPLINE_CURVE_WITH_KNOTS ( 'NONE', 3,
 ( #64326, #16448, #11205, #53856 ),
 .UNSPECIFIED., .F., .F.,
 ( 4, 4 ),
 ( 0.000000000000000000, 1.000000000000000000 ),
 .UNSPECIFIED. ) ;
#32445=ORIENTED_EDGE ( 'NONE', *, *, #28582, .T. ) ;
#32451=CARTESIAN_POINT ( 'NONE',  ( 10.33022766388000058, -2.650179121646999647, -7.694581537458001108 ) ) ;
#32456=CARTESIAN_POINT ( 'NONE',  ( 11.09999999999999964, -5.299316147296000423, 5.124965750789000296 ) ) ;
#32488=CARTESIAN_POINT ( 'NONE',  ( 9.590594544025000445, -2.445960766574000189, 7.841185849078001091 ) ) ;
#32489=CARTESIAN_POINT ( 'NONE',  ( 7.743183059623000020, -2.735207418315000361, 6.771977475428999860 ) ) ;
#32490=ORIENTED_EDGE ( 'NONE', *, *, #64028, .F. ) ;
#32493=CARTESIAN_POINT ( 'NONE',  ( 10.13035685320999946, -2.409329538444999752, -8.058042649154000259 ) ) ;
#32494=CARTESIAN_POINT ( 'NONE',  ( 7.754005127114919738, -5.344455520341463206, 8.603494402914543926 ) ) ;
#32495=CARTESIAN_POINT ( 'NONE',  ( 9.471368011205999693, -2.030678448189000118, 7.549764202121000523 ) ) ;
#32512=AXIS2_PLACEMENT_3D ( 'NONE', #19977, #41299, #62607 ) ;
#32519=CARTESIAN_POINT ( 'NONE',  ( 11.14993998249000029, -2.627133311863999676, 6.696092388640000337 ) ) ;
#32526=ADVANCED_FACE ( 'NONE', ( #18677 ), #34074, .T. ) ;
#32528=ADVANCED_FACE ( 'NONE', ( #17647 ), #64087, .F. ) ;
#32538=ORIENTED_EDGE ( 'NONE', *, *, #19837, .F. ) ;
#32554=( BOUNDED_SURFACE ( )  B_SPLINE_SURFACE ( 3, 3, ( 
 ( #15860, #69000, #42096, #5373, #32305, #63050, #21112, #4672, #57821, #20420, #9578 ),
 ( #42780, #31606, #58855, #53614, #10273, #48365, #52928, #5024, #21789, #52578, #26014 ),
 ( #43123, #14838, #47343, #36159, #57471, #52233, #46999, #63404, #20766, #68301, #9930 ),
 ( #58172, #39265, #16549, #22828, #54296, #11642, #44176, #17597, #7439, #17945, #37879 ) ),
 .UNSPECIFIED., .F., .F., .F. ) 
 B_SPLINE_SURFACE_WITH_KNOTS ( ( 4, 4 ),
 ( 4, 1, 1, 1, 1, 1, 1, 1, 4 ),
 ( 0.000000000000000000, 1.000000000000000000 ),
 ( -0.004668278336391999857, 0.000000000000000000, 0.03269534097185999855, 0.06255479614191999937, 0.08986301827556000821, 0.1148786485006000058, 0.1378153831697999931, 0.1587710662428999941, 0.1687086804768000159 ),
 .UNSPECIFIED. ) 
 GEOMETRIC_REPRESENTATION_ITEM ( )  RATIONAL_B_SPLINE_SURFACE ( (
 ( 1.221011660805000121, 1.221011660805000121, 1.221011660805000121, 1.221011660805000121, 1.221011660805000121, 1.221011660805000121, 1.221011660805000121, 1.221011660805000121, 1.221011660805000121, 1.221011660805000121, 1.221011660805000121),
 ( 0.9263294463983999805, 0.9263294463983999805, 0.9263294463983999805, 0.9263294463983999805, 0.9263294463983999805, 0.9263294463983999805, 0.9263294463983999805, 0.9263294463983999805, 0.9263294463983999805, 0.9263294463983999805, 0.9263294463983999805),
 ( 0.9263294463983999805, 0.9263294463983999805, 0.9263294463983999805, 0.9263294463983999805, 0.9263294463983999805, 0.9263294463983999805, 0.9263294463983999805, 0.9263294463983999805, 0.9263294463983999805, 0.9263294463983999805, 0.9263294463983999805),
 ( 1.221011660805000121, 1.221011660805000121, 1.221011660805000121, 1.221011660805000121, 1.221011660805000121, 1.221011660805000121, 1.221011660805000121, 1.221011660805000121, 1.221011660805000121, 1.221011660805000121, 1.221011660805000121) ) ) 
 REPRESENTATION_ITEM ( '' )  SURFACE ( )  );
#32570=B_SPLINE_CURVE_WITH_KNOTS ( 'NONE', 3,
 ( #61309, #29164, #56410, #19001, #56760, #29520, #51500, #40665, #46613, #57088, #9188, #40328, #50473, #35434, #3597, #3940, #13764, #56060 ),
 .UNSPECIFIED., .F., .F.,
 ( 4, 2, 2, 2, 2, 2, 2, 2, 4 ),
 ( 0.000000000000000000, 0.1250000000000000000, 0.2500000000000000000, 0.3750000000000000000, 0.5000000000000000000, 0.6250000000000000000, 0.7500000000000000000, 0.8750000000000000000, 1.000000000000000000 ),
 .UNSPECIFIED. ) ;
#32573=CARTESIAN_POINT ( 'NONE',  ( 9.617013408676374553, -5.079309631299753214, -8.329427714267961136 ) ) ;
#32580=DIRECTION ( 'NONE',  ( 0.000000000000000000, -1.000000000000000000, 0.000000000000000000 ) ) ;
#32581=CARTESIAN_POINT ( 'NONE',  ( 10.75101814679000078, -2.478465696309000155, -7.438303690845000204 ) ) ;
#32597=B_SPLINE_CURVE_WITH_KNOTS ( 'NONE', 3,
 ( #58877, #31979, #58528, #5045 ),
 .UNSPECIFIED., .F., .F.,
 ( 4, 4 ),
 ( 0.000000000000000000, 1.000000000000000000 ),
 .UNSPECIFIED. ) ;
#32601=CARTESIAN_POINT ( 'NONE',  ( 10.69578225082999978, -5.505007625740000243, -7.759264430206000540 ) ) ;
#32614=CARTESIAN_POINT ( 'NONE',  ( 10.59991574914826451, -2.968501058370544232, 5.041504506945282849 ) ) ;
#32616=CARTESIAN_POINT ( 'NONE',  ( 10.46085355684000007, -5.403406918566000527, 7.721809917403000156 ) ) ;
#32617=CARTESIAN_POINT ( 'NONE',  ( 8.433148997460000018, -5.167567567567999731, 6.822293592207000934 ) ) ;
#32629=CARTESIAN_POINT ( 'NONE',  ( 10.13061232742999884, -2.189322372303999842, -7.101642112140999608 ) ) ;
#32643=CARTESIAN_POINT ( 'NONE',  ( 9.691080333872001518, -5.335644368206000188, 8.701217921043999937 ) ) ;
#32646=CARTESIAN_POINT ( 'NONE',  ( 9.657547180956999711, -5.333447643521000536, 6.049925825719999928 ) ) ;
#32647=CARTESIAN_POINT ( 'NONE',  ( 9.889653591487839179, -2.705485811107797289, 8.717674038414637394 ) ) ;
#32648=CARTESIAN_POINT ( 'NONE',  ( 10.81905590578999998, -2.899999999999999911, -6.571291218949999902 ) ) ;
#32671=AXIS2_PLACEMENT_3D ( 'NONE', #53068, #10408, #16684 ) ;
#32673=CARTESIAN_POINT ( 'NONE',  ( 10.91307648679999964, -2.096298111716999646, 7.827187677719999570 ) ) ;
#32675=EDGE_LOOP ( 'NONE', ( #34552, #39213, #15385, #11142, #56916 ) ) ;
#32677=CARTESIAN_POINT ( 'NONE',  ( 8.738433059624998833, -5.414909314743000301, 8.890670256079998168 ) ) ;
#32685=CARTESIAN_POINT ( 'NONE',  ( 10.28315099603999982, -2.387772357283999725, 7.684266429524000408 ) ) ;
#32689=CARTESIAN_POINT ( 'NONE',  ( 10.72801694037999987, -3.751276547904999870, -8.836912395451999913 ) ) ;
#32699=CARTESIAN_POINT ( 'NONE',  ( 9.326707230296040763, -3.961060040642459423, 9.239254357279243379 ) ) ;
#32706=VECTOR ( 'NONE', #48812, 1000.000000000000000 ) ;
#32709=CARTESIAN_POINT ( 'NONE',  ( 10.21608469020999976, -5.961703525007000515, 7.319668113368000384 ) ) ;
#32717=CARTESIAN_POINT ( 'NONE',  ( 9.634027193201999850, -3.042970193091000031, 8.588108172435999776 ) ) ;
#32719=CARTESIAN_POINT ( 'NONE',  ( 8.721004440379999778, -5.983034890242000081, 7.440798487724999966 ) ) ;
#32722=CARTESIAN_POINT ( 'NONE',  ( 9.819055905797000605, -2.899999999999999911, -6.571291218949999902 ) ) ;
#32731=CARTESIAN_POINT ( 'NONE',  ( 7.481081853206999810, -2.374041291348000016, 8.293390875797999939 ) ) ;
#32733=CARTESIAN_POINT ( 'NONE',  ( 10.90000000296000060, -5.100000000009000445, 5.160242730682999657 ) ) ;
#32734=CARTESIAN_POINT ( 'NONE',  ( 9.118435835444707038, -5.100000000000000533, 6.178531823617834817 ) ) ;
#32739=EDGE_CURVE ( 'NONE', #6003, #4443, #47394, .T. ) ;
#32744=CARTESIAN_POINT ( 'NONE',  ( 7.890669427268998781, -4.660296165433000404, 6.322498843348999920 ) ) ;
#32749=EDGE_CURVE ( 'NONE', #52849, #46692, #17243, .T. ) ;
#32752=CARTESIAN_POINT ( 'NONE',  ( 8.359995882382332155, -3.256579615318050624, 9.091912762848693319 ) ) ;
#32755=CARTESIAN_POINT ( 'NONE',  ( 10.06493315628555862, -5.349942305088194239, -7.500003965376651038 ) ) ;
#32766=CARTESIAN_POINT ( 'NONE',  ( 8.987238607305510385, -2.413693965082394310, 6.702889251169676932 ) ) ;
#32778=VECTOR ( 'NONE', #12933, 1000.000000000000000 ) ;
#32799=CARTESIAN_POINT ( 'NONE',  ( 10.87835931249053267, -5.126777126165768195, 6.752018918838227357 ) ) ;
#32816=VERTEX_POINT ( 'NONE', #6672 ) ;
#32827=CARTESIAN_POINT ( 'NONE',  ( 11.24052627608000066, -2.774025043188999895, 6.782107572692000375 ) ) ;
#32830=VERTEX_POINT ( 'NONE', #19415 ) ;
#32837=CARTESIAN_POINT ( 'NONE',  ( 11.26847231345999845, -2.565616654150999931, -7.116622328138999976 ) ) ;
#32838=CARTESIAN_POINT ( 'NONE',  ( 7.806951053071116142, -4.387620322963519115, 9.195870376599991403 ) ) ;
#32839=CARTESIAN_POINT ( 'NONE',  ( 9.815199780373001559, -2.813634733202999616, 8.848854270764999086 ) ) ;
#32841=ORIENTED_EDGE ( 'NONE', *, *, #42613, .F. ) ;
#32851=ADVANCED_FACE ( 'NONE', ( #58929 ), #65242, .T. ) ;
#32853=CARTESIAN_POINT ( 'NONE',  ( 11.09999999999999964, -6.354980837003999738, -5.388690576903999663 ) ) ;
#32854=ORIENTED_EDGE ( 'NONE', *, *, #17695, .T. ) ;
#32856=CARTESIAN_POINT ( 'NONE',  ( 11.00000000000000000, -5.200000000000000178, -5.864181267619000160 ) ) ;
#32864=DIRECTION ( 'NONE',  ( -0.000000000000000000, 1.000000000000000000, 0.000000000000000000 ) ) ;
#32886=CARTESIAN_POINT ( 'NONE',  ( 10.68904248846000016, -2.568964727443000307, 7.728094434513999467 ) ) ;
#32920=CONICAL_SURFACE ( 'NONE', #2780, 1.449999999965999375, 0.7853981633972997312 ) ;
#32922=DIRECTION ( 'NONE',  ( 0.8843050093870327144, 0.1786786010978065053, -0.4313682972620159761 ) ) ;
#32923=CARTESIAN_POINT ( 'NONE',  ( 10.84974435320999930, -5.265000209383999596, -6.385811305909999902 ) ) ;
#32945=CARTESIAN_POINT ( 'NONE',  ( 10.18512684885999953, -5.526147823900999789, -7.556025229989000280 ) ) ;
#32969=CARTESIAN_POINT ( 'NONE',  ( 10.28773706650000008, -5.077599250153999932, -5.991350640809000261 ) ) ;
#32983=EDGE_LOOP ( 'NONE', ( #64355, #41635, #3535, #68318 ) ) ;
#32985=CARTESIAN_POINT ( 'NONE',  ( 9.347248564704999652, -4.028326926800000152, 9.469437404464001062 ) ) ;
#32988=CARTESIAN_POINT ( 'NONE',  ( 11.06924082387999952, -5.425685649895999774, 8.012912555523998392 ) ) ;
#32993=EDGE_CURVE ( 'NONE', #37807, #36315, #5803, .T. ) ;
#33017=ORIENTED_EDGE ( 'NONE', *, *, #45232, .F. ) ;
#33027=CARTESIAN_POINT ( 'NONE',  ( 10.45746213570999927, -5.100000000000000533, -6.571291218949999902 ) ) ;
#33030=CARTESIAN_POINT ( 'NONE',  ( 9.075489683949001574, -4.020837068201999820, 8.948702918089999514 ) ) ;
#33035=CARTESIAN_POINT ( 'NONE',  ( 10.23580444037999904, -3.621838308198000345, -8.806219190581000333 ) ) ;
#33045=ORIENTED_EDGE ( 'NONE', *, *, #57129, .F. ) ;
#33051=CARTESIAN_POINT ( 'NONE',  ( 9.256662271119999730, -4.025830307267999508, 9.295859242339000517 ) ) ;
#33062=CARTESIAN_POINT ( 'NONE',  ( 10.25462442569999943, -2.860634389522000109, 6.604605425112000994 ) ) ;
#33064=CARTESIAN_POINT ( 'NONE',  ( 7.871558059623000148, -4.780993534312999671, 6.267212032957000467 ) ) ;
#33075=CARTESIAN_POINT ( 'NONE',  ( 11.09999999999999964, -5.299999999999999822, 6.469505845987999493 ) ) ;
#33078=CARTESIAN_POINT ( 'NONE',  ( 7.839808059622000336, -3.084082018960999871, 9.259837032825000591 ) ) ;
#33081=EDGE_CURVE ( 'NONE', #8185, #29320, #47560, .T. ) ;
#33094=ORIENTED_EDGE ( 'NONE', *, *, #40728, .F. ) ;
#33097=CARTESIAN_POINT ( 'NONE',  ( 8.347296311784370815, -3.523203782693021591, 9.195961815643585169 ) ) ;
#33105=EDGE_CURVE ( 'NONE', #41119, #5164, #39590, .T. ) ;
#33112=CARTESIAN_POINT ( 'NONE',  ( 8.788005865575000186, -3.396241925389000382, -6.276539452210999848 ) ) ;
#33121=LINE ( 'NONE', #53409, #49137 ) ;
#33126=DIRECTION ( 'NONE',  ( 0.000000000000000000, 1.000000000000000000, 0.000000000000000000 ) ) ;
#33139=CARTESIAN_POINT ( 'NONE',  ( 10.66852499011999988, -4.435470817312999969, -5.866470266317000082 ) ) ;
#33145=EDGE_LOOP ( 'NONE', ( #67731, #19167, #43626, #31581 ) ) ;
#33158=ORIENTED_EDGE ( 'NONE', *, *, #25281, .T. ) ;
#33166=CARTESIAN_POINT ( 'NONE',  ( 10.67956456102511886, -4.176706786694480478, -8.849774126559321274 ) ) ;
#33171=ORIENTED_EDGE ( 'NONE', *, *, #8880, .F. ) ;
#33175=CARTESIAN_POINT ( 'NONE',  ( 9.757667269575000191, -4.489271889653999814, 5.986031004145000445 ) ) ;
#33180=CARTESIAN_POINT ( 'NONE',  ( 10.73615685320999980, -3.078046833211999900, -6.088743704655001032 ) ) ;
#33181=CARTESIAN_POINT ( 'NONE',  ( 7.738470611522092923, -5.540180350881191096, 8.309424268451294893 ) ) ;
#33182=CARTESIAN_POINT ( 'NONE',  ( 9.347248564704999652, -4.028326926800000152, 9.469437404464001062 ) ) ;
#33187=EDGE_CURVE ( 'NONE', #42061, #67307, #9444, .T. ) ;
#33196=ORIENTED_EDGE ( 'NONE', *, *, #39934, .F. ) ;
#33200=ORIENTED_EDGE ( 'NONE', *, *, #51955, .T. ) ;
#33202=DIRECTION ( 'NONE',  ( 0.7071067811865475727, 0.7071067811865475727, 0.000000000000000000 ) ) ;
#33203=ORIENTED_EDGE ( 'NONE', *, *, #56274, .F. ) ;
#33207=CARTESIAN_POINT ( 'NONE',  ( 10.75915805961999894, -5.387268372866000021, -6.278119777966000292 ) ) ;
#33210=CARTESIAN_POINT ( 'NONE',  ( 10.85738557828999973, -2.754556666341999804, 8.976367391363998749 ) ) ;
#33217=VECTOR ( 'NONE', #52265, 1000.000000000000114 ) ;
#33225=CIRCLE ( 'NONE', #12004, 1.250000000000000000 ) ;
#33230=EDGE_LOOP ( 'NONE', ( #15576, #17565, #12126, #63810, #45156 ) ) ;
#33234=CARTESIAN_POINT ( 'NONE',  ( 10.50286331871000023, -5.158900740613000302, 8.369962360110999811 ) ) ;
#33256=VECTOR ( 'NONE', #28452, 1000.000000000000000 ) ;
#33262=CARTESIAN_POINT ( 'NONE',  ( 8.702564146836854420, -2.714984396920495868, 7.027277620402951896 ) ) ;
#33269=CARTESIAN_POINT ( 'NONE',  ( 10.90000000000000036, -2.899999999999999911, -6.571291218949999902 ) ) ;
#33276=CARTESIAN_POINT ( 'NONE',  ( 11.20536814679000059, -2.688541832249000230, -8.273932507170000505 ) ) ;
#33279=CARTESIAN_POINT ( 'NONE',  ( 10.98768472639999949, -0.3876847264043000174, -4.945212061661000469 ) ) ;
#33280=CARTESIAN_POINT ( 'NONE',  ( 9.214598350275000627, -4.599999999999999645, -6.571291218958999814 ) ) ;
#33287=VERTEX_POINT ( 'NONE', #2868 ) ;
#33290=CARTESIAN_POINT ( 'NONE',  ( 10.35685100253999913, -2.832432432432000269, -6.822293592207000934 ) ) ;
#33293=LINE ( 'NONE', #36219, #67393 ) ;
#33295=CARTESIAN_POINT ( 'NONE',  ( 9.922182479546000522, -3.489927462211000364, -9.111803974470001677 ) ) ;
#33296=CARTESIAN_POINT ( 'NONE',  ( 10.00991387826809920, -4.592587181568636545, -8.996716702657641562 ) ) ;
#33303=CARTESIAN_POINT ( 'NONE',  ( 11.08518686003000120, -5.334253229556999543, 4.956526821568000507 ) ) ;
#33307=CARTESIAN_POINT ( 'NONE',  ( 10.62792628238999981, -3.100579357212000176, 8.599905962393000536 ) ) ;
#33310=EDGE_CURVE ( 'NONE', #873, #38701, #44225, .T. ) ;
#33321=CARTESIAN_POINT ( 'NONE',  ( 10.70780617489000086, -5.157482071823000780, -6.267811103859000532 ) ) ;
#33323=CARTESIAN_POINT ( 'NONE',  ( 6.976556957425999350, -9.209923018478999523, -5.193750594735999648 ) ) ;
#33326=CARTESIAN_POINT ( 'NONE',  ( 8.617943828495366887, -2.919020491875332635, -6.688170526709825481 ) ) ;
#33327=CARTESIAN_POINT ( 'NONE',  ( 8.642077642326000841, -2.899999999999999911, 6.463854830420999953 ) ) ;
#33333=CARTESIAN_POINT ( 'NONE',  ( 10.33240787032999997, -3.158183717747000241, 4.868352313451000057 ) ) ;
#33337=ADVANCED_FACE ( 'NONE', ( #46216 ), #13378, .T. ) ;
#33339=CARTESIAN_POINT ( 'NONE',  ( 11.20904026220999938, -5.937811873294999820, 7.147336919140999001 ) ) ;
#33342=CARTESIAN_POINT ( 'NONE',  ( 10.13050497920000126, -3.092053006542000215, 8.629388195475000245 ) ) ;
#33359=CARTESIAN_POINT ( 'NONE',  ( 7.590045049562995416, -4.176984001086847087, 8.849581831964579592 ) ) ;
#33369=ORIENTED_EDGE ( 'NONE', *, *, #33081, .F. ) ;
#33373=CYLINDRICAL_SURFACE ( 'NONE', #11883, 0.5000000000000002220 ) ;
#33385=CARTESIAN_POINT ( 'NONE',  ( 10.80374194038000013, -2.766944173105999827, -8.073385940268000383 ) ) ;
#33402=CARTESIAN_POINT ( 'NONE',  ( 9.380781717619999682, -2.204246399534000034, 7.545378188773000261 ) ) ;
#33411=CARTESIAN_POINT ( 'NONE',  ( 7.329854050017977407, -3.645852630943380746, 6.184363563554137855 ) ) ;
#33413=CARTESIAN_POINT ( 'NONE',  ( 7.058516392956000196, -4.314043295739000250, 8.819145559946001356 ) ) ;
#33416=CARTESIAN_POINT ( 'NONE',  ( 11.07242469412000041, -6.088279333841999374, 5.193826216086000258 ) ) ;
#33419=CARTESIAN_POINT ( 'NONE',  ( -15.86200481174999943, -2.399999999999999911, 6.571291218949999902 ) ) ;
#33422=B_SPLINE_SURFACE_WITH_KNOTS ( 'NONE', 3, 3, ( 
 ( #8053, #34636, #66776, #45119, #39876, #39176, #30083, #19221, #67112, #29742, #55260, #34286, #39523, #60847, #12962, #55608, #40547, #44780, #28699, #13649, #2123, #12608, #51385, #51045, #7709, #23442, #34977, #13992, #24818, #60499, #35317, #56294, #18892, #8738, #2459 ),
 ( #2801, #3482, #33939, #29395, #8397, #66079, #3146, #24477, #40217, #23783, #66426, #61193, #13314, #50704, #61875, #42530, #5468, #69095, #31357, #42874, #31699, #16640, #32049, #26107, #59287, #67450, #54046, #21883, #15953, #53365, #53021, #11392, #19575, #63496, #64522 ),
 ( #37283, #11059, #64182, #32731, #37967, #48118, #6144, #46144, #5117, #26453, #48464, #40895, #62216, #10704, #58603, #58260, #58952, #26805, #10364, #68741, #27144, #15273, #47786, #222, #47432, #53708, #20858, #43216, #21539, #16296, #37619, #63839, #32393, #5801, #572 ),
 ( #36597, #57923, #10019, #52671, #4765, #42196, #15616, #36946, #21199, #28886, #33078, #22920, #22573, #38312, #59640, #2295, #43916, #65912, #1258, #59983, #11736, #54392, #65220, #6495, #55438, #28531, #33426, #17335, #49844, #12095, #66260, #49492, #18381, #38664, #7531 ) ),
 .UNSPECIFIED., .F., .F., .F.,
 ( 4, 4 ),
 ( 4, 1, 1, 1, 1, 1, 1, 1, 1, 1, 1, 1, 1, 1, 1, 1, 1, 1, 1, 1, 1, 1, 1, 1, 1, 1, 1, 1, 1, 1, 1, 1, 4 ),
 ( -0.1039086239011999951, 1.103908623900999864 ),
 ( -0.02000000000000000042, 0.01250000000000000069, 0.04499999999999999833, 0.07749999999999999944, 0.1100000000000000006, 0.1424999999999999878, 0.1749999999999999889, 0.2074999999999999900, 0.2399999999999999911, 0.2725000000000000200, 0.3049999999999999933, 0.3375000000000000222, 0.3699999999999999956, 0.4025000000000000244, 0.4349999999999999978, 0.4675000000000000266, 0.5000000000000000000, 0.5324999999999999734, 0.5649999999999999467, 0.5975000000000000311, 0.6300000000000000044, 0.6624999999999999778, 0.6949999999999999512, 0.7275000000000000355, 0.7600000000000000089, 0.7924999999999999822, 0.8249999999999999556, 0.8575000000000000400, 0.8900000000000000133, 0.9224999999999999867, 0.9549999999999999600, 0.9875000000000000444, 1.020000000000000018 ),
 .UNSPECIFIED. ) ;
#33426=CARTESIAN_POINT ( 'NONE',  ( 8.866808059624998961, -2.550589632307000088, 8.854674225901000284 ) ) ;
#33440=ORIENTED_EDGE ( 'NONE', *, *, #57129, .T. ) ;
#33444=CARTESIAN_POINT ( 'NONE',  ( 8.606573840185609114, -4.691422996753022545, 5.902471595303201646 ) ) ;
#33448=CARTESIAN_POINT ( 'NONE',  ( 8.616332388160998335, -5.167567399848000065, -6.822293593032000558 ) ) ;
#33458=CARTESIAN_POINT ( 'NONE',  ( 10.59529221449796665, -2.228646686619264905, -7.375818029046365076 ) ) ;
#33485=CARTESIAN_POINT ( 'NONE',  ( 8.725348536223782148, -2.649439212887072959, 7.500023728975150128 ) ) ;
#33488=CARTESIAN_POINT ( 'NONE',  ( 10.22440803363000050, -5.317414323721999736, -8.272454209812998727 ) ) ;
#33496=CARTESIAN_POINT ( 'NONE',  ( 11.09999999999999964, -2.700000000000000178, -6.461133846875999787 ) ) ;
#33507=CARTESIAN_POINT ( 'NONE',  ( 7.308879440377999970, -4.847802017252000439, 9.065364004483999594 ) ) ;
#33508=CARTESIAN_POINT ( 'NONE',  ( 9.397139116365000433, -4.993413662858000812, -9.088148847710000311 ) ) ;
#33512=ORIENTED_EDGE ( 'NONE', *, *, #20264, .T. ) ;
#33513=DIRECTION ( 'NONE',  ( -1.000000000000000000, 0.000000000000000000, 0.000000000000000000 ) ) ;
#33522=CARTESIAN_POINT ( 'NONE',  ( 9.834153701540001791, -5.173926576843999925, 8.813045240277000758 ) ) ;
#33527=CARTESIAN_POINT ( 'NONE',  ( 10.59956814679000026, -4.438148200474000937, -8.958389257466000899 ) ) ;
#33528=CARTESIAN_POINT ( 'NONE',  ( 7.677856441088493078, -5.680960098108038814, 7.021194307766620568 ) ) ;
#33529=CARTESIAN_POINT ( 'NONE',  ( 9.380781717619999682, -2.204246399534000034, 7.545378188773000261 ) ) ;
#33535=ORIENTED_EDGE ( 'NONE', *, *, #33310, .T. ) ;
#33545=CARTESIAN_POINT ( 'NONE',  ( 7.000000000000000000, -9.186881099820000784, 5.186879182879000183 ) ) ;
#33547=FACE_OUTER_BOUND ( 'NONE', #68969, .T. ) ;
#33550=CARTESIAN_POINT ( 'NONE',  ( 10.14163331274965962, -2.604736771093051129, -6.440282737489662956 ) ) ;
#33561=VERTEX_POINT ( 'NONE', #37777 ) ;
#33568=AXIS2_PLACEMENT_3D ( 'NONE', #2941, #46975, #47664 ) ;
#33570=DIRECTION ( 'NONE',  ( 1.000000000000000000, 0.000000000000000000, 0.000000000000000000 ) ) ;
#33572=CARTESIAN_POINT ( 'NONE',  ( 10.43464903646999886, -8.245890014837998550, -6.615317941358999754 ) ) ;
#33579=B_SPLINE_CURVE_WITH_KNOTS ( 'NONE', 3,
 ( #24301, #23271, #28881, #55779 ),
 .UNSPECIFIED., .F., .F.,
 ( 4, 4 ),
 ( 0.000000000000000000, 1.000000000000000000 ),
 .UNSPECIFIED. ) ;
#33588=EDGE_LOOP ( 'NONE', ( #26220, #64721, #56650 ) ) ;
#33609=CONICAL_SURFACE ( 'NONE', #51462, 10.64999999998000035, 0.7853981633972997312 ) ;
#33614=CARTESIAN_POINT ( 'NONE',  ( 10.81746213571000048, -5.100000000000000533, 6.571291218949999902 ) ) ;
#33620=EDGE_CURVE ( 'NONE', #28572, #30733, #49330, .T. ) ;
#33622=CARTESIAN_POINT ( 'NONE',  ( 10.90000000164000049, -2.899999999992999733, 5.160242739040000082 ) ) ;
#33623=CARTESIAN_POINT ( 'NONE',  ( 10.48598064679000075, -5.506038521567000465, -7.274786670944999756 ) ) ;
#33632=B_SPLINE_CURVE_WITH_KNOTS ( 'NONE', 3,
 ( #60358, #66284, #33800, #7220, #6867, #28557, #60702, #7913, #28914, #12819, #49868, #7560, #1982, #23304, #44644, #39381, #34145, #50219, #18408, #56490, #57863, #20114, #20802, #68684, #4019, #51248 ),
 .UNSPECIFIED., .F., .F.,
 ( 4, 2, 2, 2, 2, 2, 2, 2, 2, 2, 2, 2, 4 ),
 ( 0.000000000000000000, 0.08792262688039514940, 0.1758452537607902988, 0.2198065672009883176, 0.2417872239210860641, 0.2527775522811350761, 0.2637678806411841159, 0.3516905075215719378, 0.4396131344019597598, 0.4835744478421525883, 0.5055551045622493911, 0.5275357612823460274, 0.7033810150431129005 ),
 .UNSPECIFIED. ) ;
#33638=CARTESIAN_POINT ( 'NONE',  ( 7.774523880555999966, -9.023795782617998640, 5.558109039331999846 ) ) ;
#33643=CARTESIAN_POINT ( 'NONE',  ( 10.49937632700000023, -2.985311165300999825, -6.358653174814000053 ) ) ;
#33645=CARTESIAN_POINT ( 'NONE',  ( 10.36409408021999923, -3.399999909169000301, -4.954046131279000065 ) ) ;
#33652=CARTESIAN_POINT ( 'NONE',  ( 10.62546583196254879, -2.957832985152635263, 5.049157649731592201 ) ) ;
#33655=CARTESIAN_POINT ( 'NONE',  ( 9.444317341922999987, -2.927260449021000355, 8.897015448164999896 ) ) ;
#33659=ORIENTED_EDGE ( 'NONE', *, *, #43881, .F. ) ;
#33667=CARTESIAN_POINT ( 'NONE',  ( 8.378939856114634210, -5.131721215521674040, 6.760536705178638250 ) ) ;
#33668=CARTESIAN_POINT ( 'NONE',  ( 10.07930721860999945, -2.718124813223000036, -6.397797539448999871 ) ) ;
#33671=FACE_OUTER_BOUND ( 'NONE', #21911, .T. ) ;
#33673=CARTESIAN_POINT ( 'NONE',  ( 9.216140818749000374, -4.008306780893000187, -8.877926425468999128 ) ) ;
#33684=CARTESIAN_POINT ( 'NONE',  ( 10.65050275296000137, -5.200029647236999786, 5.937716681140000397 ) ) ;
#33687=CARTESIAN_POINT ( 'NONE',  ( 9.972852379787999766, -5.044471434015000533, 6.258101649750000384 ) ) ;
#33690=UNCERTAINTY_MEASURE_WITH_UNIT (LENGTH_MEASURE( 1.000000000000000082E-05 ), #59323, 'distance_accuracy_value', 'NONE');
#33703=CARTESIAN_POINT ( 'NONE',  ( 9.136057238048000073, -5.084840204920000772, -6.477689566282000655 ) ) ;
#33712=VERTEX_POINT ( 'NONE', #59102 ) ;
#33721=CARTESIAN_POINT ( 'NONE',  ( 9.365000000002998704, -2.649999999999999911, -7.500000000000000000 ) ) ;
#33729=VERTEX_POINT ( 'NONE', #21690 ) ;
#33730=EDGE_CURVE ( 'NONE', #26679, #852, #32442, .T. ) ;
#33740=B_SPLINE_CURVE_WITH_KNOTS ( 'NONE', 3,
 ( #46089, #18841, #2071, #40838 ),
 .UNSPECIFIED., .F., .F.,
 ( 4, 4 ),
 ( 0.000000000000000000, 0.1253528645472067604 ),
 .UNSPECIFIED. ) ;
#33743=CARTESIAN_POINT ( 'NONE',  ( 9.353559602067283762, -3.378361522263298777, 9.124549040636324548 ) ) ;
#33744=ORIENTED_EDGE ( 'NONE', *, *, #32052, .F. ) ;
#33749=LINE ( 'NONE', #17666, #24796 ) ;
#33753=ORIENTED_EDGE ( 'NONE', *, *, #13383, .T. ) ;
#33759=CARTESIAN_POINT ( 'NONE',  ( 10.37874387220000116, -4.882732524430000609, 6.350796477317000921 ) ) ;
#33761=CARTESIAN_POINT ( 'NONE',  ( 7.935745559623000212, -5.430412429559000387, 7.210798766422999329 ) ) ;
#33764=FACE_OUTER_BOUND ( 'NONE', #58629, .T. ) ;
#33766=AXIS2_PLACEMENT_3D ( 'NONE', #36559, #15581, #8366 ) ;
#33767=CARTESIAN_POINT ( 'NONE',  ( 5.700000000399000122, -0.2999999996014000025, -3.150000003758000044 ) ) ;
#33773=CARTESIAN_POINT ( 'NONE',  ( 11.09999999999999964, -6.593648099371000271, -5.598803483715999896 ) ) ;
#33792=EDGE_CURVE ( 'NONE', #27164, #10252, #43723, .T. ) ;
#33794=CARTESIAN_POINT ( 'NONE',  ( 8.557873356888400451, -3.635451402876086924, 5.799052727755670489 ) ) ;
#33798=CARTESIAN_POINT ( 'NONE',  ( 10.12670810574000058, -3.117521507207000386, 8.613544937223998943 ) ) ;
#33800=CARTESIAN_POINT ( 'NONE',  ( 9.511909979525512426, -4.618059472559051137, 8.703333823275881898 ) ) ;
#33817=ORIENTED_EDGE ( 'NONE', *, *, #62888, .F. ) ;
#33819=ADVANCED_FACE ( 'NONE', ( #54551 ), #27642, .F. ) ;
#33833=CARTESIAN_POINT ( 'NONE',  ( 9.701728707608999969, -4.253751259212999791, -8.839942087209999855 ) ) ;
#33836=LINE ( 'NONE', #34182, #30028 ) ;
#33843=DIRECTION ( 'NONE',  ( 0.000000000000000000, -0.8648648648648717963, 0.5020047465136829867 ) ) ;
#33852=CARTESIAN_POINT ( 'NONE',  ( 7.950754440378000609, -2.095727472214000020, 8.056487497515000484 ) ) ;
#33853=CARTESIAN_POINT ( 'NONE',  ( 9.883740731405000091, -5.634417356902000407, -7.003562403358999156 ) ) ;
#33857=VERTEX_POINT ( 'NONE', #49129 ) ;
#33868=CARTESIAN_POINT ( 'NONE',  ( 11.11504459742000073, -3.456612073675000119, 5.970342812640000218 ) ) ;
#33870=ORIENTED_EDGE ( 'NONE', *, *, #61002, .T. ) ;
#33871=CARTESIAN_POINT ( 'NONE',  ( 8.983146706526143888, -2.899999999999999911, 6.231099004638222638 ) ) ;
#33874=CARTESIAN_POINT ( 'NONE',  ( 10.38725444037999956, -2.888666857901000196, -6.716331201355000502 ) ) ;
#33875=CARTESIAN_POINT ( 'NONE',  ( 7.929910832275415267, -2.314979100831407788, 7.934222329365288040 ) ) ;
#33876=CARTESIAN_POINT ( 'NONE',  ( 9.538434317036999843, -5.620900626097999897, 7.423100105894999245 ) ) ;
#33913=CARTESIAN_POINT ( 'NONE',  ( 10.60113158428419311, -5.349785647438510594, -7.263300972600942984 ) ) ;
#33931=EDGE_CURVE ( 'NONE', #50218, #16743, #44087, .T. ) ;
#33939=CARTESIAN_POINT ( 'NONE',  ( 7.507480646791999668, -3.501517589953999643, 9.055975309745999624 ) ) ;
#33956=CARTESIAN_POINT ( 'NONE',  ( 7.433267076835290865, -2.295947205248204170, 7.848471278922707128 ) ) ;
#33967=CARTESIAN_POINT ( 'NONE',  ( 10.72801694037999987, -3.751276547904999870, -8.836912395451999913 ) ) ;
#33978=EDGE_LOOP ( 'NONE', ( #24447, #58510, #31757, #59965 ) ) ;
#33988=CARTESIAN_POINT ( 'NONE',  ( 9.856713838269000050, -4.814118338972999567, -8.929571672388000536 ) ) ;
#33996=CARTESIAN_POINT ( 'NONE',  ( 10.53432647553000123, -4.980255174632999271, 5.071214337227999636 ) ) ;
#34001=CARTESIAN_POINT ( 'NONE',  ( 10.61382642076999971, -3.385081736013999976, 5.849525238167000651 ) ) ;
#34008=CARTESIAN_POINT ( 'NONE',  ( 5.500000000000000000, -1.300000000000000044, 9.662944685757000940 ) ) ;
#34014=CYLINDRICAL_SURFACE ( 'NONE', #50340, 1.350000000000000089 ) ;
#34021=CARTESIAN_POINT ( 'NONE',  ( 9.837330429757999539, -5.176458967229000230, -8.738385553646999426 ) ) ;
#34029=CARTESIAN_POINT ( 'NONE',  ( 10.41599335357999934, -3.102203969901999869, 5.040281075867000027 ) ) ;
#34035=CARTESIAN_POINT ( 'NONE',  ( 10.46933016578999975, -4.988498232033999891, 6.213103211926000569 ) ) ;
#34038=CARTESIAN_POINT ( 'NONE',  ( 9.476374593785998002, -5.098398394707999159, 6.305533045879999854 ) ) ;
#34050=CARTESIAN_POINT ( 'NONE',  ( 9.260142521132999960, -3.283392111224999965, -8.676955243274001361 ) ) ;
#34053=CARTESIAN_POINT ( 'NONE',  ( 10.02052890782000105, -2.899999999999999911, 6.152188490330000370 ) ) ;
#34064=CARTESIAN_POINT ( 'NONE',  ( 8.930995559624999913, -2.019079883662000086, 7.390983468784999566 ) ) ;
#34068=CARTESIAN_POINT ( 'NONE',  ( 10.52314899745999988, -5.167567567567999731, -6.822293592207000934 ) ) ;
#34073=CARTESIAN_POINT ( 'NONE',  ( 11.06924082387999952, -5.425685649895999774, 8.012912555523998392 ) ) ;
#34074=CYLINDRICAL_SURFACE ( 'NONE', #50739, 1.000000000000000444 ) ;
#34079=CARTESIAN_POINT ( 'NONE',  ( 9.957462135714001406, -5.100000000000000533, -6.571291218949999902 ) ) ;
#34080=VERTEX_POINT ( 'NONE', #12338 ) ;
#34087=CARTESIAN_POINT ( 'NONE',  ( 6.748939170459999914, -9.313044101531000152, -5.427197938553000256 ) ) ;
#34091=CARTESIAN_POINT ( 'NONE',  ( 10.89034309416000035, -5.058758371668000464, -5.035645192038000317 ) ) ;
#34104=ADVANCED_FACE ( 'NONE', ( #33671 ), #54989, .F. ) ;
#34106=FACE_OUTER_BOUND ( 'NONE', #32983, .T. ) ;
#34107=CARTESIAN_POINT ( 'NONE',  ( 8.962745559623000347, -5.445226602819000838, 7.703375344019999460 ) ) ;
#34124=EDGE_CURVE ( 'NONE', #1057, #65964, #28427, .T. ) ;
#34145=CARTESIAN_POINT ( 'NONE',  ( 9.464432710331807996, -5.182476493413302521, 8.153247799998663226 ) ) ;
#34146=CARTESIAN_POINT ( 'NONE',  ( 10.31746213571000048, -5.100000000000000533, 6.571291218949999902 ) ) ;
#34155=VERTEX_POINT ( 'NONE', #23860 ) ;
#34160=B_SPLINE_CURVE_WITH_KNOTS ( 'NONE', 3,
 ( #43400, #60507, #37799, #59122 ),
 .UNSPECIFIED., .F., .F.,
 ( 4, 4 ),
 ( 0.000000000000000000, 1.000000000000000000 ),
 .UNSPECIFIED. ) ;
#34161=EDGE_LOOP ( 'NONE', ( #31382, #50743, #23386, #44707, #26664, #10980, #8806 ) ) ;
#34162=CARTESIAN_POINT ( 'NONE',  ( 10.68864842108893498, -2.651255354521660834, 7.268672825006785132 ) ) ;
#34170=ORIENTED_EDGE ( 'NONE', *, *, #9073, .F. ) ;
#34173=B_SPLINE_CURVE_WITH_KNOTS ( 'NONE', 3,
 ( #32617, #52905, #5003, #26688 ),
 .UNSPECIFIED., .F., .F.,
 ( 4, 4 ),
 ( 0.000000000000000000, 0.1253969396550571880 ),
 .UNSPECIFIED. ) ;
#34178=CARTESIAN_POINT ( 'NONE',  ( 10.34225158793000077, -3.348983461003999906, -8.881464249475000017 ) ) ;
#34182=CARTESIAN_POINT ( 'NONE',  ( 11.09999999999999964, -2.649999999999999911, 7.500000000000000000 ) ) ;
#34184=CARTESIAN_POINT ( 'NONE',  ( 10.16000000000000014, -4.496968146123999865, -8.755198255949000696 ) ) ;
#34185=ADVANCED_FACE ( 'NONE', ( #27738 ), #65810, .F. ) ;
#34188=EDGE_CURVE ( 'NONE', #40775, #61047, #4061, .T. ) ;
#34189=CARTESIAN_POINT ( 'NONE',  ( 10.72963504510672195, -4.176677120266497845, -8.849854844400173448 ) ) ;
#34199=CARTESIAN_POINT ( 'NONE',  ( 9.041941940379999210, -2.707994276285999646, 5.994456121676999594 ) ) ;
#34201=EDGE_CURVE ( 'NONE', #9091, #20205, #54977, .T. ) ;
#34216=CARTESIAN_POINT ( 'NONE',  ( 9.388626433405999450, -4.079401915682999480, 9.259353168384000909 ) ) ;
#34221=CARTESIAN_POINT ( 'NONE',  ( 7.998638406009124679, -2.569044558284087731, 6.497043829224429246 ) ) ;
#34222=CARTESIAN_POINT ( 'NONE',  ( 9.662553763536999796, -4.094830574823999925, 9.119950378356000087 ) ) ;
#34223=CIRCLE ( 'NONE', #63184, 1.000000000000000000 ) ;
#34226=ORIENTED_EDGE ( 'NONE', *, *, #9246, .F. ) ;
#34232=CARTESIAN_POINT ( 'NONE',  ( 9.619730517102000888, -2.477793449086000077, -8.275032865112999403 ) ) ;
#34242=CARTESIAN_POINT ( 'NONE',  ( 8.572269353210000276, -2.606998386752999775, 6.345764833140000505 ) ) ;
#34244=VERTEX_POINT ( 'NONE', #9148 ) ;
#34248=CARTESIAN_POINT ( 'NONE',  ( 10.91060805961999947, -4.702347118766000200, -9.210032991522000501 ) ) ;
#34251=CARTESIAN_POINT ( 'NONE',  ( 8.058915628308609413, -4.678948124125613894, 8.679023822940409971 ) ) ;
#34272=EDGE_CURVE ( 'NONE', #3478, #4443, #52139, .T. ) ;
#34285=CARTESIAN_POINT ( 'NONE',  ( 10.68437022634959099, -5.721797460400984470, 7.171884794389442597 ) ) ;
#34286=CARTESIAN_POINT ( 'NONE',  ( 8.175754440378000254, -2.599231861044000169, 7.909347897884000389 ) ) ;
#34290=ORIENTED_EDGE ( 'NONE', *, *, #68985, .T. ) ;
#34299=CARTESIAN_POINT ( 'NONE',  ( 9.398030179116712901, -5.281061815207925392, 7.060613688865339910 ) ) ;
#34301=ORIENTED_EDGE ( 'NONE', *, *, #30497, .F. ) ;
#34304=CARTESIAN_POINT ( 'NONE',  ( 7.433210666546943735, -2.296204528772303188, 7.849734464718515881 ) ) ;
#34306=CARTESIAN_POINT ( 'NONE',  ( 10.55880524124688158, -4.703942329536042521, 8.703471051125557523 ) ) ;
#34310=FACE_OUTER_BOUND ( 'NONE', #16173, .T. ) ;
#34315=CARTESIAN_POINT ( 'NONE',  ( 11.37167944038000122, -2.803484087760999888, -6.967877228197000505 ) ) ;
#34316=AXIS2_PLACEMENT_3D ( 'NONE', #45364, #2705, #22643 ) ;
#34329=CARTESIAN_POINT ( 'NONE',  ( 8.949577224479325466, -5.282137943145613690, 7.064064936788390980 ) ) ;
#34332=CARTESIAN_POINT ( 'NONE',  ( 6.953073139469000630, -9.233001678504999532, 5.200628701625999994 ) ) ;
#34336=FACE_OUTER_BOUND ( 'NONE', #12440, .T. ) ;
#34340=CARTESIAN_POINT ( 'NONE',  ( 10.55068143582000140, -2.412180768165999911, -6.919582641217999708 ) ) ;
#34347=CARTESIAN_POINT ( 'NONE',  ( 11.09689463776999929, -5.238465444143000305, 5.055407489333999749 ) ) ;
#34351=CARTESIAN_POINT ( 'NONE',  ( 10.50244460374000077, -2.268915328469999881, 7.824865002012999504 ) ) ;
#34353=CARTESIAN_POINT ( 'NONE',  ( 10.81746213571000048, -5.100000000000000533, 6.571291218949999902 ) ) ;
#34360=CARTESIAN_POINT ( 'NONE',  ( 10.97843137008999825, -5.235400103863000254, 6.782920672145000829 ) ) ;
#34369=CARTESIAN_POINT ( 'NONE',  ( 9.101385834542000453, -4.783349162191000481, -6.231236652334000148 ) ) ;
#34375=CARTESIAN_POINT ( 'NONE',  ( 10.27678977068999977, -3.259542233426000024, 4.694017977725000179 ) ) ;
#34381=CARTESIAN_POINT ( 'NONE',  ( 9.104016254283999743, -5.045864843302999780, 8.527867871227000407 ) ) ;
#34385=CARTESIAN_POINT ( 'NONE',  ( 9.696086916451999826, -2.554404004330999900, 7.600685922079000179 ) ) ;
#34398=CARTESIAN_POINT ( 'NONE',  ( 9.746744136172999617, -5.062748727288000516, -8.618689820632001286 ) ) ;
#34400=VERTEX_POINT ( 'NONE', #8128 ) ;
#34417=ADVANCED_FACE ( 'NONE', ( #50783 ), #25921, .F. ) ;
#34418=CARTESIAN_POINT ( 'NONE',  ( 11.09999999999999964, -2.660544054589125462, -8.447007675617404843 ) ) ;
#34426=CARTESIAN_POINT ( 'NONE',  ( 10.25462442569999943, -2.860634389522000109, 6.604605425112000994 ) ) ;
#34429=ORIENTED_EDGE ( 'NONE', *, *, #870, .T. ) ;
#34440=CARTESIAN_POINT ( 'NONE',  ( 9.379272429982512094, -2.901493056294750073, 8.849497897647601974 ) ) ;
#34444=CARTESIAN_POINT ( 'NONE',  ( 11.04423059897000137, -5.244779299905999892, -5.172774331138000115 ) ) ;
#34448=CARTESIAN_POINT ( 'NONE',  ( 11.02786767503999954, -5.596230239120999705, 7.209501483790000442 ) ) ;
#34451=ORIENTED_EDGE ( 'NONE', *, *, #27354, .F. ) ;
#34458=CARTESIAN_POINT ( 'NONE',  ( 7.422245559621999611, -5.361050935357000391, 6.973449182446000094 ) ) ;
#34461=CARTESIAN_POINT ( 'NONE',  ( 11.12486982654999856, -5.426806274205000058, 5.164827877695000069 ) ) ;
#34466=AXIS2_PLACEMENT_3D ( 'NONE', #28239, #50253, #23679 ) ;
#34476=CARTESIAN_POINT ( 'NONE',  ( 8.057193283769001013, -5.122325659685000865, 6.732791538586998747 ) ) ;
#34479=CARTESIAN_POINT ( 'NONE',  ( 8.590472024761121261, -4.653241489316459756, 5.916299078424147595 ) ) ;
#34481=ORIENTED_EDGE ( 'NONE', *, *, #42574, .T. ) ;
#34485=CARTESIAN_POINT ( 'NONE',  ( 7.807587516710824183, -3.023362854828683499, 6.518709396491844110 ) ) ;
#34492=CARTESIAN_POINT ( 'NONE',  ( 9.516209514376292589, -2.899999999999999911, -6.465979581418092259 ) ) ;
#34500=CARTESIAN_POINT ( 'NONE',  ( 8.881816940380000247, -4.977917894183000236, 6.416767031887000705 ) ) ;
#34507=CARTESIAN_POINT ( 'NONE',  ( 5.600000001140999828, 0.000000000000000000, -1.349999998858999906 ) ) ;
#34508=EDGE_CURVE ( 'NONE', #26111, #66341, #56587, .T. ) ;
#34516=CARTESIAN_POINT ( 'NONE',  ( 9.629471092178999214, -5.100000000000000533, 6.152188490330000370 ) ) ;
#34527=ORIENTED_EDGE ( 'NONE', *, *, #42613, .T. ) ;
#34532=CARTESIAN_POINT ( 'NONE',  ( 10.78636854442000192, -5.666037955714999796, -7.787004779180999314 ) ) ;
#34549=CARTESIAN_POINT ( 'NONE',  ( 7.000000000000000000, -7.526486366024999874, 3.526486366024999874 ) ) ;
#34552=ORIENTED_EDGE ( 'NONE', *, *, #52393, .T. ) ;
#34553=CARTESIAN_POINT ( 'NONE',  ( 8.373668146795001377, -2.202816532622999812, 7.706987678916999762 ) ) ;
#34566=CARTESIAN_POINT ( 'NONE',  ( 9.854949224988001077, -2.800315695760000168, 9.013807298610000629 ) ) ;
#34570=CARTESIAN_POINT ( 'NONE',  ( 11.03091694037999915, -5.020463882420000523, -6.601194361798000010 ) ) ;
#34571=CARTESIAN_POINT ( 'NONE',  ( 7.899652377730045139, -2.585612559568443380, 8.512102292667707459 ) ) ;
#34572=CARTESIAN_POINT ( 'NONE',  ( 9.034116535116000435, -4.695350938297000454, 8.660677768253002284 ) ) ;
#34581=CARTESIAN_POINT ( 'NONE',  ( 9.886323620223000930, -4.261100936929000049, -5.979198511086000423 ) ) ;
#34586=EDGE_CURVE ( 'NONE', #22584, #68990, #6655, .T. ) ;
#34590=ORIENTED_EDGE ( 'NONE', *, *, #30618, .F. ) ;
#34594=CARTESIAN_POINT ( 'NONE',  ( 8.149355646792999508, -2.583664704444999849, 6.684748541034000624 ) ) ;
#34600=CARTESIAN_POINT ( 'NONE',  ( 11.19050685320999960, -2.516759970060999940, -6.840363309917000478 ) ) ;
#34612=CYLINDRICAL_SURFACE ( 'NONE', #39201, 0.4999999999999998335 ) ;
#34621=VERTEX_POINT ( 'NONE', #21278 ) ;
#34635=CARTESIAN_POINT ( 'NONE',  ( 10.81249950090998269, -4.268769985470544093, 9.219235902382948211 ) ) ;
#34636=CARTESIAN_POINT ( 'NONE',  ( 7.555275273711000494, -4.314043295739000250, 8.819145559946001356 ) ) ;
#34646=FACE_OUTER_BOUND ( 'NONE', #23397, .T. ) ;
#34647=CARTESIAN_POINT ( 'NONE',  ( 7.000000000000000000, -1.065814103639999922E-14, 1.505462421391999793E-13 ) ) ;
#34660=DIRECTION ( 'NONE',  ( -0.8660254037844289376, 0.000000000000000000, 0.5000000000000169864 ) ) ;
#34664=CARTESIAN_POINT ( 'NONE',  ( 10.27366694038000006, -3.065543393453000309, -8.487918777453998587 ) ) ;
#34671=ORIENTED_EDGE ( 'NONE', *, *, #21002, .F. ) ;
#34679=CARTESIAN_POINT ( 'NONE',  ( 9.721802827886667941, -2.874603711572091935, 6.749639981085449492 ) ) ;
#34682=LINE ( 'NONE', #32345, #1861 ) ;
#34683=CARTESIAN_POINT ( 'NONE',  ( 10.53733998880999856, -2.992814141720000265, 8.731692578598000409 ) ) ;
#34687=CARTESIAN_POINT ( 'NONE',  ( 10.70846056750539788, -2.938500698085303675, -5.066367099627377080 ) ) ;
#34694=DIRECTION ( 'NONE',  ( 0.000000000000000000, -0.9928377162714321358, 0.1194707878476041485 ) ) ;
#34697=CARTESIAN_POINT ( 'NONE',  ( 10.00122642709000154, -2.274091010763000131, 7.851325450887000734 ) ) ;
#34711=CARTESIAN_POINT ( 'NONE',  ( 9.573320215454998561, -2.624754973437999794, -6.486841649805000110 ) ) ;
#34718=CARTESIAN_POINT ( 'NONE',  ( 10.28638091290000034, -3.298456390694000095, 5.006422727232999748 ) ) ;
#34719=DIRECTION ( 'NONE',  ( 0.000000000000000000, 0.000000000000000000, -1.000000000000000000 ) ) ;
#34723=CARTESIAN_POINT ( 'NONE',  ( 10.55991645936999923, -5.094263939633999705, 6.075409946530999861 ) ) ;
#34727=CARTESIAN_POINT ( 'NONE',  ( 10.37874387220000116, -4.882732524430000609, 6.350796477317000921 ) ) ;
#34733=CARTESIAN_POINT ( 'NONE',  ( 8.839582747487000347, -3.464784534403999139, -6.238107624440003107 ) ) ;
#34737=CARTESIAN_POINT ( 'NONE',  ( 9.957251191599000961, -4.686746084135999801, -9.174865097765998456 ) ) ;
#34749=ORIENTED_EDGE ( 'NONE', *, *, #39534, .T. ) ;
#34757=CARTESIAN_POINT ( 'NONE',  ( 11.09999999999999964, -3.166318547749471080, -8.857024312923449827 ) ) ;
#34777=CYLINDRICAL_SURFACE ( 'NONE', #16775, 0.5000000000000002220 ) ;
#34778=CARTESIAN_POINT ( 'NONE',  ( 9.363635060566240398, -3.176852285862109770, 9.044600143522814051 ) ) ;
#34785=CARTESIAN_POINT ( 'NONE',  ( 10.43579701286999928, -2.587605342384000195, 6.390039770907999461 ) ) ;
#34793=DIRECTION ( 'NONE',  ( -0.7071067811865475727, 0.7071067811865475727, 0.000000000000000000 ) ) ;
#34797=CARTESIAN_POINT ( 'NONE',  ( 11.02039621389999979, -6.423930830464999353, 5.275616672426000520 ) ) ;
#34798=CARTESIAN_POINT ( 'NONE',  ( 8.393929141338995592, -5.090180864267003003, -6.637945330154001233 ) ) ;
#34808=CARTESIAN_POINT ( 'NONE',  ( 10.96882000591000050, -5.145193212282999973, 5.031654701678999864 ) ) ;
#34821=CARTESIAN_POINT ( 'NONE',  ( 11.08757144985999865, -2.712428550139000194, 6.571291218949999902 ) ) ;
#34823=DIRECTION ( 'NONE',  ( 0.000000000000000000, -0.8646938284590766077, 0.5022992962614868384 ) ) ;
#34832=CARTESIAN_POINT ( 'NONE',  ( 9.479212726990999371, -4.071727350623000063, 9.089303488377000306 ) ) ;
#34835=CARTESIAN_POINT ( 'NONE',  ( 8.175754440378000254, -2.599231861044000169, 7.909347897884000389 ) ) ;
#34850=CARTESIAN_POINT ( 'NONE',  ( 10.47094409420000005, -5.100000000000000533, 6.571291218949999902 ) ) ;
#34855=CARTESIAN_POINT ( 'NONE',  ( 6.799999045260999964, -9.295457794069999835, 5.399713664196000629 ) ) ;
#34864=CARTESIAN_POINT ( 'NONE',  ( 10.58996262057999971, -2.876743158681999812, -6.236533224899999617 ) ) ;
#34866=CARTESIAN_POINT ( 'NONE',  ( 9.652022804587478078, -2.759070395092175332, -6.267057333003529074 ) ) ;
#34869=EDGE_LOOP ( 'NONE', ( #24529, #65822, #62433, #68636, #2916, #21752, #42492, #30453, #62412, #1133, #9541, #28837, #60869, #21993, #39716, #38271, #10771 ) ) ;
#34886=ORIENTED_EDGE ( 'NONE', *, *, #14369, .T. ) ;
#34887=CARTESIAN_POINT ( 'NONE',  ( 7.731793146792000471, -4.580607464247000493, 9.213361409141999303 ) ) ;
#34893=B_SPLINE_CURVE_WITH_KNOTS ( 'NONE', 3,
 ( #55421, #45281, #24637, #56449 ),
 .UNSPECIFIED., .F., .F.,
 ( 4, 4 ),
 ( 0.8746828543526545818, 1.000000000000000000 ),
 .UNSPECIFIED. ) ;
#34895=CARTESIAN_POINT ( 'NONE',  ( 10.90453766415000025, -2.900310535872000273, -5.130381900875999435 ) ) ;
#34902=CARTESIAN_POINT ( 'NONE',  ( 9.889844610056000462, -4.052276314598000084, 9.260527932809999641 ) ) ;
#34907=CARTESIAN_POINT ( 'NONE',  ( 10.06949314679000018, -4.910373174915999783, -8.649593977693999847 ) ) ;
#34908=B_SPLINE_CURVE_WITH_KNOTS ( 'NONE', 3,
 ( #24968, #23339, #44682, #65974, #18102, #34184 ),
 .UNSPECIFIED., .F., .F.,
 ( 4, 2, 4 ),
 ( 0.3058164706682733325, 0.6529082353341366662, 1.000000000000000000 ),
 .UNSPECIFIED. ) ;
#34909=CARTESIAN_POINT ( 'NONE',  ( 8.053293077950769430, -3.529150488797779595, 5.824254571415059978 ) ) ;
#34910=CARTESIAN_POINT ( 'NONE',  ( 10.84168850528999961, -2.681008214828000114, 6.554752254946000889 ) ) ;
#34915=CARTESIAN_POINT ( 'NONE',  ( 10.32891567890999873, -4.769919575850000371, -4.571345007831999929 ) ) ;
#34917=ORIENTED_EDGE ( 'NONE', *, *, #50752, .F. ) ;
#34920=CARTESIAN_POINT ( 'NONE',  ( 9.754318513071000396, -2.462132291381999849, -7.373611177161000008 ) ) ;
#34930=CIRCLE ( 'NONE', #27083, 1.300000000000000044 ) ;
#34931=CARTESIAN_POINT ( 'NONE',  ( 8.058769353207999586, -2.432121990576000314, 6.597519606637999523 ) ) ;
#34933=EDGE_LOOP ( 'NONE', ( #68375, #12248, #41453, #43215, #46347, #36149, #10040, #56557 ) ) ;
#34937=CARTESIAN_POINT ( 'NONE',  ( 10.67529314679000052, -3.066674550532999977, -8.703235919197002346 ) ) ;
#34943=EDGE_CURVE ( 'NONE', #21223, #36042, #39076, .T. ) ;
#34949=( NAMED_UNIT ( * ) PLANE_ANGLE_UNIT ( ) SI_UNIT ( $, .RADIAN. ) );
#34958=CARTESIAN_POINT ( 'NONE',  ( 10.26088874563355091, -3.646602187523998673, -8.814783671671618137 ) ) ;
#34964=B_SPLINE_SURFACE_WITH_KNOTS ( 'NONE', 3, 3, ( 
 ( #55913, #27965, #1730, #23049, #60463, #39486, #34248, #65699, #64993, #38443, #33207, #6627, #54872, #66389, #59766, #2086, #7318, #11867, #18164, #17822, #60809, #39136, #50322, #7668, #29015, #2420, #12225, #49275, #6974, #18512, #54525, #39834, #61156, #44046, #13273 ),
 ( #34600, #65351, #61834, #25118, #24092, #50665, #68096, #8702, #10666, #56252, #62173, #51006, #67072, #25458, #2766, #9033, #40508, #18853, #30045, #29705, #9365, #30711, #13953, #14969, #45425, #61496, #36292, #46790, #35279, #66734, #19185, #40180, #46104, #52021, #8359 ),
 ( #14296, #13614, #35624, #24777, #67749, #24438, #3106, #20213, #35951, #62514, #41539, #51348, #56937, #4122, #19874, #57612, #62851, #34937, #45764, #56595, #3440, #67410, #19534, #40853, #30374, #51682, #3780, #46450, #41204, #14633, #57265, #17293, #21841, #11016, #6105 ),
 ( #65176, #1218, #38975, #65524, #32013, #38620, #17652, #53327, #59941, #64479, #5427, #42832, #12052, #48077, #60293, #26767, #33385, #54701, #32689, #11695, #181, #16256, #37579, #37927, #59596, #21498, #54003, #38270, #64141, #58913, #22191, #33035, #16937, #59246, #54347 ) ),
 .UNSPECIFIED., .F., .F., .F.,
 ( 4, 4 ),
 ( 4, 1, 1, 1, 1, 1, 1, 1, 1, 1, 1, 1, 1, 1, 1, 1, 1, 1, 1, 1, 1, 1, 1, 1, 1, 1, 1, 1, 1, 1, 1, 1, 4 ),
 ( -0.1039086239011999951, 1.103908623900999864 ),
 ( 0.2233333333344000027, 0.2480800653604999795, 0.2728267973865999840, 0.2975735294126999886, 0.3223202614387999931, 0.3470669934649999733, 0.3718137254910999778, 0.3965604575171999824, 0.4213071895433000424, 0.4460539215694000470, 0.4708006535954999960, 0.4955473856216000006, 0.5202941176476999496, 0.5450408496738000652, 0.5697875816999000698, 0.5945343137260000743, 0.6192810457521999989, 0.6440277777783000035, 0.6687745098044000081, 0.6935212418305000126, 0.7182679738566000172, 0.7430147058827000217, 0.7677614379088000263, 0.7925081699349000308, 0.8172549019609999243, 0.8420016339870999289, 0.8667483660132000445, 0.8914950980394000801, 0.9162418300655000847, 0.9409885620915999782, 0.9657352941176999828, 0.9904820261437999873, 1.015228758169999912 ),
 .UNSPECIFIED. ) ;
#34976=CARTESIAN_POINT ( 'NONE',  ( 10.89729545638381403, -2.607631909929567282, 8.596128993616638070 ) ) ;
#34977=CARTESIAN_POINT ( 'NONE',  ( 9.138566940380000503, -2.933824946949000090, 8.496487880080000110 ) ) ;
#34987=DIRECTION ( 'NONE',  ( 0.8480635683784220058, 0.000000000000000000, -0.5298945026977139872 ) ) ;
#34992=CARTESIAN_POINT ( 'NONE',  ( 8.977754440379998258, -2.019079883662000086, 7.390983468784999566 ) ) ;
#34995=EDGE_CURVE ( 'NONE', #32140, #40775, #40801, .T. ) ;
#34997=CARTESIAN_POINT ( 'NONE',  ( 7.428154886651814337, -2.321820467422959666, 7.962693524187518079 ) ) ;
#35003=CARTESIAN_POINT ( 'NONE',  ( 11.09999999999999964, -2.274006712557999688, -7.281956340829000673 ) ) ;
#35008=CARTESIAN_POINT ( 'NONE',  ( 10.99305444037999990, -4.495427106425000652, -6.233607450113000326 ) ) ;
#35024=CARTESIAN_POINT ( 'NONE',  ( 11.00000000000000000, -2.799999999999999822, 5.865766984179000332 ) ) ;
#35026=CARTESIAN_POINT ( 'NONE',  ( 10.40516264833000015, -5.216401621862000404, 6.765753642936999768 ) ) ;
#35029=CARTESIAN_POINT ( 'NONE',  ( 10.64126772939999910, -2.258710642251000156, -6.863482599505999815 ) ) ;
#35031=DIRECTION ( 'NONE',  ( 1.000000000000000000, 0.000000000000000000, 0.000000000000000000 ) ) ;
#35034=CARTESIAN_POINT ( 'NONE',  ( 10.96866170142999941, -6.476647493854999382, -5.207916108537000710 ) ) ;
#35040=CARTESIAN_POINT ( 'NONE',  ( 9.500008250440000523, -2.279684233303000074, 7.877691491255999878 ) ) ;
#35047=B_SPLINE_CURVE_WITH_KNOTS ( 'NONE', 3,
 ( #6131, #22904, #54728, #59626 ),
 .UNSPECIFIED., .F., .F.,
 ( 4, 4 ),
 ( 0.000000000000000000, 1.000000000000000000 ),
 .UNSPECIFIED. ) ;
#35050=CARTESIAN_POINT ( 'NONE',  ( 8.933148997457999840, -5.167567567567999731, 6.822293592207000934 ) ) ;
#35054=CARTESIAN_POINT ( 'NONE',  ( 9.776078604427999252, -4.565692099013000771, -8.879633571423999783 ) ) ;
#35059=EDGE_CURVE ( 'NONE', #13225, #29696, #64060, .T. ) ;
#35068=CARTESIAN_POINT ( 'NONE',  ( 10.03491210303999992, -5.615910465798999773, 7.351455544018000943 ) ) ;
#35075=EDGE_CURVE ( 'NONE', #44229, #7255, #26574, .T. ) ;
#35076=AXIS2_PLACEMENT_3D ( 'NONE', #12816, #50217, #28555 ) ;
#35083=DIRECTION ( 'NONE',  ( 0.7071067811865475727, 0.7071067811865475727, 0.000000000000000000 ) ) ;
#35086=CARTESIAN_POINT ( 'NONE',  ( 9.348145925901000908, -2.626678530444999993, -7.387134320497999340 ) ) ;
#35104=CARTESIAN_POINT ( 'NONE',  ( 11.09999999999999964, -3.512324525112999751, -8.971282648301999174 ) ) ;
#35122=CARTESIAN_POINT ( 'NONE',  ( 9.501882463939899992, -2.610834736344150642, 6.433711780408752468 ) ) ;
#35125=CARTESIAN_POINT ( 'NONE',  ( 9.838376522720714945, -5.764887630754955694, -7.468471882345152579 ) ) ;
#35126=CARTESIAN_POINT ( 'NONE',  ( 10.95934799724999920, -5.155594434375000645, -5.120697376301999171 ) ) ;
#35129=CARTESIAN_POINT ( 'NONE',  ( 9.166075977534999808, -4.023333687735000552, 9.122281080215000060 ) ) ;
#35145=CARTESIAN_POINT ( 'NONE',  ( 8.853612782865001307, -4.539814389745004952, -6.225821853175999010 ) ) ;
#35148=CARTESIAN_POINT ( 'NONE',  ( 8.199995110659001440, -2.894508759333000114, 6.645190873281999089 ) ) ;
#35149=CARTESIAN_POINT ( 'NONE',  ( 9.976909913808000852, -4.233164088428999605, -6.141918726850000176 ) ) ;
#35155=AXIS2_PLACEMENT_3D ( 'NONE', #41178, #25091, #36617 ) ;
#35164=CARTESIAN_POINT ( 'NONE',  ( 7.808061958594711527, -3.029385392905544538, 6.512745199459435419 ) ) ;
#35175=CARTESIAN_POINT ( 'NONE',  ( 10.34947173981000113, -4.457565973839000328, 6.154866550070000386 ) ) ;
#35178=CARTESIAN_POINT ( 'NONE',  ( 8.432504440379000599, -5.430412429559000387, 7.210798766422999329 ) ) ;
#35188=CARTESIAN_POINT ( 'NONE',  ( 10.96080136920999948, -2.054580854576999904, 7.810082699133999995 ) ) ;
#35192=FACE_OUTER_BOUND ( 'NONE', #28370, .T. ) ;
#35198=CARTESIAN_POINT ( 'NONE',  ( 10.92360823440131590, -2.830160228212987850, -6.777088824845431958 ) ) ;
#35203=EDGE_CURVE ( 'NONE', #29696, #606, #53314, .T. ) ;
#35213=CARTESIAN_POINT ( 'NONE',  ( 9.882901294779998125, -4.314558311729999929, -9.161035779983999205 ) ) ;
#35214=LINE ( 'NONE', #20151, #5986 ) ;
#35223=CARTESIAN_POINT ( 'NONE',  ( -15.86200481174999943, -2.399999999999999911, 6.571291218949999902 ) ) ;
#35232=ORIENTED_EDGE ( 'NONE', *, *, #47132, .T. ) ;
#35233=CARTESIAN_POINT ( 'NONE',  ( 8.668206853210000062, -3.979464503892999439, 9.134080454305001595 ) ) ;
#35235=CARTESIAN_POINT ( 'NONE',  ( 7.744301838472999577, -3.130384865731000055, 6.467396727560999814 ) ) ;
#35243=EDGE_LOOP ( 'NONE', ( #69067, #47100, #48867, #36842, #44564, #58607, #47995, #19416 ) ) ;
#35245=CARTESIAN_POINT ( 'NONE',  ( 9.437500199782947519, -5.100000000000000533, -6.523154174498921876 ) ) ;
#35247=CARTESIAN_POINT ( 'NONE',  ( 7.936333720142999759, -5.123034382927999175, 6.721303993095999907 ) ) ;
#35251=CARTESIAN_POINT ( 'NONE',  ( 11.25809194037999994, -3.275508415657999883, -8.650784343212000849 ) ) ;
#35252=CARTESIAN_POINT ( 'NONE',  ( 8.071816895048858242, -3.937760767473150292, 5.761230312822644528 ) ) ;
#35263=CARTESIAN_POINT ( 'NONE',  ( 9.399722005181999407, -5.700621988293000264, -7.339579610785999186 ) ) ;
#35264=DIRECTION ( 'NONE',  ( 1.000000000000000000, 0.000000000000000000, 0.000000000000000000 ) ) ;
#35270=ORIENTED_EDGE ( 'NONE', *, *, #45724, .T. ) ;
#35273=CARTESIAN_POINT ( 'NONE',  ( 7.635855646791999796, -2.466384407480000096, 6.935560677555000275 ) ) ;
#35279=CARTESIAN_POINT ( 'NONE',  ( 10.16821935321000048, -2.330398934821000356, -7.267462182607999921 ) ) ;
#35288=ADVANCED_FACE ( 'NONE', ( #16128 ), #21371, .F. ) ;
#35300=CARTESIAN_POINT ( 'NONE',  ( 10.19837725605996326, -4.679950664087114909, -8.679651447173698742 ) ) ;
#35313=ORIENTED_EDGE ( 'NONE', *, *, #62693, .T. ) ;
#35316=CARTESIAN_POINT ( 'NONE',  ( 10.81004357109428327, -4.321142019900527487, 9.210264094307881066 ) ) ;
#35317=CARTESIAN_POINT ( 'NONE',  ( 9.395316940379000670, -5.146736128384000075, 6.597417125647000447 ) ) ;
#35328=CARTESIAN_POINT ( 'NONE',  ( 6.999999999999999112, -7.162151381622562596, 3.226150686063063322 ) ) ;
#35335=CARTESIAN_POINT ( 'NONE',  ( 7.539230646792000279, -4.696237245142999228, 5.830277424166999900 ) ) ;
#35339=CARTESIAN_POINT ( 'NONE',  ( 7.450492827224381109, -2.261080942162393637, 7.469285780581691903 ) ) ;
#35340=CARTESIAN_POINT ( 'NONE',  ( 10.67320712187270004, -2.921171224854953063, 8.329102901498991685 ) ) ;
#35345=CARTESIAN_POINT ( 'NONE',  ( 10.94841903626084090, -4.366312240206965178, -9.227246227427363223 ) ) ;
#35348=CARTESIAN_POINT ( 'NONE',  ( 10.69015444038000062, -4.391267940138999570, -8.802346922965000431 ) ) ;
#35351=CARTESIAN_POINT ( 'NONE',  ( 10.97581817698185525, -5.215421929002181933, 6.751285922363551073 ) ) ;
#35365=CARTESIAN_POINT ( 'NONE',  ( 10.68361719090999884, -2.603550124652000086, 7.762065570229999878 ) ) ;
#35394=CARTESIAN_POINT ( 'NONE',  ( 9.282558421712998609, -4.950980172046000050, -5.959730545597000884 ) ) ;
#35405=VECTOR ( 'NONE', #44914, 1000.000000000000000 ) ;
#35406=CARTESIAN_POINT ( 'NONE',  ( 9.538434317036999843, -5.620900626097999897, 7.423100105894999245 ) ) ;
#35412=CARTESIAN_POINT ( 'NONE',  ( 10.17284693385893490, -4.293232846717661033, -8.835933254752704968 ) ) ;
#35422=AXIS2_PLACEMENT_3D ( 'NONE', #49882, #65946, #65607 ) ;
#35423=CARTESIAN_POINT ( 'NONE',  ( 9.436149330669000079, -3.485164486501000081, -6.221839249167999242 ) ) ;
#35425=EDGE_LOOP ( 'NONE', ( #64848, #31826, #17864, #57324, #66004, #60638, #10243, #47016 ) ) ;
#35434=CARTESIAN_POINT ( 'NONE',  ( 9.167129859538265535, -5.079276359681585973, -8.329393289878948892 ) ) ;
#35445=CARTESIAN_POINT ( 'NONE',  ( 8.654403730149667240, -2.899999999999999911, 6.499666959930667787 ) ) ;
#35461=CARTESIAN_POINT ( 'NONE',  ( 9.089766096192999356, -8.660638521191998507, -6.051256224376999171 ) ) ;
#35466=CARTESIAN_POINT ( 'NONE',  ( 8.122851870745966707, -2.921728982776596872, 8.328193042681078850 ) ) ;
#35473=B_SPLINE_CURVE_WITH_KNOTS ( 'NONE', 3,
 ( #53050, #3181, #24509, #69121, #21566, #63867 ),
 .UNSPECIFIED., .F., .F.,
 ( 4, 2, 4 ),
 ( 0.000000000000000000, 0.5000000000000000000, 1.000000000000000000 ),
 .UNSPECIFIED. ) ;
#35488=CARTESIAN_POINT ( 'NONE',  ( 10.60811446581000084, -2.866936631589000140, -4.836298645267000929 ) ) ;
#35489=CARTESIAN_POINT ( 'NONE',  ( 9.930325322607000516, -5.020908168068000776, -6.342951604057000203 ) ) ;
#35490=DIRECTION ( 'NONE',  ( 1.000000000000000000, 0.000000000000000000, 0.000000000000000000 ) ) ;
#35494=VECTOR ( 'NONE', #55829, 1000.000000000000000 ) ;
#35516=CARTESIAN_POINT ( 'NONE',  ( 10.85068991645999859, -4.478102922274999287, 6.162028334171000488 ) ) ;
#35519=CARTESIAN_POINT ( 'NONE',  ( 7.983191940377000861, -5.321924421352999701, 8.118250081378000971 ) ) ;
#35523=CARTESIAN_POINT ( 'NONE',  ( 10.98688827724942207, -5.367975154760490142, -6.994477628653238632 ) ) ;
#35526=CARTESIAN_POINT ( 'NONE',  ( 9.179055905797000037, -2.899999999999999911, 6.571291218949999902 ) ) ;
#35527=CARTESIAN_POINT ( 'NONE',  ( 8.199995110659001440, -2.894508759333000114, 6.645190873281999089 ) ) ;
#35528=ORIENTED_EDGE ( 'NONE', *, *, #12235, .F. ) ;
#35529=CARTESIAN_POINT ( 'NONE',  ( 8.679055905797000037, -2.899999999999999911, 6.571291218949999902 ) ) ;
#35534=CARTESIAN_POINT ( 'NONE',  ( 10.91944543538999923, -3.268376408192000149, -6.413937436229999456 ) ) ;
#35554=CARTESIAN_POINT ( 'NONE',  ( 10.20917469696999902, -3.334764780022000163, -5.769478358936999562 ) ) ;
#35557=VERTEX_POINT ( 'NONE', #53454 ) ;
#35562=CARTESIAN_POINT ( 'NONE',  ( 7.758191940376999440, -5.797088532631000213, 8.340479314546998424 ) ) ;
#35575=CARTESIAN_POINT ( 'NONE',  ( 7.358058059621999547, -4.561648098548999997, 6.153050355516999304 ) ) ;
#35576=B_SPLINE_CURVE_WITH_KNOTS ( 'NONE', 3,
 ( #17539, #28731, #50044, #2154, #23471, #60878, #66112 ),
 .UNSPECIFIED., .F., .F.,
 ( 4, 1, 1, 1, 4 ),
 ( 0.000000000000000000, 0.2500000039165359289, 0.5000000015352937810, 0.7499999991540515776, 1.000000000000000000 ),
 .UNSPECIFIED. ) ;
#35586=ORIENTED_EDGE ( 'NONE', *, *, #39003, .F. ) ;
#35587=ADVANCED_FACE ( 'NONE', ( #23008 ), #8251, .T. ) ;
#35596=CARTESIAN_POINT ( 'NONE',  ( 8.242389367084641094, -5.499373901227779804, 8.386263970964396464 ) ) ;
#35600=CARTESIAN_POINT ( 'NONE',  ( 10.33327595171000013, -4.639045857913999704, -4.712793788258000660 ) ) ;
#35604=AXIS2_PLACEMENT_3D ( 'NONE', #11599, #23136, #38172 ) ;
#35606=CARTESIAN_POINT ( 'NONE',  ( 9.837156140204001531, -5.811247906278000031, -7.978055797018001272 ) ) ;
#35614=EDGE_CURVE ( 'NONE', #20205, #9159, #18278, .T. ) ;
#35619=CARTESIAN_POINT ( 'NONE',  ( 7.571668146791999732, -2.531197775378000170, 8.216705951490000714 ) ) ;
#35620=LINE ( 'NONE', #20209, #68088 ) ;
#35621=EDGE_LOOP ( 'NONE', ( #59321, #32538, #46148, #47740 ) ) ;
#35624=CARTESIAN_POINT ( 'NONE',  ( 11.24323064679000161, -2.479730344050999680, -7.587230764681999418 ) ) ;
#35627=CARTESIAN_POINT ( 'NONE',  ( 7.399258644420781295, -3.999959970822239530, 9.109379115530307658 ) ) ;
#35635=LINE ( 'NONE', #56264, #26925 ) ;
#35643=CARTESIAN_POINT ( 'NONE',  ( 10.31298165360644425, -2.920330592985297624, -8.329669302950559739 ) ) ;
#35658=CARTESIAN_POINT ( 'NONE',  ( 10.94563198394039283, -2.254998712725911236, 7.605124749578603627 ) ) ;
#35668=EDGE_CURVE ( 'NONE', #606, #54866, #27213, .T. ) ;
#35669=ADVANCED_FACE ( 'NONE', ( #23495 ), #12667, .T. ) ;
#35673=CARTESIAN_POINT ( 'NONE',  ( 8.373668146795001377, -2.202816532622999812, 7.706987678916999762 ) ) ;
#35680=CARTESIAN_POINT ( 'NONE',  ( 7.454383804049630413, -2.263917759343326619, 7.386920749780896855 ) ) ;
#35689=CARTESIAN_POINT ( 'NONE',  ( 8.474485200571999499, -5.100000000000000533, 6.560614371780999043 ) ) ;
#35691=CARTESIAN_POINT ( 'NONE',  ( 10.99937785741359519, -5.205492584227198627, 6.645915226615812799 ) ) ;
#35696=EDGE_CURVE ( 'NONE', #35912, #15625, #38385, .T. ) ;
#35698=CARTESIAN_POINT ( 'NONE',  ( 8.933148997457999840, -5.167567567567999731, 6.822293592207000934 ) ) ;
#35703=CARTESIAN_POINT ( 'NONE',  ( 7.000000000000000000, -0.2897247358851999799, -3.000000000000000000 ) ) ;
#35705=CARTESIAN_POINT ( 'NONE',  ( 10.90638082498000117, -5.227498618488000126, 6.784459667733999666 ) ) ;
#35707=CARTESIAN_POINT ( 'NONE',  ( 9.973487588364999823, -4.344961837988999598, -9.321582626371998970 ) ) ;
#35709=CARTESIAN_POINT ( 'NONE',  ( 10.90227388941000086, -5.099948884123999271, -5.143660596970000221 ) ) ;
#35717=CARTESIAN_POINT ( 'NONE',  ( 9.298040139821001304, -4.087076480742000584, 9.429402848390999736 ) ) ;
#35721=ORIENTED_EDGE ( 'NONE', *, *, #61088, .T. ) ;
#35733=DIRECTION ( 'NONE',  ( -0.7071067811865475727, 0.7071067811865475727, 0.000000000000000000 ) ) ;
#35752=EDGE_CURVE ( 'NONE', #43226, #27541, #47583, .T. ) ;
#35759=CARTESIAN_POINT ( 'NONE',  ( 9.048302809847001527, -2.866747332746000243, -6.341063895044004362 ) ) ;
#35767=CARTESIAN_POINT ( 'NONE',  ( 8.266851002545999805, -2.832432432432000269, 6.822293592207000934 ) ) ;
#35768=DIRECTION ( 'NONE',  ( 0.000000000000000000, 0.000000000000000000, -1.000000000000000000 ) ) ;
#35774=CARTESIAN_POINT ( 'NONE',  ( 8.507804550190643411, -4.678883388517643738, 8.679043930492003511 ) ) ;
#35786=B_SPLINE_CURVE_WITH_KNOTS ( 'NONE', 3,
 ( #39837, #2423, #35627, #29708 ),
 .UNSPECIFIED., .F., .F.,
 ( 4, 4 ),
 ( 0.000000000000000000, 1.000000000000000000 ),
 .UNSPECIFIED. ) ;
#35794=EDGE_CURVE ( 'NONE', #46842, #10663, #27434, .T. ) ;
#35804=CIRCLE ( 'NONE', #29134, 1.449999999999999956 ) ;
#35806=CARTESIAN_POINT ( 'NONE',  ( 8.716851002545999094, -2.832432432432000269, 6.822293592207000934 ) ) ;
#35808=ORIENTED_EDGE ( 'NONE', *, *, #100, .T. ) ;
#35822=CARTESIAN_POINT ( 'NONE',  ( 10.36995232148000134, -3.372430527473000428, -5.009914361523000181 ) ) ;
#35823=CARTESIAN_POINT ( 'NONE',  ( 9.707733921870000060, -2.624754973437999794, -6.486841649805000110 ) ) ;
#35831=CARTESIAN_POINT ( 'NONE',  ( 7.913666363270997373, -4.616745235331003450, 6.306613118563004328 ) ) ;
#35850=CARTESIAN_POINT ( 'NONE',  ( 10.51654446536000087, -4.930670681812999945, 8.573593359022000371 ) ) ;
#35854=CARTESIAN_POINT ( 'NONE',  ( 8.368316940379001423, -4.780993534312999671, 6.267212032957000467 ) ) ;
#35859=VECTOR ( 'NONE', #19393, 1000.000000000000114 ) ;
#35864=ORIENTED_EDGE ( 'NONE', *, *, #27795, .T. ) ;
#35867=FACE_OUTER_BOUND ( 'NONE', #31756, .T. ) ;
#35869=CARTESIAN_POINT ( 'NONE',  ( 10.09454055528000005, -5.362855569781999954, -7.550030734599999960 ) ) ;
#35870=CARTESIAN_POINT ( 'NONE',  ( 10.76947109217999810, -5.100000000000000533, -6.152188490330000370 ) ) ;
#35880=CARTESIAN_POINT ( 'NONE',  ( 8.186778834302003816, -5.111320685747004156, 6.695945149192998436 ) ) ;
#35901=CARTESIAN_POINT ( 'NONE',  ( 9.129428851719998406, -5.099284414202999827, 6.151604790022999758 ) ) ;
#35906=CARTESIAN_POINT ( 'NONE',  ( 8.951355646795001064, -2.821866379289000193, 6.127148604720000336 ) ) ;
#35912=VERTEX_POINT ( 'NONE', #11454 ) ;
#35922=CARTESIAN_POINT ( 'NONE',  ( 7.000000092426000187, -9.186879080274000131, 5.186879143973999184 ) ) ;
#35925=CARTESIAN_POINT ( 'NONE',  ( 7.839304865445928527, -5.021524044172331891, 6.546612932266471674 ) ) ;
#35928=CARTESIAN_POINT ( 'NONE',  ( 8.128419906718608701, -5.085263205253937713, 6.140446736834060282 ) ) ;
#35931=CARTESIAN_POINT ( 'NONE',  ( 10.31724051754000016, -4.562409174416999669, -4.565398975579999963 ) ) ;
#35937=CARTESIAN_POINT ( 'NONE',  ( 9.490308298768001194, -5.536248950452999473, -7.355084988757000453 ) ) ;
#35951=CARTESIAN_POINT ( 'NONE',  ( 11.01605564679000082, -5.482859940357000639, -7.846409404949000077 ) ) ;
#35983=CARTESIAN_POINT ( 'NONE',  ( 10.97807333593999957, -5.235090452703000885, -6.783100406990000053 ) ) ;
#35999=PRODUCT_DEFINITION_CONTEXT ( 'detailed design', #56566, 'design' ) ;
#36007=CARTESIAN_POINT ( 'NONE',  ( 9.041941940379999210, -2.707994276285999646, 5.994456121676999594 ) ) ;
#36012=CARTESIAN_POINT ( 'NONE',  ( 7.645335379506589035, -5.356736300262827655, 6.411841797474306048 ) ) ;
#36037=CARTESIAN_POINT ( 'NONE',  ( 9.625489929093001606, -3.134630999349000025, 8.626959345509000343 ) ) ;
#36042=VERTEX_POINT ( 'NONE', #17399 ) ;
#36044=CARTESIAN_POINT ( 'NONE',  ( 11.01655351471000088, -6.705640160583000053, -5.522669566710000311 ) ) ;
#36078=ORIENTED_EDGE ( 'NONE', *, *, #52554, .F. ) ;
#36082=CARTESIAN_POINT ( 'NONE',  ( 9.634027193201999850, -3.042970193091000031, 8.588108172435999776 ) ) ;
#36085=FACE_OUTER_BOUND ( 'NONE', #65869, .T. ) ;
#36093=CARTESIAN_POINT ( 'NONE',  ( 10.98768472639999949, -0.3876847264043000174, 4.945212061661000469 ) ) ;
#36095=EDGE_CURVE ( 'NONE', #63766, #11391, #3740, .T. ) ;
#36097=CARTESIAN_POINT ( 'NONE',  ( 8.819279415752005136, -3.128895434138999843, -6.198312589903004266 ) ) ;
#36100=CARTESIAN_POINT ( 'NONE',  ( 10.96500214151999941, -2.847408127283999946, -5.071952786765999477 ) ) ;
#36102=CARTESIAN_POINT ( 'NONE',  ( 9.642108463020875320, -3.293853022145220688, 8.705313308395860261 ) ) ;
#36108=CARTESIAN_POINT ( 'NONE',  ( 11.09999999999999964, -7.940796613052000019, 6.945951997396999644 ) ) ;
#36113=EDGE_LOOP ( 'NONE', ( #67758, #23697, #69189, #42904, #62186, #60165, #63891, #31505 ) ) ;
#36121=CARTESIAN_POINT ( 'NONE',  ( 11.05853316602999925, -8.013872486471999679, 6.925173420900999410 ) ) ;
#36125=EDGE_LOOP ( 'NONE', ( #18222, #26437, #44815, #3378 ) ) ;
#36142=CARTESIAN_POINT ( 'NONE',  ( 11.05490012380000131, -5.246473031683000166, -5.052786172115000696 ) ) ;
#36147=CARTESIAN_POINT ( 'NONE',  ( 10.98277446826000059, -2.518728855032000169, -8.314788219120000434 ) ) ;
#36149=ORIENTED_EDGE ( 'NONE', *, *, #2489, .F. ) ;
#36159=CARTESIAN_POINT ( 'NONE',  ( 8.046990059540997109, -3.146252403201002856, 6.173090499042001689 ) ) ;
#36161=CARTESIAN_POINT ( 'NONE',  ( 11.04783424078000031, -2.764605797469000148, 5.041477660832000218 ) ) ;
#36163=CARTESIAN_POINT ( 'NONE',  ( 10.31726253785999958, -3.438690054218000114, -4.565404970506000026 ) ) ;
#36167=CARTESIAN_POINT ( 'NONE',  ( 11.01870309098000078, -5.269007982505999443, -4.994855899974000479 ) ) ;
#36182=CARTESIAN_POINT ( 'NONE',  ( 10.88314899746000108, -5.167567567567999731, 6.822293592207000934 ) ) ;
#36185=CARTESIAN_POINT ( 'NONE',  ( 9.679055905794999859, -2.899999999999999911, 6.571291218949999902 ) ) ;
#36191=CARTESIAN_POINT ( 'NONE',  ( 11.18483536755999808, -2.599651619047000040, 7.740676724427999922 ) ) ;
#36193=CARTESIAN_POINT ( 'NONE',  ( 7.664150527885400521, -2.651202557357406508, 7.676969588268241829 ) ) ;
#36194=CARTESIAN_POINT ( 'NONE',  ( 7.673644353206999114, -4.696237245142999228, 5.830277424166999900 ) ) ;
#36196=ORIENTED_EDGE ( 'NONE', *, *, #23704, .F. ) ;
#36204=CARTESIAN_POINT ( 'NONE',  ( 10.46432358320999967, -2.042767395367000027, 7.723698102088000006 ) ) ;
#36208=CARTESIAN_POINT ( 'NONE',  ( 10.89218817467000200, -2.661900611977999986, -8.236035141896001832 ) ) ;
#36210=CARTESIAN_POINT ( 'NONE',  ( 10.98953890776364872, -6.637400546507714161, -5.389624950907599299 ) ) ;
#36219=CARTESIAN_POINT ( 'NONE',  ( 8.716851002545999094, -2.832432432432000269, 6.822293592207000934 ) ) ;
#36221=CARTESIAN_POINT ( 'NONE',  ( 10.90638082498000117, -5.227498618488000126, 6.784459667733999666 ) ) ;
#36225=ORIENTED_EDGE ( 'NONE', *, *, #52700, .T. ) ;
#36227=CARTESIAN_POINT ( 'NONE',  ( 11.04782425406999913, -5.235403588978999601, 5.041461677707999911 ) ) ;
#36231=CARTESIAN_POINT ( 'NONE',  ( 9.341766659739111134, -5.749051749107375819, -7.541331268112342556 ) ) ;
#36240=VECTOR ( 'NONE', #28715, 1000.000000000000000 ) ;
#36247=CARTESIAN_POINT ( 'NONE',  ( 10.66052890781999984, -2.899999999999999911, -6.152188490330000370 ) ) ;
#36249=CARTESIAN_POINT ( 'NONE',  ( 8.539831853209999935, -5.633481712366999794, 7.451234046297000368 ) ) ;
#36253=ORIENTED_EDGE ( 'NONE', *, *, #62444, .T. ) ;
#36260=DIRECTION ( 'NONE',  ( 0.000000000000000000, 1.000000000000000000, 0.000000000000000000 ) ) ;
#36267=CARTESIAN_POINT ( 'NONE',  ( 7.871384613761001070, -5.129340912189999990, 6.740051747100999968 ) ) ;
#36270=CARTESIAN_POINT ( 'NONE',  ( 8.287139215840040762, -4.779713743860946273, 9.054660631579276142 ) ) ;
#36273=CARTESIAN_POINT ( 'NONE',  ( 10.41219359575999981, -4.853866617716000142, -4.884258404949999743 ) ) ;
#36274=CARTESIAN_POINT ( 'NONE',  ( 10.43314899746000002, -5.167567567567999731, 6.822293592207000934 ) ) ;
#36279=CARTESIAN_POINT ( 'NONE',  ( 9.446306596383999832, -5.231133027468000130, -6.569831606205999819 ) ) ;
#36283=DIRECTION ( 'NONE',  ( 0.000000000000000000, -1.000000000000000000, 0.000000000000000000 ) ) ;
#36286=ORIENTED_EDGE ( 'NONE', *, *, #18427, .T. ) ;
#36287=CARTESIAN_POINT ( 'NONE',  ( 9.096071945540000314, -5.102479135096000817, -6.621020973615999061 ) ) ;
#36292=CARTESIAN_POINT ( 'NONE',  ( 10.24394435321000074, -3.220344030624999743, -6.005416930865999703 ) ) ;
#36305=CARTESIAN_POINT ( 'NONE',  ( 5.000000000000000000, 0.000000000000000000, 0.000000000000000000 ) ) ;
#36307=CARTESIAN_POINT ( 'NONE',  ( 10.26195629121000152, -3.399999734730999812, 4.591198190832999515 ) ) ;
#36313=DIRECTION ( 'NONE',  ( 0.000000000000000000, 1.000000000000000000, 0.000000000000000000 ) ) ;
#36315=VERTEX_POINT ( 'NONE', #47072 ) ;
#36321=EDGE_CURVE ( 'NONE', #49429, #67945, #35214, .T. ) ;
#36324=DIRECTION ( 'NONE',  ( -0.5298945028671029345, -0.5996714985845039703, 0.5996715014211040362 ) ) ;
#36350=CARTESIAN_POINT ( 'NONE',  ( 11.05947712336570632, -5.538520942942948722, 7.349130516419520198 ) ) ;
#36351=CARTESIAN_POINT ( 'NONE',  ( 9.015543146794000151, -4.175914961544999748, 5.699510287082000026 ) ) ;
#36355=CARTESIAN_POINT ( 'NONE',  ( 10.38053305961999939, -5.283785200568999585, -8.830188095997000275 ) ) ;
#36356=CARTESIAN_POINT ( 'NONE',  ( 7.617277775139868368, -4.886096859513470392, 6.002900497088587528 ) ) ;
#36376=CARTESIAN_POINT ( 'NONE',  ( 9.705773468360421319, -5.100000000000000533, -6.304440313841761068 ) ) ;
#36383=CARTESIAN_POINT ( 'NONE',  ( 9.298040139821001304, -4.087076480742000584, 9.429402848390999736 ) ) ;
#36398=CARTESIAN_POINT ( 'NONE',  ( 10.94797187187000098, -2.864324950622999744, 8.846246404612999825 ) ) ;
#36405=CARTESIAN_POINT ( 'NONE',  ( 10.06343867337000120, -5.156226070197000411, 6.125223053176999777 ) ) ;
#36406=CARTESIAN_POINT ( 'NONE',  ( 9.141935773284000533, -3.399999999999999911, -6.632262360512000576 ) ) ;
#36415=CARTESIAN_POINT ( 'NONE',  ( 9.267891187585000523, -4.645169647889000331, -5.840816811670999975 ) ) ;
#36443=CARTESIAN_POINT ( 'NONE',  ( 11.04437549732999813, -2.755184240810999885, -5.169198519660000990 ) ) ;
#36444=CARTESIAN_POINT ( 'NONE',  ( 11.09992055961999924, -2.373397911211000189, -6.776606350776999577 ) ) ;
#36449=DIRECTION ( 'NONE',  ( 0.7071067811865475727, -0.7071067811865475727, 0.000000000000000000 ) ) ;
#36457=ORIENTED_EDGE ( 'NONE', *, *, #15179, .F. ) ;
#36480=CARTESIAN_POINT ( 'NONE',  ( 7.945608795480825215, -5.314576234847506520, 7.853946780411532380 ) ) ;
#36481=CARTESIAN_POINT ( 'NONE',  ( 8.410398127216412334, -5.351350780489295467, 7.263115598813800311 ) ) ;
#36488=CARTESIAN_POINT ( 'NONE',  ( 10.73506343560000076, -5.202499304193000107, -8.441414596927000247 ) ) ;
#36500=PLANE ( 'NONE',  #3986 ) ;
#36504=CARTESIAN_POINT ( 'NONE',  ( 8.335542453529990681, -2.897657451248000893, 6.653312621732999865 ) ) ;
#36508=CARTESIAN_POINT ( 'NONE',  ( 10.00137895011999944, -3.855365288061999962, 5.709482985498999241 ) ) ;
#36525=LINE ( 'NONE', #15549, #68383 ) ;
#36536=CARTESIAN_POINT ( 'NONE',  ( 11.00366278039000001, -2.264082614160999984, 7.798350693290999835 ) ) ;
#36537=ORIENTED_EDGE ( 'NONE', *, *, #56274, .T. ) ;
#36539=CARTESIAN_POINT ( 'NONE',  ( 8.572269353210000276, -2.606998386752999775, 6.345764833140000505 ) ) ;
#36543=LINE ( 'NONE', #57869, #59511 ) ;
#36548=ORIENTED_EDGE ( 'NONE', *, *, #43260, .T. ) ;
#36549=CARTESIAN_POINT ( 'NONE',  ( 10.18755811987000115, -5.387486580809999204, 8.640943191857999750 ) ) ;
#36551=CARTESIAN_POINT ( 'NONE',  ( 7.307500000000000107, -0.2999999999999999889, -3.149999999999999911 ) ) ;
#36553=CARTESIAN_POINT ( 'NONE',  ( 10.72303951155000057, -3.890113427500999421, -8.859339185702999941 ) ) ;
#36559=CARTESIAN_POINT ( 'NONE',  ( 5.600000001140999828, 0.000000000000000000, 0.000000000000000000 ) ) ;
#36560=FACE_OUTER_BOUND ( 'NONE', #8872, .T. ) ;
#36565=CARTESIAN_POINT ( 'NONE',  ( 10.40516264833000015, -5.216401621862000404, 6.765753642936999768 ) ) ;
#36566=ORIENTED_EDGE ( 'NONE', *, *, #34188, .F. ) ;
#36583=CARTESIAN_POINT ( 'NONE',  ( 9.298691940377999288, -5.159251056493999954, 9.109488373271000583 ) ) ;
#36597=CARTESIAN_POINT ( 'NONE',  ( 7.262120559621999760, -4.847802017252000439, 9.065364004483999594 ) ) ;
#36598=CARTESIAN_POINT ( 'NONE',  ( 9.208105646793001142, -5.057079407184000175, 8.967634647348999621 ) ) ;
#36617=DIRECTION ( 'NONE',  ( 0.000000000000000000, 0.000000000000000000, 1.000000000000000000 ) ) ;
#36618=CARTESIAN_POINT ( 'NONE',  ( 8.171101097212417841, -5.642366377685726242, 6.904702228779299844 ) ) ;
#36621=CARTESIAN_POINT ( 'NONE',  ( 10.90000000346999975, -5.100000000044000892, -5.157071296039999808 ) ) ;
#36629=CARTESIAN_POINT ( 'NONE',  ( 9.712899699504999873, -4.008306780893000187, -8.877926425468999128 ) ) ;
#36640=CARTESIAN_POINT ( 'NONE',  ( 11.05574479014000211, -5.246314385833000138, 5.054138008665999493 ) ) ;
#36641=ORIENTED_EDGE ( 'NONE', *, *, #22465, .F. ) ;
#36643=CIRCLE ( 'NONE', #44446, 1.250000000000000000 ) ;
#36644=DIRECTION ( 'NONE',  ( -1.000000000000000000, 0.000000000000000000, 0.000000000000000000 ) ) ;
#36653=B_SPLINE_CURVE_WITH_KNOTS ( 'NONE', 3,
 ( #43472, #26704, #38210, #37870 ),
 .UNSPECIFIED., .F., .F.,
 ( 4, 4 ),
 ( 0.000000000000000000, 1.000000000000000000 ),
 .UNSPECIFIED. ) ;
#36661=CARTESIAN_POINT ( 'NONE',  ( 10.72303951155000057, -3.890113427500999421, -8.859339185702999941 ) ) ;
#36668=CARTESIAN_POINT ( 'NONE',  ( 8.650504956611454688, -4.887017940256735749, -6.482196879590077288 ) ) ;
#36681=CARTESIAN_POINT ( 'NONE',  ( 9.092670730108844523, -4.128092163117982771, 8.851211507171084847 ) ) ;
#36689=ORIENTED_EDGE ( 'NONE', *, *, #20203, .F. ) ;
#36691=CARTESIAN_POINT ( 'NONE',  ( 6.799999045260999964, -9.295457794069999835, 5.399713664196000629 ) ) ;
#36703=CARTESIAN_POINT ( 'NONE',  ( 8.924956853209002006, -4.158911960977000000, 5.873536005760000123 ) ) ;
#36709=FACE_OUTER_BOUND ( 'NONE', #43785, .T. ) ;
#36710=CARTESIAN_POINT ( 'NONE',  ( 7.533751553497644693, -3.156652531865319133, 5.968239819955745595 ) ) ;
#36737=CARTESIAN_POINT ( 'NONE',  ( 10.27968096967000022, -5.739708848514999850, 7.774962785835000112 ) ) ;
#36746=CARTESIAN_POINT ( 'NONE',  ( 7.000000000000000000, -6.255435840762999966, 3.000000000000000000 ) ) ;
#36750=VECTOR ( 'NONE', #43219, 1000.000000000000000 ) ;
#36758=CARTESIAN_POINT ( 'NONE',  ( 10.87021507563000000, -2.226042145532000305, 7.782753277595999997 ) ) ;
#36764=CARTESIAN_POINT ( 'NONE',  ( 9.443897997121000643, -4.993413662857000723, -9.088148847710000311 ) ) ;
#36772=VERTEX_POINT ( 'NONE', #16367 ) ;
#36775=CARTESIAN_POINT ( 'NONE',  ( 9.882266086202999844, -4.932716797830999589, 6.390980246320999925 ) ) ;
#36782=EDGE_CURVE ( 'NONE', #21554, #43226, #9835, .T. ) ;
#36795=CARTESIAN_POINT ( 'NONE',  ( 9.619904806657000762, -2.133039813254999917, -7.346564890486999566 ) ) ;
#36796=CARTESIAN_POINT ( 'NONE',  ( 10.11549555961999936, -2.489199523559999960, -6.434642413229999747 ) ) ;
#36818=CARTESIAN_POINT ( 'NONE',  ( 10.90000000000000036, -1.300000000000000044, -9.662944685757000940 ) ) ;
#36823=AXIS2_PLACEMENT_3D ( 'NONE', #16225, #25688, #62737 ) ;
#36839=CARTESIAN_POINT ( 'NONE',  ( 10.48735240295000004, -4.351290250877999810, -6.182246784057000788 ) ) ;
#36842=ORIENTED_EDGE ( 'NONE', *, *, #45626, .T. ) ;
#36845=PLANE ( 'NONE',  #49979 ) ;
#36851=FACE_OUTER_BOUND ( 'NONE', #4427, .T. ) ;
#36855=CARTESIAN_POINT ( 'NONE',  ( 8.500486250726996929, -2.902641158998001458, 6.605591905707999700 ) ) ;
#36858=CARTESIAN_POINT ( 'NONE',  ( 10.18755811987000115, -5.387486580809999204, 8.640943191857999750 ) ) ;
#36862=ADVANCED_FACE ( 'NONE', ( #56193 ), #50260, .F. ) ;
#36870=CARTESIAN_POINT ( 'NONE',  ( 10.31498017945871126, -2.650031506806249659, -7.499998780888571304 ) ) ;
#36875=CARTESIAN_POINT ( 'NONE',  ( 8.241912900173000267, -4.599999999999999645, 6.117539782833000928 ) ) ;
#36887=CARTESIAN_POINT ( 'NONE',  ( 10.89228096335999929, -3.998355205482000851, 9.261304730013998565 ) ) ;
#36890=ORIENTED_EDGE ( 'NONE', *, *, #22746, .T. ) ;
#36891=ADVANCED_FACE ( 'NONE', ( #7608 ), #12860, .T. ) ;
#36892=CARTESIAN_POINT ( 'NONE',  ( 6.953073139469000630, -9.233001678504999532, 5.200628701625999994 ) ) ;
#36893=CARTESIAN_POINT ( 'NONE',  ( 7.326308059621999824, -3.394845988290999816, 9.388942682504000103 ) ) ;
#36894=LINE ( 'NONE', #168, #41150 ) ;
#36901=CARTESIAN_POINT ( 'NONE',  ( 9.538434317036999843, -5.620900626097999897, 7.423100105894999245 ) ) ;
#36916=CARTESIAN_POINT ( 'NONE',  ( 8.244326721667006197, -4.955553483043997787, 6.175174249266997428 ) ) ;
#36927=DIRECTION ( 'NONE',  ( -0.9999999999999998890, 4.498712764241000040E-09, -1.506424703057999482E-08 ) ) ;
#36935=CARTESIAN_POINT ( 'NONE',  ( 9.041941940379999210, -2.707994276285999646, 5.994456121676999594 ) ) ;
#36946=CARTESIAN_POINT ( 'NONE',  ( 7.647245559622000144, -5.850279024084999335, 6.784181137144999596 ) ) ;
#36960=CARTESIAN_POINT ( 'NONE',  ( 11.09999999999999964, -2.899999999999999911, 4.467422426380999845 ) ) ;
#36965=CARTESIAN_POINT ( 'NONE',  ( 8.541089604138797142, -3.299759450154362117, 5.908022738197796109 ) ) ;
#36981=FACE_OUTER_BOUND ( 'NONE', #32675, .T. ) ;
#36987=CARTESIAN_POINT ( 'NONE',  ( 7.583058059622000080, -4.763531818439999732, 5.668890958491999754 ) ) ;
#37012=CARTESIAN_POINT ( 'NONE',  ( 8.740166936413396925, -4.651882090383574919, -6.316683530224510790 ) ) ;
#37029=CARTESIAN_POINT ( 'NONE',  ( 10.99590832059627132, -2.534418414327098468, 6.542952895858777929 ) ) ;
#37035=CARTESIAN_POINT ( 'NONE',  ( 9.271640687504833167, -2.873222873817937284, 6.752018918866299124 ) ) ;
#37044=CARTESIAN_POINT ( 'NONE',  ( 9.208105646793001142, -5.057079407184000175, 8.967634647348999621 ) ) ;
#37048=CARTESIAN_POINT ( 'NONE',  ( 10.94847055962000049, -3.841065069379000274, -9.341805385095000247 ) ) ;
#37049=CARTESIAN_POINT ( 'NONE',  ( 7.469483898962876900, -2.313341745386989334, 7.073925100461147863 ) ) ;
#37059=ORIENTED_EDGE ( 'NONE', *, *, #43881, .T. ) ;
#37067=LINE ( 'NONE', #69195, #66230 ) ;
#37072=CARTESIAN_POINT ( 'NONE',  ( 10.97719478263000070, -5.298911744033000026, 4.940093110104999852 ) ) ;
#37078=CARTESIAN_POINT ( 'NONE',  ( 9.667080975990000269, -4.541622198376999542, 5.824041840233000755 ) ) ;
#37091=CARTESIAN_POINT ( 'NONE',  ( 9.242852049159891337, -2.682263764936901662, 7.207900080852989610 ) ) ;
#37099=CARTESIAN_POINT ( 'NONE',  ( 10.93728138146000006, -5.425439422033999648, 7.240583766112999697 ) ) ;
#37104=CARTESIAN_POINT ( 'NONE',  ( 7.766851002543999627, -2.832432432432000269, 6.822293592207000934 ) ) ;
#37116=VECTOR ( 'NONE', #68858, 999.9999999999998863 ) ;
#37119=CARTESIAN_POINT ( 'NONE',  ( 10.99934110471000004, -5.081022574063999819, 8.239050178861999640 ) ) ;
#37128=CARTESIAN_POINT ( 'NONE',  ( 8.455992358812000731, -4.599999999999999645, 6.571291218949999902 ) ) ;
#37133=CARTESIAN_POINT ( 'NONE',  ( 9.487899699504998452, -4.011292643094999555, -9.373220388412001114 ) ) ;
#37135=EDGE_CURVE ( 'NONE', #66793, #25777, #62208, .T. ) ;
#37147=DIRECTION ( 'NONE',  ( 1.000000000000000000, 0.000000000000000000, 0.000000000000000000 ) ) ;
#37149=ORIENTED_EDGE ( 'NONE', *, *, #30017, .F. ) ;
#37169=EDGE_CURVE ( 'NONE', #30230, #60711, #39682, .T. ) ;
#37177=CARTESIAN_POINT ( 'NONE',  ( 9.976697000975999430, -4.172225768856000272, -6.147144998063999388 ) ) ;
#37180=ORIENTED_EDGE ( 'NONE', *, *, #19477, .T. ) ;
#37189=CARTESIAN_POINT ( 'NONE',  ( 10.26027384100999917, -3.427607989534000144, 4.531780802426999877 ) ) ;
#37190=FACE_OUTER_BOUND ( 'NONE', #33588, .T. ) ;
#37198=CARTESIAN_POINT ( 'NONE',  ( 9.471368011205999693, -2.030678448189000118, 7.549764202121000523 ) ) ;
#37211=CARTESIAN_POINT ( 'NONE',  ( 8.228368194306998618, -4.806758213702000404, 6.177034600996000435 ) ) ;
#37213=FACE_OUTER_BOUND ( 'NONE', #31256, .T. ) ;
#37218=DIRECTION ( 'NONE',  ( 1.000000000000000000, 0.000000000000000000, 0.000000000000000000 ) ) ;
#37222=ORIENTED_EDGE ( 'NONE', *, *, #20396, .F. ) ;
#37223=B_SPLINE_CURVE_WITH_KNOTS ( 'NONE', 3,
 ( #35247, #46072, #67378, #25775, #4092, #25429, #46762, #48133, #6157, #16310, #58274, #53381, #11071, #32064, #32744 ),
 .UNSPECIFIED., .F., .F.,
 ( 4, 2, 2, 2, 1, 2, 2, 4 ),
 ( 0.000000000000000000, 0.2500000000000199840, 0.3750000000000303646, 0.4375000000000324185, 0.4687500000000315858, 0.4843750000000310307, 0.5000000000000305311, 1.000000000000000000 ),
 .UNSPECIFIED. ) ;
#37224=CARTESIAN_POINT ( 'NONE',  ( 10.78089914631999946, -5.735295708369000600, 7.801561210335000496 ) ) ;
#37228=CARTESIAN_POINT ( 'NONE',  ( 8.187144353207999714, -4.968144979409999884, 5.971795951526999602 ) ) ;
#37232=CARTESIAN_POINT ( 'NONE',  ( 9.906851002540999929, -2.832432432432000269, -6.822293592207000934 ) ) ;
#37236=ORIENTED_EDGE ( 'NONE', *, *, #34272, .T. ) ;
#37237=CARTESIAN_POINT ( 'NONE',  ( 10.09697182628999990, -5.253379538902000156, 8.530665717066000298 ) ) ;
#37241=ORIENTED_EDGE ( 'NONE', *, *, #45006, .F. ) ;
#37243=DIRECTION ( 'NONE',  ( 1.000000000000000000, 7.105427357289000429E-14, 1.065814103592999999E-13 ) ) ;
#37244=ORIENTED_EDGE ( 'NONE', *, *, #49105, .T. ) ;
#37251=DIRECTION ( 'NONE',  ( 0.000000000000000000, -1.000000000000000000, 0.000000000000000000 ) ) ;
#37254=CARTESIAN_POINT ( 'NONE',  ( 7.954655249370001791, -5.133340916889001626, 6.761736834907998706 ) ) ;
#37256=EDGE_LOOP ( 'NONE', ( #8670, #32060, #58294, #21896 ) ) ;
#37259=CARTESIAN_POINT ( 'NONE',  ( 11.01922882085999866, -5.268778362341000054, 4.995697847266999503 ) ) ;
#37265=CARTESIAN_POINT ( 'NONE',  ( 9.299840153678500698, -5.532928100317616504, -6.657476841886525776 ) ) ;
#37266=VERTEX_POINT ( 'NONE', #32722 ) ;
#37270=CARTESIAN_POINT ( 'NONE',  ( 8.400066940379998570, -2.800111029801999774, 9.079936276749000612 ) ) ;
#37282=ORIENTED_EDGE ( 'NONE', *, *, #38600, .T. ) ;
#37283=CARTESIAN_POINT ( 'NONE',  ( 7.352706853207999771, -4.773080213113000347, 8.927399220053999329 ) ) ;
#37285=DIRECTION ( 'NONE',  ( -0.000000000000000000, 1.000000000000000000, 0.000000000000000000 ) ) ;
#37288=AXIS2_PLACEMENT_3D ( 'NONE', #64954, #33513, #49931 ) ;
#37294=DIRECTION ( 'NONE',  ( 0.000000000000000000, -0.1333333333333049098, -0.9910712498212373989 ) ) ;
#37301=CARTESIAN_POINT ( 'NONE',  ( 8.414745334144418720, -2.420441346954531614, 8.227856752513583061 ) ) ;
#37314=PRESENTATION_STYLE_ASSIGNMENT (( #43602 ) ) ;
#37316=AXIS2_PLACEMENT_3D ( 'NONE', #19680, #2226, #66185 ) ;
#37335=CARTESIAN_POINT ( 'NONE',  ( 9.002831022981437670, -8.696154316442465060, 6.348875575362916024 ) ) ;
#37336=ADVANCED_FACE ( 'NONE', ( #33764 ), #55789, .F. ) ;
#37357=CONICAL_SURFACE ( 'NONE', #30673, 1.349999998858999906, 0.7853981633972997312 ) ;
#37381=CARTESIAN_POINT ( 'NONE',  ( 10.29378083128999855, -3.483628580733000302, 6.176326635498999629 ) ) ;
#37382=CARTESIAN_POINT ( 'NONE',  ( 7.149102686541000118, -4.351670788182000038, 8.977200644264000218 ) ) ;
#37384=CARTESIAN_POINT ( 'NONE',  ( 9.630961809707432764, -5.349948547046357028, -7.768702954767688240 ) ) ;
#37386=CARTESIAN_POINT ( 'NONE',  ( 11.05391814679000184, -5.159486550382999859, -8.487149456222999433 ) ) ;
#37387=CARTESIAN_POINT ( 'NONE',  ( 7.742845422086257479, -5.491633101817720686, 8.395373286608034391 ) ) ;
#37388=CARTESIAN_POINT ( 'NONE',  ( 10.96080136920999948, -2.054580854576999904, 7.810082699133999995 ) ) ;
#37405=CARTESIAN_POINT ( 'NONE',  ( 11.09999999999999964, -1.300000000000000044, -9.662944685757000940 ) ) ;
#37411=CARTESIAN_POINT ( 'NONE',  ( 11.09999999999999964, -5.299524241844999928, -5.124965750789000296 ) ) ;
#37414=CARTESIAN_POINT ( 'NONE',  ( 9.351499161061999743, -4.821938821912000073, 8.950150764319998231 ) ) ;
#37449=DIRECTION ( 'NONE',  ( 0.000000000000000000, -1.000000000000000000, 0.000000000000000000 ) ) ;
#37457=CARTESIAN_POINT ( 'NONE',  ( 11.09999999999999964, -4.000000000000000000, 7.500000000000000000 ) ) ;
#37460=CARTESIAN_POINT ( 'NONE',  ( 8.716851002545999094, -2.832432432432000269, 6.822293592207000934 ) ) ;
#37461=ORIENTED_EDGE ( 'NONE', *, *, #485, .T. ) ;
#37464=CARTESIAN_POINT ( 'NONE',  ( 10.26685100253999927, -2.832432432432000269, 6.822293592207000934 ) ) ;
#37471=CARTESIAN_POINT ( 'NONE',  ( 10.25880564679000173, -2.491773655925000330, -7.289938045981000592 ) ) ;
#37489=CARTESIAN_POINT ( 'NONE',  ( 9.957462135714001406, -5.100000000000000533, -6.571291218949999902 ) ) ;
#37499=VECTOR ( 'NONE', #27399, 1000.000000000000000 ) ;
#37501=VERTEX_POINT ( 'NONE', #68300 ) ;
#37516=CARTESIAN_POINT ( 'NONE',  ( 10.06728329455999926, -4.192861215955000276, -5.985050974557999837 ) ) ;
#37531=CARTESIAN_POINT ( 'NONE',  ( 9.215289122285998502, -4.861979632688999686, 8.938813901364000003 ) ) ;
#37532=CARTESIAN_POINT ( 'NONE',  ( 9.668897997121000287, -4.730747404809998891, -8.668230005597001409 ) ) ;
#37534=CARTESIAN_POINT ( 'NONE',  ( 10.09196524370999981, -3.841385669346000231, 5.536421174581999338 ) ) ;
#37536=CARTESIAN_POINT ( 'NONE',  ( 11.09999999999999964, -2.700000000000000178, -5.157071250680000496 ) ) ;
#37550=CARTESIAN_POINT ( 'NONE',  ( 7.527700667618229424, -5.079562351722092473, 8.329181850972373624 ) ) ;
#37557=LINE ( 'NONE', #4701, #54027 ) ;
#37560=CARTESIAN_POINT ( 'NONE',  ( 10.44675369521999997, -2.885048926231000177, 8.863479194807000638 ) ) ;
#37563=CARTESIAN_POINT ( 'NONE',  ( 11.01978213580999899, -2.731808064604999586, 4.996583140031000347 ) ) ;
#37564=CARTESIAN_POINT ( 'NONE',  ( 7.968183059622999664, -2.280579276705999803, 6.510290672242000198 ) ) ;
#37566=ORIENTED_EDGE ( 'NONE', *, *, #5781, .T. ) ;
#37572=CARTESIAN_POINT ( 'NONE',  ( 11.11845396862999991, -5.767021056207999763, 7.178419201465000121 ) ) ;
#37579=CARTESIAN_POINT ( 'NONE',  ( 10.57656694038000111, -5.344897889496000865, -7.298883676216999739 ) ) ;
#37588=LINE ( 'NONE', #191, #22072 ) ;
#37590=B_SPLINE_CURVE_WITH_KNOTS ( 'NONE', 3,
 ( #43469, #38912, #66160, #49387 ),
 .UNSPECIFIED., .F., .F.,
 ( 4, 4 ),
 ( 0.000000000000000000, 1.000000000000000000 ),
 .UNSPECIFIED. ) ;
#37591=EDGE_LOOP ( 'NONE', ( #40191, #38995, #51003, #49729 ) ) ;
#37604=ORIENTED_EDGE ( 'NONE', *, *, #55932, .F. ) ;
#37609=CARTESIAN_POINT ( 'NONE',  ( 7.577019353207000485, -5.480312458445999901, 8.192326492433998908 ) ) ;
#37611=CARTESIAN_POINT ( 'NONE',  ( 10.26685100253999927, -2.832432432432000269, 6.822293592207000934 ) ) ;
#37617=LINE ( 'NONE', #220, #13158 ) ;
#37619=CARTESIAN_POINT ( 'NONE',  ( 9.214144353209000826, -5.421531391267000011, 6.381128921159999301 ) ) ;
#37621=CARTESIAN_POINT ( 'NONE',  ( 5.599999999371999770, -1.300000000000000044, 9.662944685757000940 ) ) ;
#37636=VERTEX_POINT ( 'NONE', #64775 ) ;
#37639=ADVANCED_FACE ( 'NONE', ( #36851 ), #45191, .F. ) ;
#37642=CARTESIAN_POINT ( 'NONE',  ( 8.296621455525475142, -4.598534371660971232, 9.142000767755396495 ) ) ;
#37654=CARTESIAN_POINT ( 'NONE',  ( 11.11532707317000046, -8.027733648058999805, 6.810713678640000879 ) ) ;
#37722=CARTESIAN_POINT ( 'NONE',  ( 10.81579453138999902, -5.374572909254000663, 6.698726302909000729 ) ) ;
#37723=CARTESIAN_POINT ( 'NONE',  ( 7.229683059621999419, -2.630475685621000093, 6.995953627589999613 ) ) ;
#37730=CARTESIAN_POINT ( 'NONE',  ( 11.19050685320999960, -2.516759970060999940, -6.840363309917000478 ) ) ;
#37731=CARTESIAN_POINT ( 'NONE',  ( 7.753453601445883692, -5.352470295837787440, 8.593756411513149729 ) ) ;
#37732=CARTESIAN_POINT ( 'NONE',  ( 9.629020610622001541, -5.794331084664000819, 7.414872097535999629 ) ) ;
#37747=CARTESIAN_POINT ( 'NONE',  ( 8.368316940379001423, -4.780993534312999671, 6.267212032957000467 ) ) ;
#37756=CARTESIAN_POINT ( 'NONE',  ( 9.500008250440000523, -2.279684233303000074, 7.877691491255999878 ) ) ;
#37758=VECTOR ( 'NONE', #25868, 1000.000000000000114 ) ;
#37762=ORIENTED_EDGE ( 'NONE', *, *, #18254, .T. ) ;
#37777=CARTESIAN_POINT ( 'NONE',  ( 7.773264358664000007, -2.859518314699000197, 6.768377407145999669 ) ) ;
#37778=CARTESIAN_POINT ( 'NONE',  ( 10.56492304196000021, -4.212244324161999565, 8.933470634735002136 ) ) ;
#37799=CARTESIAN_POINT ( 'NONE',  ( 9.669776904377568982, -2.899999999999999911, -6.174048679210142332 ) ) ;
#37807=VERTEX_POINT ( 'NONE', #43041 ) ;
#37818=CARTESIAN_POINT ( 'NONE',  ( 10.29666814679000097, -2.755511079787000384, -6.622434938646999392 ) ) ;
#37819=CARTESIAN_POINT ( 'NONE',  ( 11.08380555355832620, -3.999999927290649460, -9.033895164528411570 ) ) ;
#37833=CARTESIAN_POINT ( 'NONE',  ( 10.36180282789683638, -2.874603711584070354, -6.749639981064813554 ) ) ;
#37834=CARTESIAN_POINT ( 'NONE',  ( 10.02314899745999988, -5.167567567567999731, -6.822293592207000934 ) ) ;
#37837=CARTESIAN_POINT ( 'NONE',  ( 5.500000000000000000, -0.5000000000000000000, -9.662944685757000940 ) ) ;
#37839=CARTESIAN_POINT ( 'NONE',  ( 11.01003172897000049, -3.180716007396000133, -6.283809484240999943 ) ) ;
#37850=CARTESIAN_POINT ( 'NONE',  ( 9.050000000000000711, -7.679126935408000065, -5.093340497782000043 ) ) ;
#37852=CARTESIAN_POINT ( 'NONE',  ( 11.24052627608000066, -2.774025043188999895, 6.782107572692000375 ) ) ;
#37863=CARTESIAN_POINT ( 'NONE',  ( 10.82564972918999935, -5.331162346451000289, -8.542142527201001201 ) ) ;
#37865=EDGE_CURVE ( 'NONE', #16664, #10274, #48843, .T. ) ;
#37867=B_SPLINE_CURVE_WITH_KNOTS ( 'NONE', 3,
 ( #25958, #68247, #18993, #13756 ),
 .UNSPECIFIED., .F., .F.,
 ( 4, 4 ),
 ( 0.000000000000000000, 1.000000000000000000 ),
 .UNSPECIFIED. ) ;
#37870=CARTESIAN_POINT ( 'NONE',  ( 10.90437023801000116, -5.099522774867000230, 5.132565236215000049 ) ) ;
#37872=ADVANCED_FACE ( 'NONE', ( #48978 ), #30605, .F. ) ;
#37875=FACE_OUTER_BOUND ( 'NONE', #7729, .T. ) ;
#37879=CARTESIAN_POINT ( 'NONE',  ( 7.428159769834000059, -3.524402284009999331, 6.653317709399996005 ) ) ;
#37882=CARTESIAN_POINT ( 'NONE',  ( 10.34020413671000149, -4.202027362542999356, 9.459588031742001135 ) ) ;
#37885=CARTESIAN_POINT ( 'NONE',  ( 10.37373728961999930, -2.215269876326000364, 7.703982265807999497 ) ) ;
#37892=PLANE ( 'NONE',  #45115 ) ;
#37897=CARTESIAN_POINT ( 'NONE',  ( 7.933148997457998952, -5.167567567567999731, 6.822293592207000934 ) ) ;
#37900=CARTESIAN_POINT ( 'NONE',  ( 7.641998701183679188, -3.319571644187112813, 8.680369833195172191 ) ) ;
#37907=EDGE_LOOP ( 'NONE', ( #28, #66631, #46661, #55141, #31726, #68479 ) ) ;
#37908=CARTESIAN_POINT ( 'NONE',  ( 10.85738557828999973, -2.754556666341999804, 8.976367391363998749 ) ) ;
#37919=DIRECTION ( 'NONE',  ( 1.000000000000000000, 0.000000000000000000, 0.000000000000000000 ) ) ;
#37922=CARTESIAN_POINT ( 'NONE',  ( 10.22109127278999807, -2.983266195621000261, 8.764707262515999631 ) ) ;
#37927=CARTESIAN_POINT ( 'NONE',  ( 10.53870444038000009, -5.103398787993000063, -6.705198626796000205 ) ) ;
#37928=EDGE_LOOP ( 'NONE', ( #41584, #53759, #2759, #30212 ) ) ;
#37937=CARTESIAN_POINT ( 'NONE',  ( 9.325456588376336953, -3.988345520164779945, 9.239772568469039271 ) ) ;
#37944=CARTESIAN_POINT ( 'NONE',  ( 9.719606904206999687, -5.967761543230999166, 7.406644089178000101 ) ) ;
#37950=ADVANCED_FACE ( 'NONE', ( #39524 ), #59806, .T. ) ;
#37953=CARTESIAN_POINT ( 'NONE',  ( 7.236065714745352651, -2.650241189008525566, 7.323011948609822852 ) ) ;
#37955=CARTESIAN_POINT ( 'NONE',  ( 7.988543146792999927, -3.566638198986999964, 5.743608852252999775 ) ) ;
#37964=CARTESIAN_POINT ( 'NONE',  ( 11.05851190073833301, -5.258511900738333189, 6.537362761296000357 ) ) ;
#37967=CARTESIAN_POINT ( 'NONE',  ( 7.545269353206999874, -2.302293129340000188, 6.875167727519000849 ) ) ;
#37984=CARTESIAN_POINT ( 'NONE',  ( 8.531899004865357128, -3.122575144635288069, 5.996049329724215227 ) ) ;
#37986=ORIENTED_EDGE ( 'NONE', *, *, #67383, .F. ) ;
#37995=CARTESIAN_POINT ( 'NONE',  ( 10.44862608313071917, -4.356257174807515398, -9.239447894061358468 ) ) ;
#37998=ADVANCED_FACE ( 'NONE', ( #55949 ), #65279, .T. ) ;
#38024=CARTESIAN_POINT ( 'NONE',  ( 10.91944543538999923, -3.268376408192000149, -6.413937436229999456 ) ) ;
#38034=B_SPLINE_CURVE_WITH_KNOTS ( 'NONE', 3,
 ( #66191, #55719, #39988, #61302 ),
 .UNSPECIFIED., .F., .F.,
 ( 4, 4 ),
 ( 0.8746295857519847949, 1.000000000000000000 ),
 .UNSPECIFIED. ) ;
#38053=ADVANCED_FACE ( 'NONE', ( #30412 ), #2802, .T. ) ;
#38062=CARTESIAN_POINT ( 'NONE',  ( 10.96207173348999930, -5.399846879528999999, 7.743266618618998898 ) ) ;
#38066=DIRECTION ( 'NONE',  ( 4.514773433173149668E-07, -0.9999999999995329292, 8.545138996459277929E-07 ) ) ;
#38067=CARTESIAN_POINT ( 'NONE',  ( 10.81188185321000006, -4.614147550108000928, -5.930138617968999881 ) ) ;
#38068=CARTESIAN_POINT ( 'NONE',  ( 7.807026942100614875, -4.385935279688806254, 9.196252002095368638 ) ) ;
#38069=CARTESIAN_POINT ( 'NONE',  ( 10.27814441345999974, -5.521593622715999850, 8.751220666652999469 ) ) ;
#38085=CARTESIAN_POINT ( 'NONE',  ( 8.881816940380000247, -4.977917894183000236, 6.416767031887000705 ) ) ;
#38088=DIRECTION ( 'NONE',  ( -1.000000000000000000, 0.000000000000000000, 0.000000000000000000 ) ) ;
#38095=CARTESIAN_POINT ( 'NONE',  ( 10.35616740164000049, -2.777283710737999733, 8.995265811011998736 ) ) ;
#38096=PLANE ( 'NONE',  #48844 ) ;
#38127=CARTESIAN_POINT ( 'NONE',  ( 10.47530200610951034, -5.350262918594152595, 7.499984559551212904 ) ) ;
#38135=EDGE_CURVE ( 'NONE', #65197, #5301, #27313, .T. ) ;
#38145=CARTESIAN_POINT ( 'NONE',  ( 11.09999999999999964, -4.000000000000000000, -7.500000000000000000 ) ) ;
#38146=CARTESIAN_POINT ( 'NONE',  ( 7.779438594805999863, -3.186699643285999972, 6.422256653932000070 ) ) ;
#38147=CARTESIAN_POINT ( 'NONE',  ( 10.70271159698171992, -5.100000000000000533, 6.305985889763628727 ) ) ;
#38153=CARTESIAN_POINT ( 'NONE',  ( 10.86225948028000055, -2.934717151119000000, -5.172334369529000497 ) ) ;
#38154=CARTESIAN_POINT ( 'NONE',  ( 10.71315564678999976, -2.619204038425999581, -8.142086897834001746 ) ) ;
#38158=FACE_OUTER_BOUND ( 'NONE', #28461, .T. ) ;
#38170=CARTESIAN_POINT ( 'NONE',  ( 9.819055905797000605, -2.899999999999999911, -6.571291218949999902 ) ) ;
#38171=EDGE_CURVE ( 'NONE', #39230, #57495, #10107, .T. ) ;
#38172=DIRECTION ( 'NONE',  ( 0.000000000000000000, -1.000000000000000000, 0.000000000000000000 ) ) ;
#38175=CARTESIAN_POINT ( 'NONE',  ( 9.831596185961002377, -3.539228349258999984, -8.956015611440999891 ) ) ;
#38179=EDGE_LOOP ( 'NONE', ( #36457, #34451, #61311, #43258, #43752, #61378, #42326, #44143, #1552, #60609 ) ) ;
#38184=LINE ( 'NONE', #59516, #44853 ) ;
#38197=CARTESIAN_POINT ( 'NONE',  ( 10.49316300899723764, -4.959452674051987309, 8.606795388839010741 ) ) ;
#38205=CARTESIAN_POINT ( 'NONE',  ( 10.66852499011999988, -4.435470817312999969, -5.866470266317000082 ) ) ;
#38210=CARTESIAN_POINT ( 'NONE',  ( 10.94916232721328164, -5.139975539640455615, 5.103975416952581945 ) ) ;
#38222=CARTESIAN_POINT ( 'NONE',  ( 7.799092354096995194, -3.518505934209000152, 6.398021147088998717 ) ) ;
#38225=CARTESIAN_POINT ( 'NONE',  ( 10.84168850528999961, -2.681008214828000114, 6.554752254946000889 ) ) ;
#38227=LINE ( 'NONE', #8746, #55523 ) ;
#38236=CARTESIAN_POINT ( 'NONE',  ( 8.214872468085966162, -2.885034057788420370, 6.708591534144135338 ) ) ;
#38237=DIRECTION ( 'NONE',  ( 1.000000000000000000, 0.000000000000000000, 0.000000000000000000 ) ) ;
#38240=CARTESIAN_POINT ( 'NONE',  ( 7.517309937294106348, -5.180920709765818088, 8.180401817406641740 ) ) ;
#38244=CARTESIAN_POINT ( 'NONE',  ( 11.09999999999999964, -2.700000000000000178, 5.160242730440000258 ) ) ;
#38258=EDGE_CURVE ( 'NONE', #67742, #65964, #29578, .T. ) ;
#38261=CARTESIAN_POINT ( 'NONE',  ( 9.906851002540999929, -2.832432432432000269, -6.822293592207000934 ) ) ;
#38265=CARTESIAN_POINT ( 'NONE',  ( 10.90374822854000136, -3.726845778959999578, 5.900452123196999743 ) ) ;
#38270=CARTESIAN_POINT ( 'NONE',  ( 10.38725444037999956, -2.888666857901000196, -6.716331201355000502 ) ) ;
#38271=ORIENTED_EDGE ( 'NONE', *, *, #43349, .F. ) ;
#38280=CARTESIAN_POINT ( 'NONE',  ( 9.339877582927117672, -3.667929758882994218, 9.210246940688463724 ) ) ;
#38283=CARTESIAN_POINT ( 'NONE',  ( 5.599999999407000217, -1.300000000000000044, -9.662944685757000940 ) ) ;
#38288=CARTESIAN_POINT ( 'NONE',  ( 11.08492081570999943, -3.668392767032000013, 5.558160538745999801 ) ) ;
#38298=CARTESIAN_POINT ( 'NONE',  ( 9.026933059621999433, -4.852736108563000528, 8.683927195503999386 ) ) ;
#38312=CARTESIAN_POINT ( 'NONE',  ( 8.032370559622998840, -3.524751762020000179, 5.573845465339999805 ) ) ;
#38330=CARTESIAN_POINT ( 'NONE',  ( 8.380713240912069040, -2.878415775774842533, 8.829883092763182617 ) ) ;
#38341=CARTESIAN_POINT ( 'NONE',  ( 10.54640350404223526, -2.480438647385216022, -8.419559847284382670 ) ) ;
#38342=EDGE_CURVE ( 'NONE', #50218, #25777, #2977, .T. ) ;
#38374=CARTESIAN_POINT ( 'NONE',  ( 9.741009892375998902, -3.588529236307000048, -8.800227248412999970 ) ) ;
#38385=CIRCLE ( 'NONE', #20518, 1.350000000000000533 ) ;
#38410=CARTESIAN_POINT ( 'NONE',  ( 9.924739995124999936, -5.060461104229999840, 8.686133300732999274 ) ) ;
#38416=CARTESIAN_POINT ( 'NONE',  ( 11.11478185320999934, -2.548220588762000194, -8.356740464335999263 ) ) ;
#38417=CARTESIAN_POINT ( 'NONE',  ( 7.898434181710118906, -2.601011730887146989, 8.533201786423413537 ) ) ;
#38418=CARTESIAN_POINT ( 'NONE',  ( 9.285188841453999586, -5.269672295101000437, 8.747824102203999530 ) ) ;
#38432=EDGE_CURVE ( 'NONE', #11189, #10274, #57999, .T. ) ;
#38438=CARTESIAN_POINT ( 'NONE',  ( 8.560879440379000727, -4.228293421747000735, 8.941387937291999322 ) ) ;
#38441=CARTESIAN_POINT ( 'NONE',  ( 10.08525341940465303, -2.214675259024396770, -7.596661910983709021 ) ) ;
#38443=CARTESIAN_POINT ( 'NONE',  ( 10.79702055961999818, -5.792859009854000263, -7.049265738992000152 ) ) ;
#38456=CARTESIAN_POINT ( 'NONE',  ( 8.228368194306998618, -4.806758213702000404, 6.177034600996000435 ) ) ;
#38464=CARTESIAN_POINT ( 'NONE',  ( 7.734298960010000279, -9.034081823845999892, -5.540645505838000417 ) ) ;
#38477=ORIENTED_EDGE ( 'NONE', *, *, #8071, .F. ) ;
#38498=PLANE ( 'NONE',  #634 ) ;
#38507=CARTESIAN_POINT ( 'NONE',  ( 10.31966935320999923, -4.764591648058999596, -5.997654637741999473 ) ) ;
#38508=CARTESIAN_POINT ( 'NONE',  ( 7.000000000000000000, 0.5292307692307999245, -2.083846153846000249 ) ) ;
#38509=CARTESIAN_POINT ( 'NONE',  ( 9.309135711596999485, -5.864995026133001055, -7.324074232821000230 ) ) ;
#38524=B_SPLINE_CURVE_WITH_KNOTS ( 'NONE', 3,
 ( #8888, #36142, #68284, #20404, #46297 ),
 .UNSPECIFIED., .F., .F.,
 ( 4, 1, 4 ),
 ( 0.000000000000000000, 0.5000000000000000000, 1.000000000000000000 ),
 .UNSPECIFIED. ) ;
#38529=CARTESIAN_POINT ( 'NONE',  ( 10.51140025105000042, -2.326718149302000160, -7.741209600718000239 ) ) ;
#38538=EDGE_CURVE ( 'NONE', #67391, #7601, #24148, .T. ) ;
#38543=CARTESIAN_POINT ( 'NONE',  ( 10.18239901426000138, -2.607725299334000102, 7.783410967795999724 ) ) ;
#38554=CARTESIAN_POINT ( 'NONE',  ( 11.19120431613999855, -3.005395205805000192, -6.023553580263000029 ) ) ;
#38558=FACE_OUTER_BOUND ( 'NONE', #46484, .T. ) ;
#38565=FACE_OUTER_BOUND ( 'NONE', #69076, .T. ) ;
#38568=CARTESIAN_POINT ( 'NONE',  ( 10.77462219945999955, -5.575466189878000911, 8.682669263022999573 ) ) ;
#38573=CARTESIAN_POINT ( 'NONE',  ( 9.509907746701999898, -5.077451867123000007, 8.469011304701000498 ) ) ;
#38576=CONICAL_SURFACE ( 'NONE', #9370, 0.8999999994071996579, 0.7853981633972997312 ) ;
#38592=CARTESIAN_POINT ( 'NONE',  ( 7.725062132959652494, -2.650631715052233162, 7.500008390440855877 ) ) ;
#38594=CARTESIAN_POINT ( 'NONE',  ( 9.940795537695231943, -5.100000000000000533, 6.662590550615205665 ) ) ;
#38599=VECTOR ( 'NONE', #47008, 1000.000000000000000 ) ;
#38600=EDGE_CURVE ( 'NONE', #42097, #7255, #13667, .T. ) ;
#38604=DIRECTION ( 'NONE',  ( 0.000000000000000000, 1.000000000000000000, 0.000000000000000000 ) ) ;
#38612=CARTESIAN_POINT ( 'NONE',  ( 9.933536308083233735, -2.899999999999999911, -6.665341197415429519 ) ) ;
#38614=ORIENTED_EDGE ( 'NONE', *, *, #29372, .T. ) ;
#38615=CARTESIAN_POINT ( 'NONE',  ( 10.37874387220000116, -4.882732524430000609, 6.350796477317000921 ) ) ;
#38620=CARTESIAN_POINT ( 'NONE',  ( 11.22022944037999892, -3.883088694641999794, -8.854817792072001481 ) ) ;
#38637=CARTESIAN_POINT ( 'NONE',  ( 9.285188841453999586, -5.269672295101000437, 8.747824102203999530 ) ) ;
#38646=CARTESIAN_POINT ( 'NONE',  ( 7.277749419310966417, -2.920727118723208005, 6.671122885330429853 ) ) ;
#38648=B_SPLINE_CURVE_WITH_KNOTS ( 'NONE', 3,
 ( #66651, #19101, #50234, #65611 ),
 .UNSPECIFIED., .F., .F.,
 ( 4, 4 ),
 ( 0.000000000000000000, 1.000000000000000000 ),
 .UNSPECIFIED. ) ;
#38649=CARTESIAN_POINT ( 'NONE',  ( 8.475644353210000759, -5.095088356574999366, 6.286978111459999852 ) ) ;
#38652=CARTESIAN_POINT ( 'NONE',  ( 10.96866170142999941, -5.808833653407999620, 4.931298558683999467 ) ) ;
#38664=CARTESIAN_POINT ( 'NONE',  ( 9.294724726289000927, -4.148132978932999926, 9.337467253566000380 ) ) ;
#38678=CARTESIAN_POINT ( 'NONE',  ( 8.424688440789097399, -5.350083765069893360, 7.500019236172019710 ) ) ;
#38683=CARTESIAN_POINT ( 'NONE',  ( 8.558667133076065525, -3.651697308196094838, 5.795658283814029588 ) ) ;
#38687=CARTESIAN_POINT ( 'NONE',  ( 10.02314899745999988, -5.167567567567999731, -6.822293592207000934 ) ) ;
#38696=CARTESIAN_POINT ( 'NONE',  ( 10.38344113585631412, -5.519338294115820887, -8.419368937664973629 ) ) ;
#38697=FACE_OUTER_BOUND ( 'NONE', #26069, .T. ) ;
#38701=VERTEX_POINT ( 'NONE', #57327 ) ;
#38719=ORIENTED_EDGE ( 'NONE', *, *, #62642, .T. ) ;
#38725=CARTESIAN_POINT ( 'NONE',  ( 10.53865751177000121, -3.647233463439000012, -6.014125921456000334 ) ) ;
#38733=LINE ( 'NONE', #12510, #8648 ) ;
#38744=CARTESIAN_POINT ( 'NONE',  ( 7.988543146792999927, -3.566638198986999964, 5.743608852252999775 ) ) ;
#38745=CARTESIAN_POINT ( 'NONE',  ( 10.06233042975999936, -5.062748727288000516, -8.618689820632001286 ) ) ;
#38746=ADVANCED_FACE ( 'NONE', ( #36709 ), #50779, .F. ) ;
#38756=CARTESIAN_POINT ( 'NONE',  ( 9.832537864288001472, -2.899999999999999911, 6.571291218949999902 ) ) ;
#38758=ORIENTED_EDGE ( 'NONE', *, *, #39534, .F. ) ;
#38763=CARTESIAN_POINT ( 'NONE',  ( 10.51654446536000087, -4.930670681812999945, 8.573593359022000371 ) ) ;
#38766=CARTESIAN_POINT ( 'NONE',  ( 8.960616452296999768, -2.899999999999999911, 6.279946362737000243 ) ) ;
#38769=CARTESIAN_POINT ( 'NONE',  ( 10.90246814679000131, -4.554787328265999413, -6.081873034041000103 ) ) ;
#38770=CARTESIAN_POINT ( 'NONE',  ( 7.806861305538506102, -4.389447504349804241, 9.195466472809515679 ) ) ;
#38771=CARTESIAN_POINT ( 'NONE',  ( 11.27109998545999936, -5.469594811916000054, 8.504700858852999090 ) ) ;
#38772=CARTESIAN_POINT ( 'NONE',  ( 10.17500046684972936, -2.650307855384914202, 7.500001770945068813 ) ) ;
#38777=ORIENTED_EDGE ( 'NONE', *, *, #1278, .F. ) ;
#38785=AXIS2_PLACEMENT_3D ( 'NONE', #18138, #27591, #64635 ) ;
#38786=CARTESIAN_POINT ( 'NONE',  ( 11.09999999999999964, -4.000000000000000000, -7.500000000000000000 ) ) ;
#38788=CYLINDRICAL_SURFACE ( 'NONE', #26946, 0.4999999999999998335 ) ;
#38791=CARTESIAN_POINT ( 'NONE',  ( 10.96226112747999970, -2.399999999999999911, -6.571291218949999902 ) ) ;
#38797=CARTESIAN_POINT ( 'NONE',  ( 5.700000000124999744, 0.5292307632381000326, -2.083846155497000030 ) ) ;
#38801=EDGE_CURVE ( 'NONE', #48331, #22433, #39593, .T. ) ;
#38802=FACE_OUTER_BOUND ( 'NONE', #899, .T. ) ;
#38807=CARTESIAN_POINT ( 'NONE',  ( 10.61503919148196218, -5.349978903665073560, -7.499997722305344006 ) ) ;
#38820=CARTESIAN_POINT ( 'NONE',  ( 8.351726203237999968, -5.100872937112000294, 6.601389982007999535 ) ) ;
#38844=VECTOR ( 'NONE', #41174, 1000.000000000000000 ) ;
#38858=CIRCLE ( 'NONE', #66797, 0.5000000000000001110 ) ;
#38859=FACE_OUTER_BOUND ( 'NONE', #53303, .T. ) ;
#38867=CARTESIAN_POINT ( 'NONE',  ( 10.81188185321000006, -4.614147550108000928, -5.930138617968999881 ) ) ;
#38872=CARTESIAN_POINT ( 'NONE',  ( 10.99600479835999955, -8.064994891046000092, -6.834771013433999620 ) ) ;
#38885=CARTESIAN_POINT ( 'NONE',  ( 10.99479839230999900, -3.850614833844999918, -9.347951988117998212 ) ) ;
#38888=CARTESIAN_POINT ( 'NONE',  ( 10.52209773956086458, -3.051556286204309743, -5.005589990389688104 ) ) ;
#38894=CARTESIAN_POINT ( 'NONE',  ( 10.28599623668000085, -4.700321302673000190, 5.006347807457999899 ) ) ;
#38898=CARTESIAN_POINT ( 'NONE',  ( 9.479212726990999371, -4.071727350623000063, 9.089303488377000306 ) ) ;
#38910=CARTESIAN_POINT ( 'NONE',  ( 10.56270535986999981, -2.509383044034000143, -8.602408326857998944 ) ) ;
#38912=CARTESIAN_POINT ( 'NONE',  ( 7.877465178218598041, -5.139684893972532365, 6.768899977688172420 ) ) ;
#38927=CARTESIAN_POINT ( 'NONE',  ( 9.657547180956999711, -5.333447643521000536, 6.049925825719999928 ) ) ;
#38930=CARTESIAN_POINT ( 'NONE',  ( 9.634027193201999850, -3.042970193091000031, 8.588108172435999776 ) ) ;
#38932=DIRECTION ( 'NONE',  ( 9.901258578469000068E-11, -9.901224327269000045E-11, -1.000000000000000000 ) ) ;
#38946=DIRECTION ( 'NONE',  ( 0.000000000000000000, 1.000000000000000000, 0.000000000000000000 ) ) ;
#38963=CARTESIAN_POINT ( 'NONE',  ( 9.059370559623998176, -4.192917962110999319, 5.525484568403999930 ) ) ;
#38968=CARTESIAN_POINT ( 'NONE',  ( 10.93333333333530710, -5.319670837134319541, 7.972931767323275132 ) ) ;
#38975=CARTESIAN_POINT ( 'NONE',  ( 11.33381694038000020, -2.642393655627000015, -7.577897390831000557 ) ) ;
#38979=LINE ( 'NONE', #60297, #63731 ) ;
#38985=VERTEX_POINT ( 'NONE', #43504 ) ;
#38991=CARTESIAN_POINT ( 'NONE',  ( 10.58844302970999962, -3.754658547780000521, 5.545362468768000319 ) ) ;
#38995=ORIENTED_EDGE ( 'NONE', *, *, #30478, .F. ) ;
#39002=EDGE_CURVE ( 'NONE', #7917, #40162, #60800, .T. ) ;
#39003=EDGE_CURVE ( 'NONE', #34244, #2041, #63433, .T. ) ;
#39004=CARTESIAN_POINT ( 'NONE',  ( 8.283081853209001366, -2.376522687267000222, 7.686981355459999499 ) ) ;
#39010=CARTESIAN_POINT ( 'NONE',  ( 7.000000000000000000, -0.2897247358851999799, -3.000000000000000000 ) ) ;
#39021=CARTESIAN_POINT ( 'NONE',  ( 10.30204095393061081, -2.650238144765123760, -7.719132294906671632 ) ) ;
#39026=CARTESIAN_POINT ( 'NONE',  ( 8.610875063856999745, -4.757997781751000410, 5.934102420827000124 ) ) ;
#39047=CARTESIAN_POINT ( 'NONE',  ( 6.750663127261000263, -9.312586504099000351, 5.427957373207999758 ) ) ;
#39052=ORIENTED_EDGE ( 'NONE', *, *, #15529, .T. ) ;
#39062=DIRECTION ( 'NONE',  ( 0.000000000000000000, 1.000000000000000000, 0.000000000000000000 ) ) ;
#39072=CARTESIAN_POINT ( 'NONE',  ( 9.766127544684000128, -4.735430008785999512, -8.791396910319001279 ) ) ;
#39073=DIRECTION ( 'NONE',  ( 1.000000000000000000, 0.000000000000000000, 0.000000000000000000 ) ) ;
#39075=CARTESIAN_POINT ( 'NONE',  ( 8.383148997457999130, -5.167567567567999731, 6.822293592207000934 ) ) ;
#39076=B_SPLINE_CURVE_WITH_KNOTS ( 'NONE', 3,
 ( #35901, #18457, #57217, #39780 ),
 .UNSPECIFIED., .F., .F.,
 ( 4, 4 ),
 ( 0.000000000000000000, 1.000000000000000000 ),
 .UNSPECIFIED. ) ;
#39091=CARTESIAN_POINT ( 'NONE',  ( 8.785191940379998954, -5.414909314743000301, 8.890670256079998168 ) ) ;
#39092=CARTESIAN_POINT ( 'NONE',  ( 10.18225119159999892, -4.505165106450999879, -8.732017808253001334 ) ) ;
#39094=CARTESIAN_POINT ( 'NONE',  ( 11.09999999999999964, -2.646159083949000124, 6.745271721726000536 ) ) ;
#39099=EDGE_CURVE ( 'NONE', #31558, #16664, #47717, .T. ) ;
#39107=CARTESIAN_POINT ( 'NONE',  ( 9.520803773887999810, -3.270557529354000348, 5.711489293131999823 ) ) ;
#39108=CARTESIAN_POINT ( 'NONE',  ( 9.026933059621999433, -4.852736108563000528, 8.683927195503999386 ) ) ;
#39112=CARTESIAN_POINT ( 'NONE',  ( 10.08211398012999993, -4.728049789772000189, -8.793977405422999993 ) ) ;
#39114=CARTESIAN_POINT ( 'NONE',  ( 8.062962586773856799, -3.740282130435375496, 5.779432715689869937 ) ) ;
#39115=CARTESIAN_POINT ( 'NONE',  ( 9.104016254283999743, -5.045864843302999780, 8.527867871227000407 ) ) ;
#39116=CARTESIAN_POINT ( 'NONE',  ( 9.928735088624382144, -5.349822375552029108, 7.563678388627733007 ) ) ;
#39126=DIRECTION ( 'NONE',  ( 0.000000000000000000, 0.000000000000000000, -1.000000000000000000 ) ) ;
#39131=CARTESIAN_POINT ( 'NONE',  ( 7.983191940377000861, -5.321924421352999701, 8.118250081378000971 ) ) ;
#39136=CARTESIAN_POINT ( 'NONE',  ( 10.34267055962000015, -5.750479631840000216, -8.094412205797999249 ) ) ;
#39140=CARTESIAN_POINT ( 'NONE',  ( 8.204580816340637739, -2.648164948733253699, 7.853008025111919643 ) ) ;
#39157=B_SPLINE_CURVE_WITH_KNOTS ( 'NONE', 3,
 ( #64183, #26108, #5469, #43217 ),
 .UNSPECIFIED., .F., .F.,
 ( 4, 4 ),
 ( 0.000000000000000000, 1.000000000000000000 ),
 .UNSPECIFIED. ) ;
#39161=ORIENTED_EDGE ( 'NONE', *, *, #45404, .T. ) ;
#39176=CARTESIAN_POINT ( 'NONE',  ( 7.790629440376999781, -3.416208448044999901, 6.162501393933999871 ) ) ;
#39187=EDGE_CURVE ( 'NONE', #42842, #34621, #57003, .T. ) ;
#39196=CARTESIAN_POINT ( 'NONE',  ( 7.383137037416592996, -2.829917722523448642, 8.817307441672506130 ) ) ;
#39201=AXIS2_PLACEMENT_3D ( 'NONE', #29025, #8713, #40866 ) ;
#39207=CARTESIAN_POINT ( 'NONE',  ( 11.33381694038000020, -2.642393655627000015, -7.577897390831000557 ) ) ;
#39209=DIRECTION ( 'NONE',  ( 5.369763710129195918E-06, 0.9999999999350365210, -1.005448450480035185E-05 ) ) ;
#39213=ORIENTED_EDGE ( 'NONE', *, *, #43025, .F. ) ;
#39225=CARTESIAN_POINT ( 'NONE',  ( 10.38153277269999997, -2.772136814285999673, -8.408084799892998618 ) ) ;
#39228=EDGE_CURVE ( 'NONE', #63228, #11689, #66159, .T. ) ;
#39230=VERTEX_POINT ( 'NONE', #14450 ) ;
#39233=CARTESIAN_POINT ( 'NONE',  ( 10.57161764893999845, -5.198524786722999558, 4.692090250997000389 ) ) ;
#39234=B_SPLINE_CURVE_WITH_KNOTS ( 'NONE', 3,
 ( #22130, #28077, #43471, #30157 ),
 .UNSPECIFIED., .F., .F.,
 ( 4, 4 ),
 ( 0.000000000000000000, 1.000000000000000000 ),
 .UNSPECIFIED. ) ;
#39238=CARTESIAN_POINT ( 'NONE',  ( 10.76010362286999822, -4.535387425205000156, 6.001717576299999024 ) ) ;
#39244=CARTESIAN_POINT ( 'NONE',  ( 10.45187389798759270, -5.320777371542467549, 7.955754976780856857 ) ) ;
#39251=CARTESIAN_POINT ( 'NONE',  ( 11.07336076184000007, -2.375557098086999996, -8.393541296344000813 ) ) ;
#39252=CARTESIAN_POINT ( 'NONE',  ( 6.960892430994999991, -9.225317279141998839, -5.198338520859000056 ) ) ;
#39253=AXIS2_PLACEMENT_3D ( 'NONE', #32194, #53508, #5598 ) ;
#39256=CARTESIAN_POINT ( 'NONE',  ( 9.304144223516997769, -2.772050158355999994, -8.125211791007998841 ) ) ;
#39264=CARTESIAN_POINT ( 'NONE',  ( 10.91901409926999911, -2.752141321853000200, 4.977018749245999629 ) ) ;
#39265=CARTESIAN_POINT ( 'NONE',  ( 8.221178267935991713, -3.443155653785000769, 6.131664341583003441 ) ) ;
#39266=VERTEX_POINT ( 'NONE', #15129 ) ;
#39268=CARTESIAN_POINT ( 'NONE',  ( 9.034116535116000435, -4.695350938297000454, 8.660677768253002284 ) ) ;
#39271=CARTESIAN_POINT ( 'NONE',  ( 9.166075977534999808, -4.023333687735000552, 9.122281080215000060 ) ) ;
#39272=ADVANCED_FACE ( 'NONE', ( #67914 ), #41358, .T. ) ;
#39280=CARTESIAN_POINT ( 'NONE',  ( 9.189494650919995067, -2.900751414380998039, -6.630304163275999585 ) ) ;
#39286=CARTESIAN_POINT ( 'NONE',  ( 9.685492310842999331, -4.505165106450999879, -8.732017808253001334 ) ) ;
#39289=LINE ( 'NONE', #12721, #3118 ) ;
#39301=CARTESIAN_POINT ( 'NONE',  ( 8.353308059623998361, -2.800111029801999774, 9.079936276749000612 ) ) ;
#39308=CARTESIAN_POINT ( 'NONE',  ( 10.75110221171000013, -2.822135527917999820, 6.655890318096999714 ) ) ;
#39324=FACE_OUTER_BOUND ( 'NONE', #50656, .T. ) ;
#39329=CARTESIAN_POINT ( 'NONE',  ( 10.97053692116999990, -5.147214819045999867, -5.024239345603000118 ) ) ;
#39333=CARTESIAN_POINT ( 'NONE',  ( 11.20904026220999938, -5.937811873294999820, 7.147336919140999001 ) ) ;
#39335=CARTESIAN_POINT ( 'NONE',  ( 7.717562990494335473, -2.846244519028975795, 6.797277674502598011 ) ) ;
#39340=CARTESIAN_POINT ( 'NONE',  ( 10.56498513754060653, -5.349957030113857925, -7.500000808964294663 ) ) ;
#39342=CARTESIAN_POINT ( 'NONE',  ( 8.641808059624999316, -2.933824946949000090, 8.496487880080000110 ) ) ;
#39345=CARTESIAN_POINT ( 'NONE',  ( 10.96507314189000049, -6.669294869020999883, 5.364414917161000496 ) ) ;
#39357=DIRECTION ( 'NONE',  ( 1.000000000000000000, -3.552713678852000294E-14, -5.329070518279000085E-14 ) ) ;
#39360=CARTESIAN_POINT ( 'NONE',  ( 8.046447522772005811, -5.096470895078004659, 6.454903582004997808 ) ) ;
#39371=EDGE_LOOP ( 'NONE', ( #56110, #69037, #9281, #28334 ) ) ;
#39381=CARTESIAN_POINT ( 'NONE',  ( 9.468462140533970839, -5.148144707188508029, 8.212636205154785429 ) ) ;
#39386=CARTESIAN_POINT ( 'NONE',  ( 8.883148997460001084, -5.167567567567999731, 6.822293592207000934 ) ) ;
#39388=CARTESIAN_POINT ( 'NONE',  ( 8.455992358812000731, -5.100000000000000533, 6.571291218949999902 ) ) ;
#39408=ORIENTED_EDGE ( 'NONE', *, *, #53264, .T. ) ;
#39416=CARTESIAN_POINT ( 'NONE',  ( 10.89218817467000200, -2.661900611977999986, -8.236035141896001832 ) ) ;
#39417=DIRECTION ( 'NONE',  ( 0.000000000000000000, -0.1333333333333049098, 0.9910712498212373989 ) ) ;
#39435=CARTESIAN_POINT ( 'NONE',  ( 8.245293146793999384, -4.282999948634999221, 9.286791354293999490 ) ) ;
#39441=B_SPLINE_CURVE_WITH_KNOTS ( 'NONE', 3,
 ( #53308, #59232, #1205, #6091 ),
 .UNSPECIFIED., .F., .F.,
 ( 4, 4 ),
 ( 0.000000000000000000, 1.000000000000000000 ),
 .UNSPECIFIED. ) ;
#39453=CARTESIAN_POINT ( 'NONE',  ( 9.332935524889000689, -5.100347267927999972, 8.693464469215999912 ) ) ;
#39454=CARTESIAN_POINT ( 'NONE',  ( 8.385058059625000837, -4.977917894183000236, 6.416767031887000705 ) ) ;
#39458=CARTESIAN_POINT ( 'NONE',  ( 8.083009592828254597, -4.188654535187550820, 5.770339112206491983 ) ) ;
#39460=CARTESIAN_POINT ( 'NONE',  ( 11.18051369187999988, -5.340070732632000272, 8.416150632189001612 ) ) ;
#39463=ORIENTED_EDGE ( 'NONE', *, *, #28985, .T. ) ;
#39476=EDGE_CURVE ( 'NONE', #49363, #33712, #33740, .T. ) ;
#39481=CARTESIAN_POINT ( 'NONE',  ( 8.443894353209000059, -2.905864338704999827, 8.940687151810998046 ) ) ;
#39486=CARTESIAN_POINT ( 'NONE',  ( 10.94847055962000049, -3.841065069379000274, -9.341805385095000247 ) ) ;
#39495=ORIENTED_EDGE ( 'NONE', *, *, #59648, .F. ) ;
#39510=CARTESIAN_POINT ( 'NONE',  ( 11.09999999999999964, -5.449702618175999547, 5.124965750789000296 ) ) ;
#39518=ORIENTED_EDGE ( 'NONE', *, *, #17034, .F. ) ;
#39523=CARTESIAN_POINT ( 'NONE',  ( 8.239941940377999430, -2.735207418315000361, 6.771977475428999860 ) ) ;
#39524=FACE_OUTER_BOUND ( 'NONE', #17718, .T. ) ;
#39530=CARTESIAN_POINT ( 'NONE',  ( 9.832537864288001472, -2.899999999999999911, 6.571291218949999902 ) ) ;
#39532=DIRECTION ( 'NONE',  ( 0.000000000000000000, -1.000000000000000000, 0.000000000000000000 ) ) ;
#39534=EDGE_CURVE ( 'NONE', #66560, #24689, #7854, .T. ) ;
#39544=CARTESIAN_POINT ( 'NONE',  ( 7.423512759997511701, -2.354253581828240627, 8.063754798790684575 ) ) ;
#39545=CARTESIAN_POINT ( 'NONE',  ( 10.57960558317873279, -4.353252721116731117, 8.851706718789644768 ) ) ;
#39553=CARTESIAN_POINT ( 'NONE',  ( 10.80374194038000013, -2.766944173105999827, -8.073385940268000383 ) ) ;
#39563=CARTESIAN_POINT ( 'NONE',  ( 8.968532939428907724, -5.344941310868764006, 7.382699998430346078 ) ) ;
#39572=CARTESIAN_POINT ( 'NONE',  ( 10.78636854442000192, -5.666037955714999796, -7.787004779180999314 ) ) ;
#39573=CARTESIAN_POINT ( 'NONE',  ( 9.934999999999998721, -4.640430492595999823, -9.117542781427999898 ) ) ;
#39574=CARTESIAN_POINT ( 'NONE',  ( 10.69003253712258505, -2.945770442954086299, -5.060380188079816044 ) ) ;
#39583=CARTESIAN_POINT ( 'NONE',  ( 9.924739995124999936, -5.060461104229999840, 8.686133300732999274 ) ) ;
#39586=CARTESIAN_POINT ( 'NONE',  ( 6.799999999999999822, -9.295462635088998837, -5.399710584805999858 ) ) ;
#39590=LINE ( 'NONE', #60913, #48538 ) ;
#39593=CIRCLE ( 'NONE', #35155, 1.350000000000000533 ) ;
#39601=CARTESIAN_POINT ( 'NONE',  ( 9.348145925901000908, -2.626678530444999993, -7.387134320497999340 ) ) ;
#39609=CARTESIAN_POINT ( 'NONE',  ( 10.94076550314999885, -5.140765503144999471, -6.571291218949999902 ) ) ;
#39612=VECTOR ( 'NONE', #67226, 1000.000000000000114 ) ;
#39613=CARTESIAN_POINT ( 'NONE',  ( 10.06343867337000120, -5.156226070197000411, 6.125223053176999777 ) ) ;
#39618=CARTESIAN_POINT ( 'NONE',  ( 9.137549407199999862, -2.995696424181999884, 8.544763501938000161 ) ) ;
#39628=CARTESIAN_POINT ( 'NONE',  ( 8.393806199904998877, -2.909809943507001950, -6.638007308765000225 ) ) ;
#39632=CARTESIAN_POINT ( 'NONE',  ( 9.101385834542000453, -4.783349162191000481, -6.231236652334000148 ) ) ;
#39634=ORIENTED_EDGE ( 'NONE', *, *, #577, .T. ) ;
#39639=EDGE_CURVE ( 'NONE', #2324, #17007, #55818, .T. ) ;
#39653=CARTESIAN_POINT ( 'NONE',  ( 9.264236589623052964, -4.933094564478333943, -6.039157063336917375 ) ) ;
#39656=CARTESIAN_POINT ( 'NONE',  ( 9.882266086202999844, -4.932716797830999589, 6.390980246320999925 ) ) ;
#39672=CARTESIAN_POINT ( 'NONE',  ( 9.419101312255003577, -2.376585296233752143, 8.156356589247646838 ) ) ;
#39674=CARTESIAN_POINT ( 'NONE',  ( 8.281500452969403625, -5.066926970486362869, 6.455544745802533235 ) ) ;
#39679=CARTESIAN_POINT ( 'NONE',  ( 10.96580795178999956, -4.930647899304999804, 6.170539049947000088 ) ) ;
#39682=B_SPLINE_CURVE_WITH_KNOTS ( 'NONE', 3,
 ( #10354, #43559, #48454, #562, #26795 ),
 .UNSPECIFIED., .F., .F.,
 ( 4, 1, 4 ),
 ( 0.000000000000000000, 0.5000000000000000000, 1.000000000000000000 ),
 .UNSPECIFIED. ) ;
#39691=CARTESIAN_POINT ( 'NONE',  ( 7.101308059622001068, -3.554853390786000045, 8.889491623367000273 ) ) ;
#39698=CARTESIAN_POINT ( 'NONE',  ( 10.95489937859999863, -2.662062732762999762, -4.890147771044999203 ) ) ;
#39707=EDGE_CURVE ( 'NONE', #28572, #9350, #1988, .T. ) ;
#39716=ORIENTED_EDGE ( 'NONE', *, *, #15247, .F. ) ;
#39718=CARTESIAN_POINT ( 'NONE',  ( 10.99695204966289630, -2.814806026439112596, 5.073559010014569992 ) ) ;
#39726=CARTESIAN_POINT ( 'NONE',  ( 8.555928920931012982, -3.595744531712468106, 5.807944245245301396 ) ) ;
#39731=FACE_OUTER_BOUND ( 'NONE', #52762, .T. ) ;
#39735=CARTESIAN_POINT ( 'NONE',  ( 9.010191940380000375, -5.040796345420999636, 8.522966281393001609 ) ) ;
#39743=VERTEX_POINT ( 'NONE', #66978 ) ;
#39766=CARTESIAN_POINT ( 'NONE',  ( 11.02205565301999890, -2.309485172892000282, -7.515673712097999726 ) ) ;
#39780=CARTESIAN_POINT ( 'NONE',  ( 9.140753410162000492, -5.100000000000000533, 6.175944241622000064 ) ) ;
#39784=CARTESIAN_POINT ( 'NONE',  ( 7.629816940376999312, -4.763531818439999732, 5.668890958491999754 ) ) ;
#39800=CARTESIAN_POINT ( 'NONE',  ( 9.242349231304000767, -5.206700957550999931, 8.808818370147001531 ) ) ;
#39806=CARTESIAN_POINT ( 'NONE',  ( 7.901443686586306470, -2.563629936457297198, 8.480909633787742763 ) ) ;
#39807=CARTESIAN_POINT ( 'NONE',  ( 11.06924082387999952, -5.425685649895999774, 8.012912555523998392 ) ) ;
#39811=VERTEX_POINT ( 'NONE', #60285 ) ;
#39818=CARTESIAN_POINT ( 'NONE',  ( 10.01832872737000102, -5.491975933468000726, -7.893788029530999673 ) ) ;
#39829=CARTESIAN_POINT ( 'NONE',  ( 7.481081853206999810, -2.374041291348000016, 8.293390875797999939 ) ) ;
#39834=CARTESIAN_POINT ( 'NONE',  ( 9.964045559621999004, -3.485908552077000344, -9.275738075927998594 ) ) ;
#39837=CARTESIAN_POINT ( 'NONE',  ( 7.550000000000000711, -4.000000000000000000, 8.849999999999999645 ) ) ;
#39845=CARTESIAN_POINT ( 'NONE',  ( 10.89999568968999988, -1.433323842147000038, -10.65402156160000047 ) ) ;
#39846=CARTESIAN_POINT ( 'NONE',  ( 10.58718478751724312, -5.286440948693045705, -7.026985308887813808 ) ) ;
#39850=EDGE_CURVE ( 'NONE', #2231, #664, #56130, .T. ) ;
#39855=CARTESIAN_POINT ( 'NONE',  ( 9.129428851719998406, -5.099284414202999827, 6.151604790022999758 ) ) ;
#39874=ADVANCED_FACE ( 'NONE', ( #1904 ), #50830, .T. ) ;
#39876=CARTESIAN_POINT ( 'NONE',  ( 7.726441940376999717, -2.630475685621000093, 6.995953627589999613 ) ) ;
#39889=DIRECTION ( 'NONE',  ( 1.000000000000000000, 0.000000000000000000, 0.000000000000000000 ) ) ;
#39891=ORIENTED_EDGE ( 'NONE', *, *, #29374, .F. ) ;
#39894=CARTESIAN_POINT ( 'NONE',  ( 7.395800130882417278, -2.637111068654788060, 8.607766089379190078 ) ) ;
#39899=CARTESIAN_POINT ( 'NONE',  ( 8.620740978634000129, -4.599999999999999645, 5.898823289756999877 ) ) ;
#39904=CARTESIAN_POINT ( 'NONE',  ( 9.549696181504765846, -3.998651493754463271, 8.867000060670704897 ) ) ;
#39922=CARTESIAN_POINT ( 'NONE',  ( 9.972537864286000087, -2.899999999999999911, -6.571291218949999902 ) ) ;
#39923=CARTESIAN_POINT ( 'NONE',  ( 9.569799020577001158, -4.064052785562999759, 8.919253808370999792 ) ) ;
#39926=CARTESIAN_POINT ( 'NONE',  ( 10.36629943602999937, -5.852732332139999549, -7.568014220767000033 ) ) ;
#39928=CARTESIAN_POINT ( 'NONE',  ( 10.74230018269611797, -2.926900783495216096, -5.077338026010398409 ) ) ;
#39931=DIRECTION ( 'NONE',  ( 0.000000000000000000, 1.000000000000000000, 0.000000000000000000 ) ) ;
#39932=CARTESIAN_POINT ( 'NONE',  ( 10.80457650502840927, -2.650115154242059123, -7.676668932391375044 ) ) ;
#39934=EDGE_CURVE ( 'NONE', #438, #28572, #4685, .T. ) ;
#39937=CARTESIAN_POINT ( 'NONE',  ( 9.722771884505998941, -5.493781611190000191, 6.566828939965000167 ) ) ;
#39941=ORIENTED_EDGE ( 'NONE', *, *, #577, .F. ) ;
#39943=DIRECTION ( 'NONE',  ( 0.000000000000000000, 0.8648648648648720183, -0.5020047465136825426 ) ) ;
#39951=CARTESIAN_POINT ( 'NONE',  ( 11.09999999999999964, -4.000000000000000000, 7.500000000000000000 ) ) ;
#39952=AXIS2_PLACEMENT_3D ( 'NONE', #51815, #57400, #56387 ) ;
#39955=CARTESIAN_POINT ( 'NONE',  ( 9.568154437819998748, -5.318469253323000245, -7.099528416287999910 ) ) ;
#39961=CARTESIAN_POINT ( 'NONE',  ( 11.14011782775999926, -2.672921762942999990, 4.984811564083999613 ) ) ;
#39966=CARTESIAN_POINT ( 'NONE',  ( 9.709999999999999076, -4.496968146123999865, -8.755198255949000696 ) ) ;
#39967=CARTESIAN_POINT ( 'NONE',  ( 9.939319226872999735, -2.638101016021999978, 6.328632621050000573 ) ) ;
#39971=CARTESIAN_POINT ( 'NONE',  ( 9.573148997458000409, -5.167567567567999731, -6.822293592207000934 ) ) ;
#39972=FACE_OUTER_BOUND ( 'NONE', #57539, .T. ) ;
#39979=EDGE_CURVE ( 'NONE', #61812, #21138, #4297, .T. ) ;
#39982=CYLINDRICAL_SURFACE ( 'NONE', #37316, 1.100000000000000089 ) ;
#39985=CARTESIAN_POINT ( 'NONE',  ( 9.191972128127998687, -4.867164667115999599, -6.095483598963999938 ) ) ;
#39987=ORIENTED_EDGE ( 'NONE', *, *, #18312, .F. ) ;
#39988=CARTESIAN_POINT ( 'NONE',  ( 9.897088546675218979, -5.285903972627228775, 7.026783966727966124 ) ) ;
#40007=CARTESIAN_POINT ( 'NONE',  ( 8.666729817973333638, -2.899999999999999911, 6.535479089440332956 ) ) ;
#40011=ORIENTED_EDGE ( 'NONE', *, *, #56523, .F. ) ;
#40021=EDGE_CURVE ( 'NONE', #9159, #17467, #25632, .T. ) ;
#40025=CARTESIAN_POINT ( 'NONE',  ( 9.406895376471270609, -2.504060814039583249, 8.387610628396673818 ) ) ;
#40032=CARTESIAN_POINT ( 'NONE',  ( 10.12549839661999940, -5.788806995403000144, 7.335561828691000485 ) ) ;
#40039=CARTESIAN_POINT ( 'NONE',  ( 7.454905163714801830, -5.316162339229765443, 7.145932548772795379 ) ) ;
#40040=CARTESIAN_POINT ( 'NONE',  ( 9.270843198681054886, -5.086512213758866530, 8.869463831023999489 ) ) ;
#40046=CARTESIAN_POINT ( 'NONE',  ( 11.01815802025999957, -5.555209496388000545, 4.991732544280999662 ) ) ;
#40049=CARTESIAN_POINT ( 'NONE',  ( 10.56717786912000001, -2.828865965284999895, 4.740087349777999393 ) ) ;
#40061=CARTESIAN_POINT ( 'NONE',  ( 8.493356027204001180, -5.097500218784999149, 6.607661537772998805 ) ) ;
#40064=CARTESIAN_POINT ( 'NONE',  ( 8.603645510037827293, -4.706833859777778351, 5.918599468013924891 ) ) ;
#40068=CARTESIAN_POINT ( 'NONE',  ( 7.783734131047877369, -2.886512552566496748, 6.705439129923228769 ) ) ;
#40076=CARTESIAN_POINT ( 'NONE',  ( 11.09999999999999964, -5.599999999999999645, -6.571291218949999902 ) ) ;
#40081=ORIENTED_EDGE ( 'NONE', *, *, #38171, .T. ) ;
#40082=CARTESIAN_POINT ( 'NONE',  ( 11.09424907396999949, -2.431867116603999790, 7.769513708858000633 ) ) ;
#40085=CARTESIAN_POINT ( 'NONE',  ( 8.598668146794999245, -2.376522687267000222, 7.686981355459999499 ) ) ;
#40094=CARTESIAN_POINT ( 'NONE',  ( 9.595487457706001422, -3.928425191288000384, 5.531324308465000783 ) ) ;
#40096=DIRECTION ( 'NONE',  ( 1.000000000000000000, 0.000000000000000000, 0.000000000000000000 ) ) ;
#40098=ORIENTED_EDGE ( 'NONE', *, *, #60051, .F. ) ;
#40103=CARTESIAN_POINT ( 'NONE',  ( 9.679055905794999859, -2.899999999999999911, 6.571291218949999902 ) ) ;
#40115=CARTESIAN_POINT ( 'NONE',  ( 10.99479839230999900, -3.850614833844999918, -9.347951988117998212 ) ) ;
#40117=CARTESIAN_POINT ( 'NONE',  ( 9.008370456395944359, -5.237385890216453177, 8.039653529976170887 ) ) ;
#40118=ORIENTED_EDGE ( 'NONE', *, *, #59738, .F. ) ;
#40122=EDGE_CURVE ( 'NONE', #3478, #51145, #21089, .T. ) ;
#40135=CARTESIAN_POINT ( 'NONE',  ( 7.475043146792000215, -3.276313010012999793, 5.841993238691999935 ) ) ;
#40146=CARTESIAN_POINT ( 'NONE',  ( 9.234799632564795857, -4.972103827131938658, -6.117919078289220103 ) ) ;
#40149=CARTESIAN_POINT ( 'NONE',  ( 11.20563089100999932, -3.509133048232999652, 6.118191305996999674 ) ) ;
#40153=CARTESIAN_POINT ( 'NONE',  ( 10.87946694038000039, -2.817416132545000007, -6.828662897514999663 ) ) ;
#40154=CARTESIAN_POINT ( 'NONE',  ( 7.963612997803560134, -2.289570113972569487, 7.184898621721505840 ) ) ;
#40155=CARTESIAN_POINT ( 'NONE',  ( 9.600494040286998043, -5.206548117663999165, 8.585114612872999373 ) ) ;
#40162=VERTEX_POINT ( 'NONE', #37837 ) ;
#40165=CARTESIAN_POINT ( 'NONE',  ( 9.441140818749000019, -4.011292643094999555, -9.373220388412001114 ) ) ;
#40174=CARTESIAN_POINT ( 'NONE',  ( 8.406105646793999853, -5.342173944271999986, 8.432314172168000610 ) ) ;
#40175=DIRECTION ( 'NONE',  ( -1.000000000000000000, 0.000000000000000000, 0.000000000000000000 ) ) ;
#40180=CARTESIAN_POINT ( 'NONE',  ( 10.05463185321000097, -3.531218470783999752, -9.119231780812000920 ) ) ;
#40189=CARTESIAN_POINT ( 'NONE',  ( 8.616995677562000466, -4.876077402042000131, 5.996974966533000106 ) ) ;
#40191=ORIENTED_EDGE ( 'NONE', *, *, #9016, .F. ) ;
#40193=CARTESIAN_POINT ( 'NONE',  ( 8.492064203080353479, -4.378336071229006699, 5.973114860761890910 ) ) ;
#40198=CYLINDRICAL_SURFACE ( 'NONE', #4859, 1.350000000000000089 ) ;
#40213=VERTEX_POINT ( 'NONE', #28396 ) ;
#40216=CARTESIAN_POINT ( 'NONE',  ( 10.85106741697583210, -3.434344919155746023, 9.175967010814426672 ) ) ;
#40217=CARTESIAN_POINT ( 'NONE',  ( 7.892605646791999163, -5.480312458445999901, 8.192326492433998908 ) ) ;
#40226=CARTESIAN_POINT ( 'NONE',  ( 7.000000000000000888, -6.725378844700938608, 3.045375366903437797 ) ) ;
#40231=FACE_OUTER_BOUND ( 'NONE', #34161, .T. ) ;
#40240=CARTESIAN_POINT ( 'NONE',  ( 11.03105082652855984, -2.697932356969752199, -8.692104167685684502 ) ) ;
#40243=CARTESIAN_POINT ( 'NONE',  ( 9.537173706499428860, -4.215401811041904701, 8.849618031277087127 ) ) ;
#40244=CARTESIAN_POINT ( 'NONE',  ( 9.365000000002998704, -2.649999999999999911, -7.500000000000000000 ) ) ;
#40261=CARTESIAN_POINT ( 'NONE',  ( 9.423521818475000700, -4.993993578306000103, 8.578110568283999982 ) ) ;
#40263=CARTESIAN_POINT ( 'NONE',  ( 10.40558062080000035, -5.599331384652000310, -8.437753779290000367 ) ) ;
#40271=CARTESIAN_POINT ( 'NONE',  ( 11.07204542438999972, -6.380876855756000054, -5.350213802198999780 ) ) ;
#40277=CARTESIAN_POINT ( 'NONE',  ( 10.70441271436000008, -3.444516450945999786, 6.009051312948000323 ) ) ;
#40283=CARTESIAN_POINT ( 'NONE',  ( 10.56819717210643361, -5.125396288428698988, -6.749639981086813734 ) ) ;
#40291=CARTESIAN_POINT ( 'NONE',  ( 9.438732219486000830, -2.462132291381999849, -7.373611177161000008 ) ) ;
#40301=CARTESIAN_POINT ( 'NONE',  ( 10.62197618263000010, -5.779779175739000685, 7.256573549370999743 ) ) ;
#40308=ORIENTED_EDGE ( 'NONE', *, *, #5781, .F. ) ;
#40312=CARTESIAN_POINT ( 'NONE',  ( 11.05016464426000056, -2.767526642700999684, 5.012714206629000024 ) ) ;
#40315=ADVANCED_FACE ( 'NONE', ( #26073 ), #60557, .F. ) ;
#40317=CARTESIAN_POINT ( 'NONE',  ( 9.837330429757999539, -5.176458967229000230, -8.738385553646999426 ) ) ;
#40328=CARTESIAN_POINT ( 'NONE',  ( 9.198378269148916431, -4.679948058550536416, -8.679637038427665985 ) ) ;
#40332=CARTESIAN_POINT ( 'NONE',  ( 10.86501009699205866, -2.649983380499685737, -7.500000587580680111 ) ) ;
#40336=CARTESIAN_POINT ( 'NONE',  ( 9.346315804487350221, -5.086028406228472853, -6.305450188067585060 ) ) ;
#40342=EDGE_CURVE ( 'NONE', #33729, #21093, #4387, .T. ) ;
#40345=CARTESIAN_POINT ( 'NONE',  ( 0.000000000000000000, 0.000000000000000000, 0.000000000000000000 ) ) ;
#40353=CARTESIAN_POINT ( 'NONE',  ( 9.354552855434715042, -3.358379027116748183, 9.116748975407924505 ) ) ;
#40356=CARTESIAN_POINT ( 'NONE',  ( 9.921080006317001931, -4.920709323926390155, -9.006083254704995156 ) ) ;
#40360=CARTESIAN_POINT ( 'NONE',  ( 10.93227479887999998, -2.539880901735999785, 6.453614191797999666 ) ) ;
#40364=CARTESIAN_POINT ( 'NONE',  ( 10.93785547196599950, -2.862144528033999880, 6.360512911308666695 ) ) ;
#40366=ORIENTED_EDGE ( 'NONE', *, *, #6042, .F. ) ;
#40379=CARTESIAN_POINT ( 'NONE',  ( 10.02091161619000026, -4.911674715448000050, -6.466751564808000730 ) ) ;
#40388=ORIENTED_EDGE ( 'NONE', *, *, #33792, .F. ) ;
#40395=CARTESIAN_POINT ( 'NONE',  ( 6.799999999999999822, 0.000000000000000000, 0.000000000000000000 ) ) ;
#40396=EDGE_LOOP ( 'NONE', ( #65695, #49316, #29287, #62220 ) ) ;
#40404=CARTESIAN_POINT ( 'NONE',  ( 9.722771884505998941, -5.493781611190000191, 6.566828939965000167 ) ) ;
#40407=CARTESIAN_POINT ( 'NONE',  ( 7.790629440376999781, -3.416208448044999901, 6.162501393933999871 ) ) ;
#40412=CARTESIAN_POINT ( 'NONE',  ( 10.26195629121000152, -4.600000265269999389, 4.591198190832999515 ) ) ;
#40419=CARTESIAN_POINT ( 'NONE',  ( 11.09999999999999964, -5.772457065253999708, -5.146041223417999966 ) ) ;
#40421=LINE ( 'NONE', #29960, #59366 ) ;
#40438=CARTESIAN_POINT ( 'NONE',  ( 10.56270535986999981, -2.509383044034000143, -8.602408326857998944 ) ) ;
#40441=CARTESIAN_POINT ( 'NONE',  ( 9.002566322894800521, -5.272342554236079337, 7.950847953095180998 ) ) ;
#40450=AXIS2_PLACEMENT_3D ( 'NONE', #53180, #57727, #52488 ) ;
#40459=CARTESIAN_POINT ( 'NONE',  ( 8.218894353209000414, -3.011617647609999615, 8.801438026873999121 ) ) ;
#40462=FACE_OUTER_BOUND ( 'NONE', #63849, .T. ) ;
#40463=ORIENTED_EDGE ( 'NONE', *, *, #2355, .T. ) ;
#40468=ORIENTED_EDGE ( 'NONE', *, *, #57294, .T. ) ;
#40471=B_SPLINE_CURVE_WITH_KNOTS ( 'NONE', 3,
 ( #43479, #27392, #60588, #28085 ),
 .UNSPECIFIED., .F., .F.,
 ( 4, 4 ),
 ( 0.000000000000000000, 1.000000000000000000 ),
 .UNSPECIFIED. ) ;
#40476=ORIENTED_EDGE ( 'NONE', *, *, #21303, .F. ) ;
#40477=LINE ( 'NONE', #40822, #5355 ) ;
#40480=CARTESIAN_POINT ( 'NONE',  ( 10.18308064679000147, -2.953580299898999950, -8.606287508253000595 ) ) ;
#40481=CARTESIAN_POINT ( 'NONE',  ( 8.060203937213300307, -3.679481436877252154, 5.790105483359396565 ) ) ;
#40482=CARTESIAN_POINT ( 'NONE',  ( 10.34521071928999980, -2.724119865955000108, 6.497322598008000050 ) ) ;
#40487=CARTESIAN_POINT ( 'NONE',  ( 10.35302581057999838, -4.581018032643999760, -4.861894197833000142 ) ) ;
#40492=CARTESIAN_POINT ( 'NONE',  ( 9.798320215454998205, -2.757678812098000254, -6.584768124342000206 ) ) ;
#40503=CARTESIAN_POINT ( 'NONE',  ( 7.443293146792999693, -4.698358408974000255, 8.789434435623999065 ) ) ;
#40508=CARTESIAN_POINT ( 'NONE',  ( 10.62256935321000029, -2.471463903746000224, -8.210787855397999380 ) ) ;
#40519=SURFACE_STYLE_FILL_AREA ( #25471 ) ;
#40523=B_SPLINE_CURVE_WITH_KNOTS ( 'NONE', 3,
 ( #20816, #25032, #52628, #46364 ),
 .UNSPECIFIED., .F., .F.,
 ( 4, 4 ),
 ( 0.000000000000000000, 0.2180895000437835241 ),
 .UNSPECIFIED. ) ;
#40529=CARTESIAN_POINT ( 'NONE',  ( 10.32340023520112027, -2.820488420190699230, -8.179866073662411807 ) ) ;
#40546=CARTESIAN_POINT ( 'NONE',  ( 10.67395468736628672, -5.666583699971932120, 6.945968662367498325 ) ) ;
#40547=CARTESIAN_POINT ( 'NONE',  ( 8.496691940379001551, -5.198566224659999513, 8.332559954171999905 ) ) ;
#40562=CARTESIAN_POINT ( 'NONE',  ( 9.390726590333203561, -5.236125653078060438, 6.940982610062651048 ) ) ;
#40563=CARTESIAN_POINT ( 'NONE',  ( 7.330275273710999961, -4.426925773067000414, 9.293310812901001583 ) ) ;
#40568=CARTESIAN_POINT ( 'NONE',  ( 7.433994579421323579, -2.292697518400240053, 7.832234419706870732 ) ) ;
#40569=CARTESIAN_POINT ( 'NONE',  ( 10.47530200610951034, -5.350262918594152595, 7.499984559551212904 ) ) ;
#40599=CARTESIAN_POINT ( 'NONE',  ( 9.514108112060000622, -4.887639888682999256, 8.462756667353000140 ) ) ;
#40611=CARTESIAN_POINT ( 'NONE',  ( 10.46754921866999943, -2.318350880468999620, 6.549783596838000044 ) ) ;
#40615=ORIENTED_EDGE ( 'NONE', *, *, #35696, .F. ) ;
#40618=DIRECTION ( 'NONE',  ( 0.7660444431190069903, 0.000000000000000000, 0.6427876096865049460 ) ) ;
#40624=PLANE ( 'NONE',  #40798 ) ;
#40632=ORIENTED_EDGE ( 'NONE', *, *, #28545, .F. ) ;
#40635=CARTESIAN_POINT ( 'NONE',  ( 10.12549839661999940, -5.788806995403000144, 7.335561828691000485 ) ) ;
#40653=CARTESIAN_POINT ( 'NONE',  ( 9.216140818749000374, -4.008306780893000187, -8.877926425468999128 ) ) ;
#40657=AXIS2_PLACEMENT_3D ( 'NONE', #48735, #21805, #65138 ) ;
#40664=ORIENTED_EDGE ( 'NONE', *, *, #20597, .F. ) ;
#40665=CARTESIAN_POINT ( 'NONE',  ( 9.260875088370248420, -3.646744805991136928, -8.814485081663244515 ) ) ;
#40670=DIRECTION ( 'NONE',  ( 0.000000000000000000, 1.000000000000000000, 0.000000000000000000 ) ) ;
#40700=CIRCLE ( 'NONE', #12821, 1.000000000000000000 ) ;
#40702=CARTESIAN_POINT ( 'NONE',  ( 10.88016425062000003, -2.793121555136000023, -6.864957546339999439 ) ) ;
#40708=CARTESIAN_POINT ( 'NONE',  ( 7.392379606866390951, -4.680093573814123609, 6.319105353947795933 ) ) ;
#40718=CARTESIAN_POINT ( 'NONE',  ( 10.99021017617000062, -2.939022385911000068, -5.190637231063000456 ) ) ;
#40719=CARTESIAN_POINT ( 'NONE',  ( 9.886323620223000930, -4.261100936929000049, -5.979198511086000423 ) ) ;
#40720=LINE ( 'NONE', #15183, #47024 ) ;
#40721=CARTESIAN_POINT ( 'NONE',  ( 5.700000000000000178, -1.250000000000000000, 0.000000000000000000 ) ) ;
#40722=CARTESIAN_POINT ( 'NONE',  ( 11.05000833411999928, -5.233205726482999864, 5.017018830968000387 ) ) ;
#40727=AXIS2_PLACEMENT_3D ( 'NONE', #29743, #51046, #3147 ) ;
#40728=EDGE_CURVE ( 'NONE', #34244, #56244, #50181, .T. ) ;
#40747=ORIENTED_EDGE ( 'NONE', *, *, #52390, .T. ) ;
#40748=CARTESIAN_POINT ( 'NONE',  ( 10.59303089732000025, -2.436232726560000117, 7.793465286118999913 ) ) ;
#40752=CARTESIAN_POINT ( 'NONE',  ( 7.700043146791999860, -3.346260729029000291, 6.002247316312999459 ) ) ;
#40765=CARTESIAN_POINT ( 'NONE',  ( 10.57793869653000129, -4.393380534095000733, -6.024358525186999991 ) ) ;
#40775=VERTEX_POINT ( 'NONE', #18370 ) ;
#40783=CARTESIAN_POINT ( 'NONE',  ( 10.48414299032999963, -4.098653366703000067, -9.351353705206001621 ) ) ;
#40798=AXIS2_PLACEMENT_3D ( 'NONE', #61956, #35733, #30488 ) ;
#40801=B_SPLINE_CURVE_WITH_KNOTS ( 'NONE', 3,
 ( #49489, #64518, #65216, #12091 ),
 .UNSPECIFIED., .F., .F.,
 ( 4, 4 ),
 ( 0.000000000000000000, 1.000000000000000000 ),
 .UNSPECIFIED. ) ;
#40805=ORIENTED_EDGE ( 'NONE', *, *, #34272, .F. ) ;
#40806=CARTESIAN_POINT ( 'NONE',  ( 8.604019353210000887, -5.165500668528999917, 8.645534272955000432 ) ) ;
#40815=ORIENTED_EDGE ( 'NONE', *, *, #57128, .F. ) ;
#40822=CARTESIAN_POINT ( 'NONE',  ( 11.10000000009000054, -2.699999999911000259, 6.571291220400000022 ) ) ;
#40824=CARTESIAN_POINT ( 'NONE',  ( 8.246323025216810265, -5.454251951018638245, 8.457608258087930153 ) ) ;
#40829=CARTESIAN_POINT ( 'NONE',  ( 10.77808207294999931, -5.296125810246000043, -4.800100549618000478 ) ) ;
#40836=CARTESIAN_POINT ( 'NONE',  ( 9.661149330668999724, -3.300107492866999781, -5.762405935562999737 ) ) ;
#40837=CARTESIAN_POINT ( 'NONE',  ( 10.32322128467999889, -3.399999874579999748, -4.621083553505000552 ) ) ;
#40838=CARTESIAN_POINT ( 'NONE',  ( 8.174990947233128580, -2.650692654197974729, 7.500004443805800669 ) ) ;
#40847=CARTESIAN_POINT ( 'NONE',  ( 8.187144353207999714, -4.968144979409999884, 5.971795951526999602 ) ) ;
#40853=CARTESIAN_POINT ( 'NONE',  ( 10.44811814679000150, -5.235603901491000300, -6.609968500665999613 ) ) ;
#40865=PRESENTATION_STYLE_ASSIGNMENT (( #25815 ) ) ;
#40866=DIRECTION ( 'NONE',  ( 0.000000000000000000, -0.8648648648648717963, -0.5020047465136829867 ) ) ;
#40870=CARTESIAN_POINT ( 'NONE',  ( 8.893204545428000429, -4.599999999999999645, -6.188268997401999982 ) ) ;
#40874=EDGE_CURVE ( 'NONE', #29433, #27164, #22220, .T. ) ;
#40889=CARTESIAN_POINT ( 'NONE',  ( 8.793536308085935005, -2.899999999999999911, 6.665341197419078156 ) ) ;
#40894=CARTESIAN_POINT ( 'NONE',  ( 10.92932301586054145, -2.313027949505928493, 7.958417374028298852 ) ) ;
#40895=CARTESIAN_POINT ( 'NONE',  ( 7.994581853207999522, -2.263562268490999951, 8.007440964304000985 ) ) ;
#40910=CARTESIAN_POINT ( 'NONE',  ( 8.913566940379999082, -2.550589632307000088, 8.854674225901000284 ) ) ;
#40911=VERTEX_POINT ( 'NONE', #19043 ) ;
#40915=CARTESIAN_POINT ( 'NONE',  ( 7.578319455099681967, -4.092892350974873139, 5.763267803938307843 ) ) ;
#40916=CARTESIAN_POINT ( 'NONE',  ( 7.716851002542999716, -2.832432432432000269, 6.822293592207000934 ) ) ;
#40918=ORIENTED_EDGE ( 'NONE', *, *, #55802, .F. ) ;
#40927=CARTESIAN_POINT ( 'NONE',  ( 8.668612063651316646, -4.202134689411700208, 5.871184905936384979 ) ) ;
#40931=VECTOR ( 'NONE', #47734, 1000.000000000000000 ) ;
#40933=FACE_OUTER_BOUND ( 'NONE', #51318, .T. ) ;
#40943=CARTESIAN_POINT ( 'NONE',  ( 11.01776264201000011, -4.914128622650000722, 8.587713430305999651 ) ) ;
#40951=CIRCLE ( 'NONE', #50981, 10.75000000000000533 ) ;
#40952=CARTESIAN_POINT ( 'NONE',  ( 11.01817738136000102, -5.556757561671000545, -4.991717353675000801 ) ) ;
#40954=CARTESIAN_POINT ( 'NONE',  ( 10.90000000000000036, -2.399999999999999911, -6.571291218949999902 ) ) ;
#40958=CARTESIAN_POINT ( 'NONE',  ( 10.91307648679999964, -2.096298111716999646, 7.827187677719999570 ) ) ;
#40959=EDGE_LOOP ( 'NONE', ( #42913, #9450, #20401, #45209, #44894, #16257, #55310, #52163, #34917, #29191, #51919, #34481, #39634 ) ) ;
#40964=ORIENTED_EDGE ( 'NONE', *, *, #60102, .T. ) ;
#40970=CARTESIAN_POINT ( 'NONE',  ( 10.25313817995475674, -2.714785337465082549, 7.027193780659055200 ) ) ;
#40974=FACE_OUTER_BOUND ( 'NONE', #26458, .T. ) ;
#40983=ORIENTED_EDGE ( 'NONE', *, *, #58167, .F. ) ;
#40999=FACE_OUTER_BOUND ( 'NONE', #14524, .T. ) ;
#41001=B_SPLINE_CURVE_WITH_KNOTS ( 'NONE', 3,
 ( #29551, #2946, #24963, #46981 ),
 .UNSPECIFIED., .F., .F.,
 ( 4, 4 ),
 ( 0.000000000000000000, 0.1254469995254103021 ),
 .UNSPECIFIED. ) ;
#41020=FACE_OUTER_BOUND ( 'NONE', #6196, .T. ) ;
#41045=CARTESIAN_POINT ( 'NONE',  ( 8.070721554491710137, -3.646115526505184778, 8.813957122113405873 ) ) ;
#41046=VECTOR ( 'NONE', #57162, 1000.000000000000000 ) ;
#41059=EDGE_CURVE ( 'NONE', #46265, #29696, #10876, .T. ) ;
#41067=CARTESIAN_POINT ( 'NONE',  ( 10.48237399227000033, -2.917144342353999775, -4.649494773176000351 ) ) ;
#41068=CARTESIAN_POINT ( 'NONE',  ( 9.446306596383999832, -5.231133027468000130, -6.569831606205999819 ) ) ;
#41075=B_SPLINE_CURVE_WITH_KNOTS ( 'NONE', 3,
 ( #29771, #2152, #56322, #61224, #3179, #23812, #18229, #39904, #40243, #50042 ),
 .UNSPECIFIED., .F., .F.,
 ( 4, 2, 2, 2, 4 ),
 ( 0.2180895000437835241, 0.4135671250328376569, 0.6090447500218918453, 0.8045223750109458116, 1.000000000000000000 ),
 .UNSPECIFIED. ) ;
#41077=CARTESIAN_POINT ( 'NONE',  ( 10.90000000000000036, -2.778483479159999714, -6.925197956411000000 ) ) ;
#41097=CARTESIAN_POINT ( 'NONE',  ( 11.12914445903999905, -3.083861519183999977, 8.586004431109000024 ) ) ;
#41100=CARTESIAN_POINT ( 'NONE',  ( 7.591111298125107432, -3.321015683491707282, 8.680015853441066298 ) ) ;
#41101=CARTESIAN_POINT ( 'NONE',  ( 8.111566940377999302, -3.326257819185999942, 8.794522506294001118 ) ) ;
#41112=CARTESIAN_POINT ( 'NONE',  ( 11.25041341105000114, -5.730771985297000271, 8.122672103119001008 ) ) ;
#41115=ORIENTED_EDGE ( 'NONE', *, *, #65162, .T. ) ;
#41119=VERTEX_POINT ( 'NONE', #27308 ) ;
#41129=CARTESIAN_POINT ( 'NONE',  ( 8.493356027204001180, -5.097500218784999149, 6.607661537772998805 ) ) ;
#41134=CARTESIAN_POINT ( 'NONE',  ( 11.03852705926000155, -5.246732451374000128, 5.026582089102999085 ) ) ;
#41138=B_SPLINE_CURVE_WITH_KNOTS ( 'NONE', 3,
 ( #66671, #60743, #65978, #2024, #67013, #65636, #55504, #7606, #23342, #34189, #28955, #50258, #2704, #45020, #29643, #66325, #19122, #13212 ),
 .UNSPECIFIED., .F., .F.,
 ( 4, 2, 2, 2, 2, 2, 2, 2, 4 ),
 ( 0.1070776897655759813, 0.2026877965917215363, 0.2982979034178671052, 0.3939080102440126185, 0.4895181170701581874, 0.5851282238963034787, 0.6807383307224488256, 0.7763484375485940614, 0.8719585443747394082 ),
 .UNSPECIFIED. ) ;
#41139=CARTESIAN_POINT ( 'NONE',  ( 11.15192313136999935, -2.359310578948000003, -6.636692315558000210 ) ) ;
#41150=VECTOR ( 'NONE', #15213, 1000.000000000000000 ) ;
#41162=CARTESIAN_POINT ( 'NONE',  ( 7.999933059623999476, -5.198566224659999513, 8.332559954171999905 ) ) ;
#41166=CIRCLE ( 'NONE', #59026, 10.75000000000000533 ) ;
#41174=DIRECTION ( 'NONE',  ( -2.859035942644044579E-07, 0.9999999999998158140, 5.353374572246079530E-07 ) ) ;
#41177=CARTESIAN_POINT ( 'NONE',  ( 7.834258984672959336, -4.908978639643027719, 6.449989159278149309 ) ) ;
#41178=CARTESIAN_POINT ( 'NONE',  ( 7.100000000000000533, -4.000000000000000000, 7.500000000000000000 ) ) ;
#41179=CARTESIAN_POINT ( 'NONE',  ( 8.269748398527868360, -5.103706565029416886, 8.846130348739302818 ) ) ;
#41181=ORIENTED_EDGE ( 'NONE', *, *, #28726, .T. ) ;
#41182=CARTESIAN_POINT ( 'NONE',  ( 10.48792048572999924, -5.025034920168000241, -4.782290442434000255 ) ) ;
#41186=ORIENTED_EDGE ( 'NONE', *, *, #29375, .F. ) ;
#41189=CARTESIAN_POINT ( 'NONE',  ( 10.06491331857999860, -5.318469253323000245, -7.099528416287999910 ) ) ;
#41199=CARTESIAN_POINT ( 'NONE',  ( 7.390495559621999888, -2.216884807317999861, 8.370075800106999253 ) ) ;
#41204=CARTESIAN_POINT ( 'NONE',  ( 10.25880564679000173, -2.491773655925000330, -7.289938045981000592 ) ) ;
#41212=ORIENTED_EDGE ( 'NONE', *, *, #28727, .T. ) ;
#41246=CARTESIAN_POINT ( 'NONE',  ( 10.37901637862746895, -2.804465802327228197, 8.962024696469146789 ) ) ;
#41249=CARTESIAN_POINT ( 'NONE',  ( 0.000000000000000000, -2.899999999999999911, -7.500000000000000000 ) ) ;
#41254=CARTESIAN_POINT ( 'NONE',  ( 9.341483607044001047, -4.148132978932999926, 9.337467253566000380 ) ) ;
#41255=ORIENTED_EDGE ( 'NONE', *, *, #33187, .T. ) ;
#41258=CARTESIAN_POINT ( 'NONE',  ( 10.49412055961999890, -2.866949708568999888, -8.960719633954001395 ) ) ;
#41260=CARTESIAN_POINT ( 'NONE',  ( 7.585160972467329898, -4.237318164244575414, 5.776645283239123074 ) ) ;
#41269=B_SPLINE_CURVE_WITH_KNOTS ( 'NONE', 3,
 ( #47210, #57007, #35351, #52446, #4540, #14707, #46865, #46523, #19951, #35691, #56674, #8774 ),
 .UNSPECIFIED., .F., .F.,
 ( 4, 2, 2, 2, 2, 4 ),
 ( 0.000000000000000000, 0.2500000000000117129, 0.3750000000000203726, 0.4375000000000172085, 0.5000000000000140998, 1.000000000000000000 ),
 .UNSPECIFIED. ) ;
#41275=EDGE_CURVE ( 'NONE', #6365, #53919, #18493, .T. ) ;
#41285=CARTESIAN_POINT ( 'NONE',  ( 10.89598863732999945, -5.294083316034999598, 4.900488582003999838 ) ) ;
#41290=CARTESIAN_POINT ( 'NONE',  ( 11.24052627608000066, -2.774025043188999895, 6.782107572692000375 ) ) ;
#41293=LINE ( 'NONE', #14724, #53107 ) ;
#41297=CARTESIAN_POINT ( 'NONE',  ( 11.02143415462000142, -6.126230856447000050, -5.117104822491000071 ) ) ;
#41299=DIRECTION ( 'NONE',  ( -1.000000000000000000, 0.000000000000000000, 0.000000000000000000 ) ) ;
#41304=CARTESIAN_POINT ( 'NONE',  ( 9.966331042021000286, -2.304002513595999613, 6.575636708208000059 ) ) ;
#41311=VECTOR ( 'NONE', #10151, 1000.000000000000000 ) ;
#41332=CARTESIAN_POINT ( 'NONE',  ( 9.944325809452999820, -5.443013936195000291, 7.367349259341000156 ) ) ;
#41335=CARTESIAN_POINT ( 'NONE',  ( 5.700000001242999659, -1.249999998757000075, 1.883720477311000285E-09 ) ) ;
#41342=CARTESIAN_POINT ( 'NONE',  ( 10.41258553782401464, -4.805411882504589727, -4.969623107670830819 ) ) ;
#41344=VECTOR ( 'NONE', #26006, 1000.000000000000114 ) ;
#41350=CARTESIAN_POINT ( 'NONE',  ( 11.05049011050999930, -2.763560161389000402, -5.018746270741000437 ) ) ;
#41351=CARTESIAN_POINT ( 'NONE',  ( 9.926183059621999760, -4.356410583133000003, -9.313949118577001585 ) ) ;
#41358=PLANE ( 'NONE',  #63831 ) ;
#41363=CARTESIAN_POINT ( 'NONE',  ( 8.445233760363073827, -5.313925467271338299, 7.853812692271767482 ) ) ;
#41385=CARTESIAN_POINT ( 'NONE',  ( 11.03723142223999965, -8.047823047122999895, -7.049859988296000246 ) ) ;
#41392=B_SPLINE_CURVE_WITH_KNOTS ( 'NONE', 3,
 ( #68353, #51938, #68014, #35870 ),
 .UNSPECIFIED., .F., .F.,
 ( 4, 4 ),
 ( 0.000000000000000000, 1.000000000000000000 ),
 .UNSPECIFIED. ) ;
#41396=CARTESIAN_POINT ( 'NONE',  ( 10.61721988130000049, -5.045606037229999785, -6.386907901056999570 ) ) ;
#41412=CARTESIAN_POINT ( 'NONE',  ( 7.964385314170995933, -2.867871570892000399, 6.759005350280994584 ) ) ;
#41415=DIRECTION ( 'NONE',  ( 0.8480635683784329970, -0.3746919961710145075, -0.3746919961710145075 ) ) ;
#41441=CARTESIAN_POINT ( 'NONE',  ( 10.09181272066999924, -2.440908155048000516, 7.817368209339999652 ) ) ;
#41444=CARTESIAN_POINT ( 'NONE',  ( 9.240543146793999796, -4.158911960977000000, 5.873536005760000123 ) ) ;
#41452=CARTESIAN_POINT ( 'NONE',  ( 10.17500046684972936, -2.650307855384914202, 7.500001770945068813 ) ) ;
#41453=ORIENTED_EDGE ( 'NONE', *, *, #7400, .T. ) ;
#41456=CARTESIAN_POINT ( 'NONE',  ( 11.09999999999999964, -4.000000000000000000, 7.500000000000000000 ) ) ;
#41459=CARTESIAN_POINT ( 'NONE',  ( 9.780291077142999612, -3.021588645102999848, -8.450043670922001482 ) ) ;
#41470=ORIENTED_EDGE ( 'NONE', *, *, #12087, .T. ) ;
#41471=CARTESIAN_POINT ( 'NONE',  ( 8.057193283769001013, -5.122325659685000865, 6.732791538586998747 ) ) ;
#41477=CARTESIAN_POINT ( 'NONE',  ( 10.39355669675000016, -4.089958462238000081, -9.188182957628999503 ) ) ;
#41496=CARTESIAN_POINT ( 'NONE',  ( 9.015543146794000151, -4.175914961544999748, 5.699510287082000026 ) ) ;
#41505=CARTESIAN_POINT ( 'NONE',  ( 11.09999999999999964, -4.000000000000000000, 7.500000000000000000 ) ) ;
#41515=CARTESIAN_POINT ( 'NONE',  ( 8.259902546588161698, -5.265334245408268998, 8.693842063270954768 ) ) ;
#41518=CARTESIAN_POINT ( 'NONE',  ( 10.59787083401000096, -4.986416387023999697, -5.076332610094000941 ) ) ;
#41523=CARTESIAN_POINT ( 'NONE',  ( 9.976909913808000852, -4.233164088428999605, -6.141918726850000176 ) ) ;
#41524=CARTESIAN_POINT ( 'NONE',  ( 10.47094409420000005, -5.100000000000000533, 6.571291218949999902 ) ) ;
#41539=CARTESIAN_POINT ( 'NONE',  ( 10.94033064679000233, -5.142732045902000948, -6.493502833853999512 ) ) ;
#41550=ORIENTED_EDGE ( 'NONE', *, *, #20598, .F. ) ;
#41551=FACE_OUTER_BOUND ( 'NONE', #60213, .T. ) ;
#41553=CARTESIAN_POINT ( 'NONE',  ( 11.09999999999999964, -0.5000000000000000000, -9.662944685757000940 ) ) ;
#41584=ORIENTED_EDGE ( 'NONE', *, *, #23704, .T. ) ;
#41585=VECTOR ( 'NONE', #60664, 1000.000000000000000 ) ;
#41592=VERTEX_POINT ( 'NONE', #16298 ) ;
#41596=CARTESIAN_POINT ( 'NONE',  ( 11.09999999999999964, -2.685305999535000154, 6.664030027596000494 ) ) ;
#41597=CARTESIAN_POINT ( 'NONE',  ( 8.181105646794000208, -5.485781663882000281, 8.532068390166999805 ) ) ;
#41602=CARTESIAN_POINT ( 'NONE',  ( 10.68343305961999867, -3.810133104029999718, -5.661126601970999594 ) ) ;
#41603=CARTESIAN_POINT ( 'NONE',  ( 7.575399445029316503, -4.029967771855843317, 5.761070296328433038 ) ) ;
#41605=CARTESIAN_POINT ( 'NONE',  ( 7.930984152288867328, -5.149131075244117284, 6.790530796032830274 ) ) ;
#41620=ORIENTED_EDGE ( 'NONE', *, *, #13887, .F. ) ;
#41623=ORIENTED_EDGE ( 'NONE', *, *, #15075, .F. ) ;
#41630=CARTESIAN_POINT ( 'NONE',  ( 10.83659005484000026, -5.133183563847000030, 8.848364935581999546 ) ) ;
#41632=CARTESIAN_POINT ( 'NONE',  ( 10.90000000000000036, -0.2999999999999999889, 4.902439024389999567 ) ) ;
#41634=CARTESIAN_POINT ( 'NONE',  ( 10.90000000346999975, -5.100000000044000892, -5.157071296039999808 ) ) ;
#41635=ORIENTED_EDGE ( 'NONE', *, *, #16275, .T. ) ;
#41643=CARTESIAN_POINT ( 'NONE',  ( 9.854949224988001077, -2.800315695760000168, 9.013807298610000629 ) ) ;
#41646=ORIENTED_EDGE ( 'NONE', *, *, #27187, .T. ) ;
#41649=CARTESIAN_POINT ( 'NONE',  ( 11.18051369187999988, -5.340070732632000272, 8.416150632189001612 ) ) ;
#41655=EDGE_CURVE ( 'NONE', #68830, #49271, #43919, .T. ) ;
#41659=CARTESIAN_POINT ( 'NONE',  ( 9.191972128127998687, -4.867164667115999599, -6.095483598963999938 ) ) ;
#41671=CARTESIAN_POINT ( 'NONE',  ( 9.261668853699999815, -2.944250413017999612, 6.507387951280999339 ) ) ;
#41682=CARTESIAN_POINT ( 'NONE',  ( 10.90454231406000041, -5.099691312770999296, -5.130383474399000221 ) ) ;
#41685=CARTESIAN_POINT ( 'NONE',  ( 10.95904654087999930, -2.844192924580000170, 5.123817848908000627 ) ) ;
#41689=CARTESIAN_POINT ( 'NONE',  ( 11.19050685320999960, -2.516759970060999940, -6.840363309917000478 ) ) ;
#41690=CARTESIAN_POINT ( 'NONE',  ( 9.028474612548734513, -4.352782978231400257, 8.850949115404409540 ) ) ;
#41695=ORIENTED_EDGE ( 'NONE', *, *, #1566, .T. ) ;
#41713=CARTESIAN_POINT ( 'NONE',  ( 11.09999999999999964, -7.940796613052000019, 6.945951997396999644 ) ) ;
#41719=VERTEX_POINT ( 'NONE', #48467 ) ;
#41724=CARTESIAN_POINT ( 'NONE',  ( 10.40583502355000078, -8.253917379314000158, -6.947659401770000187 ) ) ;
#41733=CARTESIAN_POINT ( 'NONE',  ( 10.25166529434999951, -3.418639857622999934, -8.733652610425998830 ) ) ;
#41735=ADVANCED_FACE ( 'NONE', ( #22233 ), #53903, .T. ) ;
#41741=ADVANCED_FACE ( 'NONE', ( #63841 ), #15955, .T. ) ;
#41753=CARTESIAN_POINT ( 'NONE',  ( 7.782404085375001834, -2.843788791114000958, 6.809963588862000705 ) ) ;
#41756=CARTESIAN_POINT ( 'NONE',  ( 10.65050275296000137, -5.200029647236999786, 5.937716681140000397 ) ) ;
#41780=CARTESIAN_POINT ( 'NONE',  ( 10.66951732929000052, -4.592671928130000580, 5.841406818427000047 ) ) ;
#41781=EDGE_LOOP ( 'NONE', ( #25982, #64120, #47473, #15910 ) ) ;
#41782=CARTESIAN_POINT ( 'NONE',  ( 8.501777870119797242, -3.152918059059234945, 6.042693032664300468 ) ) ;
#41783=CARTESIAN_POINT ( 'NONE',  ( 9.475897313459000770, -4.122021308488999836, 9.013573548576999883 ) ) ;
#41786=EDGE_LOOP ( 'NONE', ( #23476, #44720, #53736, #42066 ) ) ;
#41794=CARTESIAN_POINT ( 'NONE',  ( 10.93227479887999998, -2.539880901735999785, 6.453614191797999666 ) ) ;
#41797=ORIENTED_EDGE ( 'NONE', *, *, #18365, .F. ) ;
#41800=DIRECTION ( 'NONE',  ( -0.9999999999988525845, -7.523236327271644932E-07, 1.314847452163938853E-06 ) ) ;
#41809=CARTESIAN_POINT ( 'NONE',  ( 10.34947173981000113, -4.457565973839000328, 6.154866550070000386 ) ) ;
#41811=CARTESIAN_POINT ( 'NONE',  ( 7.913666363270997373, -4.616745235331003450, 6.306613118563004328 ) ) ;
#41826=CARTESIAN_POINT ( 'NONE',  ( 7.384456853207000293, -3.346260729029000291, 6.002247316312999459 ) ) ;
#41838=CARTESIAN_POINT ( 'NONE',  ( 7.486433059621999675, -5.321924421352999701, 8.118250081378000971 ) ) ;
#41858=CARTESIAN_POINT ( 'NONE',  ( 8.177847774682394544, -5.688938049909738837, 7.046656128444472422 ) ) ;
#41868=CARTESIAN_POINT ( 'NONE',  ( 9.800903104272999045, -2.772050158355999994, -8.125211791007998841 ) ) ;
#41873=CARTESIAN_POINT ( 'NONE',  ( 8.700696199801130959, -5.750348757284029944, 7.524179667756733636 ) ) ;
#41880=ORIENTED_EDGE ( 'NONE', *, *, #56145, .F. ) ;
#41883=COLOUR_RGB ( '', 0.08235294, 0.09019608, 0.10196078) ;
#41892=VERTEX_POINT ( 'NONE', #49847 ) ;
#41897=DIRECTION ( 'NONE',  ( 0.000000000000000000, -1.000000000000000000, 0.000000000000000000 ) ) ;
#41903=CARTESIAN_POINT ( 'NONE',  ( 8.615014049714954325, -5.084477605260944166, -6.679144390359880390 ) ) ;
#41905=ORIENTED_EDGE ( 'NONE', *, *, #9016, .T. ) ;
#41918=CARTESIAN_POINT ( 'NONE',  ( 9.108369332021359455, -3.858817869685470470, 8.849160905739024585 ) ) ;
#41940=DIRECTION ( 'NONE',  ( -1.000000000000000000, 0.000000000000000000, 0.000000000000000000 ) ) ;
#41941=CARTESIAN_POINT ( 'NONE',  ( 8.347269353210000631, -2.741638482234999952, 6.457327039244000311 ) ) ;
#41945=CARTESIAN_POINT ( 'NONE',  ( 10.07763305961999833, -2.169024213715999849, -7.244986319234999250 ) ) ;
#41946=CARTESIAN_POINT ( 'NONE',  ( 7.484057796017113517, -2.418173406717145646, 6.775917929113594695 ) ) ;
#41967=LINE ( 'NONE', #53144, #41311 ) ;
#41976=CARTESIAN_POINT ( 'NONE',  ( 9.388626433405999450, -4.079401915682999480, 9.259353168384000909 ) ) ;
#41990=CARTESIAN_POINT ( 'NONE',  ( 10.90000000000000036, -0.2999999999999999889, -4.902439024389999567 ) ) ;
#41998=CARTESIAN_POINT ( 'NONE',  ( 11.09999999999999964, -2.861044734458999627E-13, 5.200284647344000995E-13 ) ) ;
#41999=CARTESIAN_POINT ( 'NONE',  ( 10.59344961228999971, -5.297755890367000120, 8.474197994416998725 ) ) ;
#42010=CARTESIAN_POINT ( 'NONE',  ( 10.67905590578999941, -2.899999999999999911, 6.571291218949999902 ) ) ;
#42022=CARTESIAN_POINT ( 'NONE',  ( 10.93728138146000006, -5.425439422033999648, 7.240583766112999697 ) ) ;
#42028=ORIENTED_EDGE ( 'NONE', *, *, #100, .F. ) ;
#42034=CARTESIAN_POINT ( 'NONE',  ( 10.52052890781999928, -2.899999999999999911, 6.152188490330000370 ) ) ;
#42039=CYLINDRICAL_SURFACE ( 'NONE', #4255, 1.350000000000000089 ) ;
#42040=CARTESIAN_POINT ( 'NONE',  ( 7.910784822166045949, -5.348998117051901424, 7.262899563230540423 ) ) ;
#42061=VERTEX_POINT ( 'NONE', #24141 ) ;
#42066=ORIENTED_EDGE ( 'NONE', *, *, #68641, .F. ) ;
#42074=CARTESIAN_POINT ( 'NONE',  ( 9.797024780922274800, -5.515983957001070692, -6.595663371089560911 ) ) ;
#42083=CARTESIAN_POINT ( 'NONE',  ( 9.780291077142999612, -3.021588645102999848, -8.450043670922001482 ) ) ;
#42088=AXIS2_PLACEMENT_3D ( 'NONE', #69021, #52949, #6075 ) ;
#42096=CARTESIAN_POINT ( 'NONE',  ( 8.437014469680988782, -2.901284097310000920, 6.624005965434003329 ) ) ;
#42097=VERTEX_POINT ( 'NONE', #61801 ) ;
#42100=EDGE_CURVE ( 'NONE', #53475, #2231, #52518, .T. ) ;
#42101=CARTESIAN_POINT ( 'NONE',  ( 10.35162153983000088, -3.367195699800999975, -4.861353673146999732 ) ) ;
#42102=CARTESIAN_POINT ( 'NONE',  ( 9.507558421712998253, -4.699533657262000119, -6.366989705700999203 ) ) ;
#42105=CARTESIAN_POINT ( 'NONE',  ( 10.80815535238000002, -2.937528991339000140, 8.948455587554001056 ) ) ;
#42107=CARTESIAN_POINT ( 'NONE',  ( 9.819055905797000605, -2.899999999999999911, -6.571291218949999902 ) ) ;
#42119=CARTESIAN_POINT ( 'NONE',  ( 10.88876599830666692, -5.215403687430652191, 6.904706716043305548 ) ) ;
#42121=ORIENTED_EDGE ( 'NONE', *, *, #28810, .T. ) ;
#42123=PRODUCT_CONTEXT ( 'NONE', #6535, 'mechanical' ) ;
#42133=CARTESIAN_POINT ( 'NONE',  ( 10.61382642076999971, -3.385081736013999976, 5.849525238167000651 ) ) ;
#42135=CARTESIAN_POINT ( 'NONE',  ( 8.439067896944781211, -2.959717315122096348, 6.275320676522057717 ) ) ;
#42136=CARTESIAN_POINT ( 'NONE',  ( 7.609456853206999938, -3.276313010012999793, 5.841993238691999935 ) ) ;
#42139=ORIENTED_EDGE ( 'NONE', *, *, #15959, .F. ) ;
#42148=CARTESIAN_POINT ( 'NONE',  ( 9.256662271119999730, -4.025830307267999508, 9.295859242339000517 ) ) ;
#42158=DIRECTION ( 'NONE',  ( 0.8660254037843856390, 0.000000000000000000, -0.5000000000000918154 ) ) ;
#42168=EDGE_CURVE ( 'NONE', #664, #46365, #10050, .T. ) ;
#42181=CARTESIAN_POINT ( 'NONE',  ( 7.256081853207000165, -2.531197775378000170, 8.216705951490000714 ) ) ;
#42186=FACE_OUTER_BOUND ( 'NONE', #953, .T. ) ;
#42196=CARTESIAN_POINT ( 'NONE',  ( 7.518870559622000016, -3.206365290996999740, 5.681739161071000410 ) ) ;
#42215=CARTESIAN_POINT ( 'NONE',  ( 8.220624047935833900, -5.675834487486897117, 7.965153098552243627 ) ) ;
#42224=CARTESIAN_POINT ( 'NONE',  ( 10.19691842572999896, -4.268950419651999617, -8.781589108989999559 ) ) ;
#42226=B_SPLINE_CURVE_WITH_KNOTS ( 'NONE', 3,
 ( #19035, #13801, #40364, #61685 ),
 .UNSPECIFIED., .F., .F.,
 ( 4, 4 ),
 ( 0.000000000000000000, 1.000000000000000000 ),
 .UNSPECIFIED. ) ;
#42229=CARTESIAN_POINT ( 'NONE',  ( 8.734407071272288547, -5.610846102776929634, 8.247418371894697842 ) ) ;
#42238=CARTESIAN_POINT ( 'NONE',  ( 9.251933059621999078, -5.159251056493999954, 9.109488373271000583 ) ) ;
#42263=CARTESIAN_POINT ( 'NONE',  ( 10.12544718489496098, -5.350147103445326735, -7.676667778836361755 ) ) ;
#42275=CARTESIAN_POINT ( 'NONE',  ( 9.218006583692512024, -2.655300810998681982, 7.619131915109693232 ) ) ;
#42276=ADVANCED_FACE ( 'NONE', ( #25427 ), #14261, .T. ) ;
#42292=CARTESIAN_POINT ( 'NONE',  ( 11.09999999999999964, -4.000000000000000000, 7.500000000000000000 ) ) ;
#42299=CARTESIAN_POINT ( 'NONE',  ( 10.97843137008999825, -5.235400103863000254, 6.782920672145000829 ) ) ;
#42300=CARTESIAN_POINT ( 'NONE',  ( 7.058516392956000196, -4.314043295739000250, 8.819145559946001356 ) ) ;
#42304=CARTESIAN_POINT ( 'NONE',  ( 10.15335805961999860, -3.144986649008000068, -5.860958514434000399 ) ) ;
#42305=CARTESIAN_POINT ( 'NONE',  ( 7.466089535749324213, -2.297169363456695201, 7.143273799371222310 ) ) ;
#42308=ORIENTED_EDGE ( 'NONE', *, *, #50321, .F. ) ;
#42313=ORIENTED_EDGE ( 'NONE', *, *, #41059, .F. ) ;
#42326=ORIENTED_EDGE ( 'NONE', *, *, #29687, .F. ) ;
#42331=CARTESIAN_POINT ( 'NONE',  ( 10.16829915263999951, -4.567213659083999566, 5.832528837986999726 ) ) ;
#42344=CARTESIAN_POINT ( 'NONE',  ( 7.717918984469999799, -2.852331559125000027, 6.784354950350999225 ) ) ;
#42367=ORIENTED_EDGE ( 'NONE', *, *, #41275, .T. ) ;
#42369=CARTESIAN_POINT ( 'NONE',  ( 9.457462135716001583, -5.100000000000000533, -6.571291218949999902 ) ) ;
#42370=CARTESIAN_POINT ( 'NONE',  ( 9.696086916451999826, -2.554404004330999900, 7.600685922079000179 ) ) ;
#42385=CARTESIAN_POINT ( 'NONE',  ( 10.75915805961999894, -5.387268372866000021, -6.278119777966000292 ) ) ;
#42391=EDGE_CURVE ( 'NONE', #52849, #46074, #5816, .T. ) ;
#42399=VERTEX_POINT ( 'NONE', #58965 ) ;
#42409=ORIENTED_EDGE ( 'NONE', *, *, #25570, .F. ) ;
#42426=CARTESIAN_POINT ( 'NONE',  ( 10.46009514222999925, -2.565650894080999667, -6.975682682930000489 ) ) ;
#42428=ORIENTED_EDGE ( 'NONE', *, *, #47046, .T. ) ;
#42431=CARTESIAN_POINT ( 'NONE',  ( 8.279780176894341537, -3.802829724692906588, 6.095677100425044515 ) ) ;
#42436=CARTESIAN_POINT ( 'NONE',  ( 10.27121258196999953, -3.420947237194000401, 4.846519661431999637 ) ) ;
#42440=CARTESIAN_POINT ( 'NONE',  ( 8.325003570449004187, -2.868532950405002779, 6.316175323229005656 ) ) ;
#42445=CARTESIAN_POINT ( 'NONE',  ( 9.533427734455999669, -2.564762519363000148, 6.150594768287000136 ) ) ;
#42449=B_SPLINE_CURVE_WITH_KNOTS ( 'NONE', 3,
 ( #9388, #639, #32799, #22297 ),
 .UNSPECIFIED., .F., .F.,
 ( 4, 4 ),
 ( 0.000000000000000000, 1.000000000000000000 ),
 .UNSPECIFIED. ) ;
#42463=ORIENTED_EDGE ( 'NONE', *, *, #14550, .F. ) ;
#42473=EDGE_CURVE ( 'NONE', #9350, #11696, #44313, .T. ) ;
#42474=CARTESIAN_POINT ( 'NONE',  ( 9.409421956854998825, -2.113407700033000047, 7.914197133433000353 ) ) ;
#42478=CARTESIAN_POINT ( 'NONE',  ( 7.583058059622000080, -4.763531818439999732, 5.668890958491999754 ) ) ;
#42486=CARTESIAN_POINT ( 'NONE',  ( 10.87021507563000000, -2.226042145532000305, 7.782753277595999997 ) ) ;
#42492=ORIENTED_EDGE ( 'NONE', *, *, #62120, .T. ) ;
#42500=DIRECTION ( 'NONE',  ( -1.000000000000000000, 0.000000000000000000, 0.000000000000000000 ) ) ;
#42507=AXIS2_PLACEMENT_3D ( 'NONE', #45470, #34987, #39532 ) ;
#42518=CARTESIAN_POINT ( 'NONE',  ( 8.592629440379999650, -3.856773448568000084, 5.521258396339000285 ) ) ;
#42522=DIRECTION ( 'NONE',  ( -1.000000000000000000, 1.157371756800000045E-14, 1.736057635198999949E-14 ) ) ;
#42529=VERTEX_POINT ( 'NONE', #53379 ) ;
#42530=CARTESIAN_POINT ( 'NONE',  ( 8.341918146793998901, -5.601799093797000140, 7.176147756900999930 ) ) ;
#42532=EDGE_CURVE ( 'NONE', #2041, #52805, #40951, .T. ) ;
#42536=EDGE_LOOP ( 'NONE', ( #21559, #27922, #41880, #36253 ) ) ;
#42542=CARTESIAN_POINT ( 'NONE',  ( 9.136057238048000073, -5.084840204920000772, -6.477689566282000655 ) ) ;
#42550=CARTESIAN_POINT ( 'NONE',  ( 8.403769448316676716, -2.537713777690222994, 8.442983533627888448 ) ) ;
#42561=CARTESIAN_POINT ( 'NONE',  ( 11.09999999999999964, -4.000000000000000000, 7.500000000000000000 ) ) ;
#42574=EDGE_CURVE ( 'NONE', #49213, #1541, #11649, .T. ) ;
#42584=CARTESIAN_POINT ( 'NONE',  ( 11.07071167063000061, -6.643645819897000315, -5.582924995379999977 ) ) ;
#42605=VECTOR ( 'NONE', #41800, 1000.000000000000114 ) ;
#42613=EDGE_CURVE ( 'NONE', #13775, #33561, #24, .T. ) ;
#42629=CARTESIAN_POINT ( 'NONE',  ( 11.01776264201000011, -4.914128622650000722, 8.587713430305999651 ) ) ;
#42630=CARTESIAN_POINT ( 'NONE',  ( 8.064120559623999540, -4.228293421747000735, 8.941387937291999322 ) ) ;
#42632=CARTESIAN_POINT ( 'NONE',  ( 9.678448551390218313, -4.965577467693124802, -8.481121822464514182 ) ) ;
#42633=EDGE_CURVE ( 'NONE', #10274, #29557, #13414, .T. ) ;
#42635=CARTESIAN_POINT ( 'NONE',  ( 11.09178064679000109, -4.578543110806999827, -8.908602356389000221 ) ) ;
#42636=CARTESIAN_POINT ( 'NONE',  ( 7.744874159809953085, -5.467231327630983628, 8.434612347329016657 ) ) ;
#42653=CARTESIAN_POINT ( 'NONE',  ( 10.67905590578999941, -2.899999999999999911, 6.571291218949999902 ) ) ;
#42658=LINE ( 'NONE', #37411, #21957 ) ;
#42661=CARTESIAN_POINT ( 'NONE',  ( 10.44675369521999997, -2.885048926231000177, 8.863479194807000638 ) ) ;
#42667=ORIENTED_EDGE ( 'NONE', *, *, #56185, .F. ) ;
#42688=ADVANCED_BREP_SHAPE_REPRESENTATION ( '', ( #29488, #9676 ), #16178 ) ;
#42716=DIRECTION ( 'NONE',  ( 0.000000000000000000, 0.8648648648648720183, 0.5020047465136825426 ) ) ;
#42722=LINE ( 'NONE', #21726, #24545 ) ;
#42723=CARTESIAN_POINT ( 'NONE',  ( 10.86460564679000029, -3.843601288168000174, -5.985268170611000471 ) ) ;
#42726=DIRECTION ( 'NONE',  ( 1.000000000000000000, 0.000000000000000000, 0.000000000000000000 ) ) ;
#42743=CARTESIAN_POINT ( 'NONE',  ( 6.999999999999999112, -6.725428974790256476, -3.045254342161083816 ) ) ;
#42747=ORIENTED_EDGE ( 'NONE', *, *, #55505, .T. ) ;
#42766=CARTESIAN_POINT ( 'NONE',  ( 10.77434462036999818, -4.612888200890999713, -8.898797372219998891 ) ) ;
#42770=CARTESIAN_POINT ( 'NONE',  ( 10.91441078833591405, -5.114410788335912450, -6.482042798774522829 ) ) ;
#42772=CARTESIAN_POINT ( 'NONE',  ( 9.266851002542999538, -2.832432432432000269, 6.822293592207000934 ) ) ;
#42773=CARTESIAN_POINT ( 'NONE',  ( 7.000000000000000000, -0.2897247358851999799, 3.000000000000000000 ) ) ;
#42774=EDGE_CURVE ( 'NONE', #23094, #58951, #62544, .T. ) ;
#42780=CARTESIAN_POINT ( 'NONE',  ( 8.332046967449000974, -2.867486995832002616, 6.314275746166007508 ) ) ;
#42784=CARTESIAN_POINT ( 'NONE',  ( 9.409308287954999628, -2.634700736117999931, 8.920302460802998823 ) ) ;
#42787=CARTESIAN_POINT ( 'NONE',  ( 10.27814441345999974, -5.521593622715999850, 8.751220666652999469 ) ) ;
#42788=CARTESIAN_POINT ( 'NONE',  ( 9.883148997457000817, -5.167567567567999731, 6.822293592207000934 ) ) ;
#42791=EDGE_CURVE ( 'NONE', #48042, #10703, #30860, .T. ) ;
#42796=EDGE_CURVE ( 'NONE', #12955, #1683, #32597, .T. ) ;
#42799=LINE ( 'NONE', #47705, #31734 ) ;
#42804=CARTESIAN_POINT ( 'NONE',  ( 10.89438299915333275, -5.254480013706496422, 6.992200716271752547 ) ) ;
#42814=CARTESIAN_POINT ( 'NONE',  ( 9.298040139821001304, -4.087076480742000584, 9.429402848390999736 ) ) ;
#42817=CARTESIAN_POINT ( 'NONE',  ( 10.99874143819000061, -2.710832050839000029, 4.962905352413001125 ) ) ;
#42818=CARTESIAN_POINT ( 'NONE',  ( 7.802019353206999241, -5.638700495537999124, 8.266402903491000487 ) ) ;
#42822=B_SPLINE_CURVE_WITH_KNOTS ( 'NONE', 3,
 ( #20040, #57432, #30882, #26322, #65074, #17194, #64732, #43437, #10920, #59156 ),
 .UNSPECIFIED., .F., .F.,
 ( 4, 2, 2, 2, 4 ),
 ( 0.1253969396550571880, 0.3126920919075452110, 0.4999872441600332618, 0.6872823964125207574, 0.8745775486650082531 ),
 .UNSPECIFIED. ) ;
#42824=CARTESIAN_POINT ( 'NONE',  ( 11.09999999999999964, -6.593648102827000201, 5.598803487171999826 ) ) ;
#42826=ORIENTED_EDGE ( 'NONE', *, *, #59507, .T. ) ;
#42827=CARTESIAN_POINT ( 'NONE',  ( 10.55991645936999923, -5.094263939633999705, 6.075409946530999861 ) ) ;
#42830=ORIENTED_EDGE ( 'NONE', *, *, #16560, .F. ) ;
#42832=CARTESIAN_POINT ( 'NONE',  ( 10.99305444037999990, -4.495427106425000652, -6.233607450113000326 ) ) ;
#42842=VERTEX_POINT ( 'NONE', #54316 ) ;
#42854=CARTESIAN_POINT ( 'NONE',  ( 9.392078467011812037, -5.386183347138083555, -8.566888829028510344 ) ) ;
#42861=CARTESIAN_POINT ( 'NONE',  ( 8.309480646794000336, -2.905864338704999827, 8.940687151810998046 ) ) ;
#42870=B_SPLINE_SURFACE_WITH_KNOTS ( 'NONE', 3, 3, ( 
 ( #62324, #30857, #51825, #3923 ),
 ( #20021, #68239, #9515, #62658 ),
 ( #25609, #24579, #41685, #8155 ),
 ( #18986, #29501, #2900, #24230 ),
 ( #66874, #40312, #61633, #13749 ) ),
 .UNSPECIFIED., .F., .F., .F.,
 ( 4, 1, 4 ),
 ( 4, 4 ),
 ( -0.007897885364823000257, 0.000000000000000000, 0.04616514892271000176 ),
 ( -0.1721959722423999917, 1.172195972106000017 ),
 .UNSPECIFIED. ) ;
#42874=CARTESIAN_POINT ( 'NONE',  ( 8.598668146794999245, -2.376522687267000222, 7.686981355459999499 ) ) ;
#42886=CARTESIAN_POINT ( 'NONE',  ( 9.629471092178999214, -5.100000000000000533, 6.152188490330000370 ) ) ;
#42893=CARTESIAN_POINT ( 'NONE',  ( 8.549219542760198465, -3.460297557318590567, 5.846195167334228948 ) ) ;
#42904=ORIENTED_EDGE ( 'NONE', *, *, #46488, .T. ) ;
#42905=CARTESIAN_POINT ( 'NONE',  ( 10.79353630809283437, -2.899999999999999911, 6.665341197380430849 ) ) ;
#42906=( NAMED_UNIT ( * ) SI_UNIT ( $, .STERADIAN. ) SOLID_ANGLE_UNIT ( ) );
#42911=ORIENTED_EDGE ( 'NONE', *, *, #29067, .F. ) ;
#42913=ORIENTED_EDGE ( 'NONE', *, *, #28951, .F. ) ;
#42917=ORIENTED_EDGE ( 'NONE', *, *, #24656, .F. ) ;
#42919=LINE ( 'NONE', #65268, #45529 ) ;
#42924=ADVANCED_FACE ( 'NONE', ( #48546 ), #20836, .T. ) ;
#42928=ORIENTED_EDGE ( 'NONE', *, *, #42473, .T. ) ;
#42971=CARTESIAN_POINT ( 'NONE',  ( 10.40516264833000015, -5.216401621862000404, 6.765753642936999768 ) ) ;
#42972=CARTESIAN_POINT ( 'NONE',  ( 8.539831853209999935, -5.633481712366999794, 7.451234046297000368 ) ) ;
#42976=CARTESIAN_POINT ( 'NONE',  ( 10.67529314679000052, -3.066674550532999977, -8.703235919197002346 ) ) ;
#42977=CARTESIAN_POINT ( 'NONE',  ( 7.798838663971441321, -4.555560098518249390, 9.151540452632529465 ) ) ;
#42978=CARTESIAN_POINT ( 'NONE',  ( 10.71256247620999957, -5.951803124515000043, 7.233045248871000865 ) ) ;
#42992=CARTESIAN_POINT ( 'NONE',  ( 8.175754440378000254, -2.599231861044000169, 7.909347897884000389 ) ) ;
#42993=DIRECTION ( 'NONE',  ( 0.000000000000000000, 0.000000000000000000, -1.000000000000000000 ) ) ;
#43001=EDGE_CURVE ( 'NONE', #16743, #66793, #27565, .T. ) ;
#43002=CARTESIAN_POINT ( 'NONE',  ( 9.353731048338000065, -2.823575173856999410, 9.032043499493001448 ) ) ;
#43005=DIRECTION ( 'NONE',  ( 0.6684585169941805738, -0.6684585169941805738, 0.3260773253629903334 ) ) ;
#43025=EDGE_CURVE ( 'NONE', #52126, #64582, #46594, .T. ) ;
#43041=CARTESIAN_POINT ( 'NONE',  ( 9.934999999999998721, -4.640430492595999823, -9.117542781427999898 ) ) ;
#43049=ADVANCED_FACE ( 'NONE', ( #998 ), #52904, .T. ) ;
#43056=FACE_OUTER_BOUND ( 'NONE', #3369, .T. ) ;
#43062=CARTESIAN_POINT ( 'NONE',  ( 10.08211398012999993, -4.728049789772000189, -8.793977405422999993 ) ) ;
#43070=ORIENTED_EDGE ( 'NONE', *, *, #7179, .F. ) ;
#43084=CARTESIAN_POINT ( 'NONE',  ( 9.675541251098000117, -4.656741678598999457, -8.653222148251000334 ) ) ;
#43087=EDGE_CURVE ( 'NONE', #17344, #26163, #39157, .T. ) ;
#43091=AXIS2_PLACEMENT_3D ( 'NONE', #64344, #23090, #37449 ) ;
#43098=CARTESIAN_POINT ( 'NONE',  ( 10.55661746422400959, -2.989346313686768397, 5.028522878686708886 ) ) ;
#43100=CARTESIAN_POINT ( 'NONE',  ( 11.18483536755999808, -2.599651619047000040, 7.740676724427999922 ) ) ;
#43111=CARTESIAN_POINT ( 'NONE',  ( 10.20917469696999902, -3.334764780022000163, -5.769478358936999562 ) ) ;
#43113=VERTEX_POINT ( 'NONE', #24306 ) ;
#43123=CARTESIAN_POINT ( 'NONE',  ( 8.212419626809003503, -3.104180672527999896, 6.104185052591001082 ) ) ;
#43126=VECTOR ( 'NONE', #59141, 1000.000000000000227 ) ;
#43127=CARTESIAN_POINT ( 'NONE',  ( 10.83668192271000130, -4.288535286065000562, 9.448729895547000268 ) ) ;
#43130=CARTESIAN_POINT ( 'NONE',  ( 10.58844302970999962, -3.754658547780000521, 5.545362468768000319 ) ) ;
#43145=FACE_OUTER_BOUND ( 'NONE', #54183, .T. ) ;
#43148=CARTESIAN_POINT ( 'NONE',  ( 7.486137746321728237, -5.349333099367949096, 7.677008113425388025 ) ) ;
#43155=CARTESIAN_POINT ( 'NONE',  ( 10.55813551225999980, -2.466564559586000183, 6.633531786299999844 ) ) ;
#43162=DIRECTION ( 'NONE',  ( -1.000000000000000000, 3.552713679099000216E-14, -7.105427358198000432E-14 ) ) ;
#43167=CARTESIAN_POINT ( 'NONE',  ( 10.03491210303999992, -5.615910465798999773, 7.351455544018000943 ) ) ;
#43206=CARTESIAN_POINT ( 'NONE',  ( 9.170316940378999249, -5.558929022707999046, 6.272984818914999927 ) ) ;
#43215=ORIENTED_EDGE ( 'NONE', *, *, #21237, .T. ) ;
#43216=CARTESIAN_POINT ( 'NONE',  ( 9.021581853209999835, -2.193670085072000120, 7.400591740205000768 ) ) ;
#43217=CARTESIAN_POINT ( 'NONE',  ( 9.179055905797000037, -2.899999999999999911, 6.571291218949999902 ) ) ;
#43219=DIRECTION ( 'NONE',  ( 1.000000000000000000, 0.000000000000000000, 0.000000000000000000 ) ) ;
#43226=VERTEX_POINT ( 'NONE', #37536 ) ;
#43234=ORIENTED_EDGE ( 'NONE', *, *, #4718, .F. ) ;
#43237=CARTESIAN_POINT ( 'NONE',  ( 8.449083656217606375, -2.260425563746147670, 7.515772993398566193 ) ) ;
#43243=ORIENTED_EDGE ( 'NONE', *, *, #46571, .F. ) ;
#43248=CARTESIAN_POINT ( 'NONE',  ( 10.62788468813516474, -2.420134780600908364, -6.689474005288416514 ) ) ;
#43258=ORIENTED_EDGE ( 'NONE', *, *, #13887, .T. ) ;
#43260=EDGE_CURVE ( 'NONE', #32830, #37266, #45845, .T. ) ;
#43274=ORIENTED_EDGE ( 'NONE', *, *, #27557, .T. ) ;
#43276=DIRECTION ( 'NONE',  ( -1.000000000000000000, 0.000000000000000000, 0.000000000000000000 ) ) ;
#43279=EDGE_CURVE ( 'NONE', #51438, #51664, #47526, .T. ) ;
#43284=CARTESIAN_POINT ( 'NONE',  ( 11.02452225494999993, -2.775477745048999800, -6.571291218949999902 ) ) ;
#43321=CARTESIAN_POINT ( 'NONE',  ( 9.569799020577001158, -4.064052785562999759, 8.919253808370999792 ) ) ;
#43322=CARTESIAN_POINT ( 'NONE',  ( 8.090519353209000286, -5.342173944271999986, 8.432314172168000610 ) ) ;
#43325=VECTOR ( 'NONE', #36644, 1000.000000000000000 ) ;
#43327=CARTESIAN_POINT ( 'NONE',  ( 10.47111935320999976, -5.170637620872999385, -8.712950754783999940 ) ) ;
#43329=CARTESIAN_POINT ( 'NONE',  ( 7.806648733296884579, -4.393915723649380212, 9.194460218222584302 ) ) ;
#43331=FACE_OUTER_BOUND ( 'NONE', #16103, .T. ) ;
#43348=CARTESIAN_POINT ( 'NONE',  ( 10.40685100253999984, -2.832432432432000269, -6.822293592207000934 ) ) ;
#43349=EDGE_CURVE ( 'NONE', #51331, #11010, #38227, .T. ) ;
#43351=CARTESIAN_POINT ( 'NONE',  ( 9.010191940380000375, -5.040796345420999636, 8.522966281393001609 ) ) ;
#43366=VERTEX_POINT ( 'NONE', #30091 ) ;
#43368=CARTESIAN_POINT ( 'NONE',  ( 8.767881343006999728, -4.605543323398999966, -6.293427432547999523 ) ) ;
#43381=CARTESIAN_POINT ( 'NONE',  ( 9.199609130449999839, -2.551382302226000487, 7.536606162076999738 ) ) ;
#43400=CARTESIAN_POINT ( 'NONE',  ( 9.660601868375998436, -2.901236202253999696, -6.151180522693000086 ) ) ;
#43421=CARTESIAN_POINT ( 'NONE',  ( 11.00119435320999983, -4.640445114785999969, -9.059317673956000405 ) ) ;
#43426=PLANE ( 'NONE',  #21977 ) ;
#43430=ORIENTED_EDGE ( 'NONE', *, *, #68658, .F. ) ;
#43437=CARTESIAN_POINT ( 'NONE',  ( 8.684028039623166606, -2.794631556210835033, 8.206409581471101333 ) ) ;
#43440=CARTESIAN_POINT ( 'NONE',  ( 7.000000000000000000, -6.255435840762999966, -3.000000000000000000 ) ) ;
#43441=CARTESIAN_POINT ( 'NONE',  ( 10.34225158793000077, -3.348983461003999906, -8.881464249475000017 ) ) ;
#43456=FACE_OUTER_BOUND ( 'NONE', #5774, .T. ) ;
#43467=CARTESIAN_POINT ( 'NONE',  ( 11.17811058788999823, -2.762459764047000110, -6.187206491620000470 ) ) ;
#43469=CARTESIAN_POINT ( 'NONE',  ( 7.871384613761001070, -5.129340912189999990, 6.740051747100999968 ) ) ;
#43471=CARTESIAN_POINT ( 'NONE',  ( 10.85502524286000003, -2.899999999999999911, 6.518873296399666728 ) ) ;
#43472=CARTESIAN_POINT ( 'NONE',  ( 11.04782425406999913, -5.235403588978999601, 5.041461677707999911 ) ) ;
#43479=CARTESIAN_POINT ( 'NONE',  ( 9.140753410162000492, -5.100000000000000533, 6.175944241622000064 ) ) ;
#43482=CARTESIAN_POINT ( 'NONE',  ( 9.285188841453999586, -5.269672295101000437, 8.747824102203999530 ) ) ;
#43486=CARTESIAN_POINT ( 'NONE',  ( 10.28315099603999982, -2.387772357283999725, 7.684266429524000408 ) ) ;
#43487=CARTESIAN_POINT ( 'NONE',  ( 9.661532504241865382, -5.554291940393154547, 6.696210084226174253 ) ) ;
#43501=CARTESIAN_POINT ( 'NONE',  ( 7.325000000000000178, -4.000000000000000000, 9.239711431703000244 ) ) ;
#43504=CARTESIAN_POINT ( 'NONE',  ( 11.09999999999999964, -5.449702613288000208, -5.124965750789000296 ) ) ;
#43505=EDGE_CURVE ( 'NONE', #53670, #67173, #66713, .T. ) ;
#43506=CIRCLE ( 'NONE', #25638, 1.000000000000000444 ) ;
#43520=CARTESIAN_POINT ( 'NONE',  ( 10.51835931249056699, -5.126777126180352084, -6.752018918863353925 ) ) ;
#43523=CARTESIAN_POINT ( 'NONE',  ( 10.99934110471000004, -5.081022574063999819, 8.239050178861999640 ) ) ;
#43537=CARTESIAN_POINT ( 'NONE',  ( 9.327456490741958817, -3.944521858995455599, 9.238771218640099647 ) ) ;
#43553=CARTESIAN_POINT ( 'NONE',  ( 9.571967469951999874, -4.084684048989999816, 8.946621592834999248 ) ) ;
#43555=CARTESIAN_POINT ( 'NONE',  ( 8.449245559625000013, -5.458705123429999695, 7.456451825584000659 ) ) ;
#43559=CARTESIAN_POINT ( 'NONE',  ( 7.882275234989998935, -4.670605665485999758, 6.328280003999000591 ) ) ;
#43572=CARTESIAN_POINT ( 'NONE',  ( 0.000000000000000000, -5.100000000000000533, 7.500000000000000000 ) ) ;
#43581=CARTESIAN_POINT ( 'NONE',  ( 7.173532264820161153, -2.920499069053410057, 8.329439769247674263 ) ) ;
#43583=ORIENTED_EDGE ( 'NONE', *, *, #49706, .T. ) ;
#43586=EDGE_CURVE ( 'NONE', #17921, #36772, #5213, .T. ) ;
#43588=CARTESIAN_POINT ( 'NONE',  ( 8.449824646308410792, -2.260412847700007610, 7.499181798588557157 ) ) ;
#43597=VECTOR ( 'NONE', #13789, 1000.000000000000227 ) ;
#43601=CARTESIAN_POINT ( 'NONE',  ( 10.76685100253999927, -2.832432432432000269, 6.822293592207000934 ) ) ;
#43602=SURFACE_STYLE_USAGE ( .BOTH. , #59672 ) ;
#43626=ORIENTED_EDGE ( 'NONE', *, *, #38600, .F. ) ;
#43632=CARTESIAN_POINT ( 'NONE',  ( 9.858853446676000942, -2.668079545448999834, -7.206971019603000350 ) ) ;
#43641=CARTESIAN_POINT ( 'NONE',  ( 11.09999999999999964, -2.700469802787999640, -5.124965750789000296 ) ) ;
#43643=CIRCLE ( 'NONE', #32512, 1.099999999999999867 ) ;
#43661=DIRECTION ( 'NONE',  ( 1.000000000000000000, -1.157371756808000041E-14, 1.157371756808000041E-14 ) ) ;
#43667=CARTESIAN_POINT ( 'NONE',  ( 11.12914445903999905, -3.083861519183999977, 8.586004431109000024 ) ) ;
#43668=CARTESIAN_POINT ( 'NONE',  ( 8.705995559625000269, -2.542850487891999745, 7.419808283050000064 ) ) ;
#43672=CARTESIAN_POINT ( 'NONE',  ( 10.94033064679000233, -5.142732045902000948, -6.493502833853999512 ) ) ;
#43673=CARTESIAN_POINT ( 'NONE',  ( 7.807018160663298012, -4.386125006573436735, 9.196209433013514456 ) ) ;
#43674=CARTESIAN_POINT ( 'NONE',  ( 9.719606904206999687, -5.967761543230999166, 7.406644089178000101 ) ) ;
#43676=ORIENTED_EDGE ( 'NONE', *, *, #45625, .T. ) ;
#43691=CARTESIAN_POINT ( 'NONE',  ( 8.817462135714999150, -5.100000000000000533, 6.571291218949999902 ) ) ;
#43693=CARTESIAN_POINT ( 'NONE',  ( 9.523691940378000709, -4.852736108563000528, 8.683927195503999386 ) ) ;
#43704=AXIS2_PLACEMENT_3D ( 'NONE', #46408, #3399, #66340 ) ;
#43719=DIRECTION ( 'NONE',  ( 0.000000000000000000, 0.000000000000000000, -1.000000000000000000 ) ) ;
#43723=LINE ( 'NONE', #28329, #57165 ) ;
#43734=B_SPLINE_CURVE_WITH_KNOTS ( 'NONE', 3,
 ( #27174, #33112, #27871, #6174, #48497 ),
 .UNSPECIFIED., .F., .F.,
 ( 4, 1, 4 ),
 ( 0.000000000000000000, 0.5000000000000000000, 1.000000000000000000 ),
 .UNSPECIFIED. ) ;
#43747=B_SPLINE_CURVE_WITH_KNOTS ( 'NONE', 3,
 ( #13868, #19102, #35198, #56510, #66304, #8616, #29965, #61070, #13189, #51266, #28575, #49890, #7933, #3362 ),
 .UNSPECIFIED., .F., .F.,
 ( 4, 2, 2, 1, 1, 2, 2, 4 ),
 ( 0.000000000000000000, 0.2499999999999955036, 0.3749999999999888978, 0.4374999999999855116, 0.4687499999999806821, 0.4843749999999786282, 0.4999999999999765743, 1.000000000000000000 ),
 .UNSPECIFIED. ) ;
#43752=ORIENTED_EDGE ( 'NONE', *, *, #46571, .T. ) ;
#43765=CARTESIAN_POINT ( 'NONE',  ( 11.28109314679000086, -2.660122028910999692, -6.904120269057000492 ) ) ;
#43767=CARTESIAN_POINT ( 'NONE',  ( 9.529144223516999190, -2.330665094450000030, -8.349943402163999551 ) ) ;
#43775=ORIENTED_EDGE ( 'NONE', *, *, #49105, .F. ) ;
#43779=CARTESIAN_POINT ( 'NONE',  ( 9.861802827889732725, -2.874603711573434417, -6.749639981083136675 ) ) ;
#43783=CARTESIAN_POINT ( 'NONE',  ( 10.26368921839999970, -4.794141574281000295, -8.804455889106000299 ) ) ;
#43785=EDGE_LOOP ( 'NONE', ( #59060, #47242, #68502, #8372, #50659, #20528, #49174 ) ) ;
#43789=AXIS2_PLACEMENT_3D ( 'NONE', #56768, #56418, #68263 ) ;
#43792=FACE_OUTER_BOUND ( 'NONE', #57843, .T. ) ;
#43798=CARTESIAN_POINT ( 'NONE',  ( 10.57223537388000167, -4.020426196685999543, 8.920680607665000039 ) ) ;
#43811=CARTESIAN_POINT ( 'NONE',  ( 9.882901294779998125, -4.314558311729999929, -9.161035779983999205 ) ) ;
#43813=CARTESIAN_POINT ( 'NONE',  ( 9.523148997461001741, -5.167567567567999731, -6.822293592207000934 ) ) ;
#43817=CARTESIAN_POINT ( 'NONE',  ( 8.549163638619971195, -3.170442981555772199, 5.998973939403969169 ) ) ;
#43822=CARTESIAN_POINT ( 'NONE',  ( 10.55944656072999877, -2.874072957412999951, 4.818572726091000291 ) ) ;
#43826=CARTESIAN_POINT ( 'NONE',  ( 10.27814441345999974, -5.521593622715999850, 8.751220666652999469 ) ) ;
#43830=CARTESIAN_POINT ( 'NONE',  ( 10.71756905878999966, -3.040221764047000175, 8.808455607108001573 ) ) ;
#43831=CARTESIAN_POINT ( 'NONE',  ( 9.954831044986722333, -2.229402479047418950, 7.375981937142048750 ) ) ;
#43834=VECTOR ( 'NONE', #42158, 1000.000000000000000 ) ;
#43844=CARTESIAN_POINT ( 'NONE',  ( 8.266851002545999805, -2.832432432432000269, 6.822293592207000934 ) ) ;
#43849=CARTESIAN_POINT ( 'NONE',  ( 7.947784805529094498, -5.286778829772836197, 7.027374276529119612 ) ) ;
#43865=CARTESIAN_POINT ( 'NONE',  ( 9.013429960698999821, -4.933961117404000341, 8.417889755737999025 ) ) ;
#43881=EDGE_CURVE ( 'NONE', #67865, #47885, #67501, .T. ) ;
#43883=CARTESIAN_POINT ( 'NONE',  ( 8.164397154371004106, -4.665396042252996978, 6.167056685642003266 ) ) ;
#43891=CARTESIAN_POINT ( 'NONE',  ( 10.34020413671000149, -4.202027362542999356, 9.459588031742001135 ) ) ;
#43895=EDGE_LOOP ( 'NONE', ( #11445, #23307, #66411, #1167 ) ) ;
#43900=CARTESIAN_POINT ( 'NONE',  ( 9.323728576950999880, -3.947350124452999598, 6.051857392047999440 ) ) ;
#43903=CARTESIAN_POINT ( 'NONE',  ( 8.064120559623999540, -4.228293421747000735, 8.941387937291999322 ) ) ;
#43907=CIRCLE ( 'NONE', #11494, 1.000000000000000000 ) ;
#43916=CARTESIAN_POINT ( 'NONE',  ( 8.224933059623998233, -5.629389383493999865, 8.631822608164000599 ) ) ;
#43919=LINE ( 'NONE', #32733, #32706 ) ;
#43936=CARTESIAN_POINT ( 'NONE',  ( 8.446461008496655154, -2.261511969888099660, 7.573099163943432188 ) ) ;
#43942=CARTESIAN_POINT ( 'NONE',  ( 10.23808992278000041, -2.752437370156000540, 6.820045513931999537 ) ) ;
#43947=ORIENTED_EDGE ( 'NONE', *, *, #40122, .T. ) ;
#43952=CARTESIAN_POINT ( 'NONE',  ( 9.470944094206000585, -5.100000000000000533, 6.571291218949999902 ) ) ;
#43961=VECTOR ( 'NONE', #17754, 999.9999999999998863 ) ;
#43977=CARTESIAN_POINT ( 'NONE',  ( 10.13382174003999836, -5.176455793257000337, -8.189804425074999727 ) ) ;
#43980=CARTESIAN_POINT ( 'NONE',  ( 10.40537527825904007, -5.100000000000000533, -6.445686799541589629 ) ) ;
#43996=CARTESIAN_POINT ( 'NONE',  ( 7.822379440378000481, -4.636725880537000855, 9.378965771357000492 ) ) ;
#43997=CARTESIAN_POINT ( 'NONE',  ( 9.619730517102000888, -2.477793449086000077, -8.275032865112999403 ) ) ;
#44007=CARTESIAN_POINT ( 'NONE',  ( 9.793536308083167441, -2.899999999999999911, 6.665341197420959318 ) ) ;
#44014=CARTESIAN_POINT ( 'NONE',  ( 9.813358178091998951, -5.349400659402999914, 6.657024270273000255 ) ) ;
#44018=CARTESIAN_POINT ( 'NONE',  ( 9.020964430773000586, -2.907392932634000005, 6.146188468825999784 ) ) ;
#44021=CARTESIAN_POINT ( 'NONE',  ( 10.71315564678999976, -2.619204038425999581, -8.142086897834001746 ) ) ;
#44022=CARTESIAN_POINT ( 'NONE',  ( 7.801841845076483040, -4.493699489315019946, 9.169207277517051224 ) ) ;
#44023=CARTESIAN_POINT ( 'NONE',  ( 10.21608469020999976, -5.961703525007000515, 7.319668113368000384 ) ) ;
#44037=CARTESIAN_POINT ( 'NONE',  ( 8.912651967921339846, -2.899999999999999911, 6.383937126463831824 ) ) ;
#44046=CARTESIAN_POINT ( 'NONE',  ( 9.900941392955999731, -4.883847137081999357, -9.070879136699002032 ) ) ;
#44057=ORIENTED_EDGE ( 'NONE', *, *, #15355, .F. ) ;
#44060=CYLINDRICAL_SURFACE ( 'NONE', #52562, 0.4999999999999998335 ) ;
#44069=CARTESIAN_POINT ( 'NONE',  ( 11.09999999999999964, -5.299524241844999928, -5.124965750789000296 ) ) ;
#44087=B_SPLINE_CURVE_WITH_KNOTS ( 'NONE', 3,
 ( #58162, #31598, #5364, #117 ),
 .UNSPECIFIED., .F., .F.,
 ( 4, 4 ),
 ( 0.000000000000000000, 1.000000000000000000 ),
 .UNSPECIFIED. ) ;
#44094=VECTOR ( 'NONE', #39357, 1000.000000000000000 ) ;
#44099=DIRECTION ( 'NONE',  ( 0.000000000000000000, 1.000000000000000000, 0.000000000000000000 ) ) ;
#44112=LINE ( 'NONE', #39899, #5363 ) ;
#44119=LINE ( 'NONE', #64715, #4412 ) ;
#44120=CARTESIAN_POINT ( 'NONE',  ( 10.82674314678999927, -3.167157901876000103, -6.225148200207000215 ) ) ;
#44126=ORIENTED_EDGE ( 'NONE', *, *, #20011, .T. ) ;
#44137=CARTESIAN_POINT ( 'NONE',  ( 9.843620110012999191, -5.021680390140000227, -8.761463725090999688 ) ) ;
#44141=CARTESIAN_POINT ( 'NONE',  ( 10.61675993195453849, -2.980798815563405757, -5.036430362955847784 ) ) ;
#44143=ORIENTED_EDGE ( 'NONE', *, *, #26997, .F. ) ;
#44149=CARTESIAN_POINT ( 'NONE',  ( 11.05166408303000125, -5.150113226472000427, 5.124970633734999836 ) ) ;
#44151=DIRECTION ( 'NONE',  ( 0.000000000000000000, 1.000000000000000000, 0.000000000000000000 ) ) ;
#44153=CARTESIAN_POINT ( 'NONE',  ( 9.388626433405999450, -4.079401915682999480, 9.259353168384000909 ) ) ;
#44165=CARTESIAN_POINT ( 'NONE',  ( 10.04002603384999937, -2.348908096685999869, -7.136751747961000092 ) ) ;
#44169=CARTESIAN_POINT ( 'NONE',  ( 8.615663457454523666, -2.873897790767480753, -6.750856197900089839 ) ) ;
#44170=CARTESIAN_POINT ( 'NONE',  ( 8.566291307401062483, -2.988918445095709142, 6.176011962928662946 ) ) ;
#44175=CARTESIAN_POINT ( 'NONE',  ( 10.95339184458999959, -2.662495063361999925, 4.888666547750000646 ) ) ;
#44176=CARTESIAN_POINT ( 'NONE',  ( 7.682778389973002220, -3.526905737521000006, 6.475916620580998817 ) ) ;
#44179=CARTESIAN_POINT ( 'NONE',  ( 10.58844302970999962, -3.754658547780000521, 5.545362468768000319 ) ) ;
#44182=CARTESIAN_POINT ( 'NONE',  ( 11.18051369187999988, -5.340070732632000272, 8.416150632189001612 ) ) ;
#44183=CARTESIAN_POINT ( 'NONE',  ( 9.743004321115734001, -5.518491777742534410, 8.419011746474035718 ) ) ;
#44199=CARTESIAN_POINT ( 'NONE',  ( 7.768029367744567537, -2.842467755650244232, 6.805004515721170044 ) ) ;
#44201=CARTESIAN_POINT ( 'NONE',  ( 8.253230575588421658, -2.714951384259771228, 7.027308161653141205 ) ) ;
#44222=CARTESIAN_POINT ( 'NONE',  ( 9.020964430773000586, -2.907392932634000005, 6.146188468825999784 ) ) ;
#44225=B_SPLINE_CURVE_WITH_KNOTS ( 'NONE', 3,
 ( #18615, #8466, #40283, #52133 ),
 .UNSPECIFIED., .F., .F.,
 ( 4, 4 ),
 ( 0.000000000000000000, 1.000000000000000000 ),
 .UNSPECIFIED. ) ;
#44229=VERTEX_POINT ( 'NONE', #36870 ) ;
#44258=CARTESIAN_POINT ( 'NONE',  ( 9.509907746701999898, -5.077451867123000007, 8.469011304701000498 ) ) ;
#44260=CARTESIAN_POINT ( 'NONE',  ( 7.678995559621999867, -2.599231861044000169, 7.909347897884000389 ) ) ;
#44266=CARTESIAN_POINT ( 'NONE',  ( 11.09999999999999964, -4.000000000000000000, 7.500000000000000000 ) ) ;
#44287=ORIENTED_EDGE ( 'NONE', *, *, #27623, .F. ) ;
#44292=CARTESIAN_POINT ( 'NONE',  ( 8.581139754955028565, -4.140793541034012648, 5.766079433607869120 ) ) ;
#44308=CARTESIAN_POINT ( 'NONE',  ( 8.936672300099200328, -2.275486823213108245, 7.787304321185041012 ) ) ;
#44310=ORIENTED_EDGE ( 'NONE', *, *, #39639, .F. ) ;
#44313=CIRCLE ( 'NONE', #18603, 10.75000000000000533 ) ;
#44329=CARTESIAN_POINT ( 'NONE',  ( 10.93146935944000120, -2.472881306517999978, -7.514158774805000718 ) ) ;
#44346=CARTESIAN_POINT ( 'NONE',  ( 7.100000000000000533, -2.649999999999999911, 7.500000000000000000 ) ) ;
#44350=CARTESIAN_POINT ( 'NONE',  ( 8.309480646794000336, -2.905864338704999827, 8.940687151810998046 ) ) ;
#44351=CARTESIAN_POINT ( 'NONE',  ( 9.974327024990000012, -5.476443305113000370, -7.051545409824000465 ) ) ;
#44355=VERTEX_POINT ( 'NONE', #49414 ) ;
#44356=VECTOR ( 'NONE', #43661, 1000.000000000000000 ) ;
#44357=CARTESIAN_POINT ( 'NONE',  ( 10.61705858902340971, -5.079493225104016574, -8.329679463145376772 ) ) ;
#44364=AXIS2_PLACEMENT_3D ( 'NONE', #33280, #765, #5317 ) ;
#44367=CARTESIAN_POINT ( 'NONE',  ( 9.910640133503999749, -2.107273866476999657, 7.885282692430999774 ) ) ;
#44374=CARTESIAN_POINT ( 'NONE',  ( 11.14450444037999866, -5.035425715994000129, -8.381528062715000615 ) ) ;
#44375=CARTESIAN_POINT ( 'NONE',  ( 8.093318583063375371, -4.415994369059405678, 5.811304729630019317 ) ) ;
#44376=CARTESIAN_POINT ( 'NONE',  ( 11.25041341105000114, -5.730771985297000271, 8.122672103119001008 ) ) ;
#44390=EDGE_CURVE ( 'NONE', #64636, #61687, #24116, .T. ) ;
#44394=CARTESIAN_POINT ( 'NONE',  ( 7.854816940377000734, -4.561648098548999997, 6.153050355516999304 ) ) ;
#44399=CARTESIAN_POINT ( 'NONE',  ( 9.115000000004000569, -5.349999999999999645, -7.500000000000000000 ) ) ;
#44402=CARTESIAN_POINT ( 'NONE',  ( 8.225195096046189036, -2.649880853682571313, 7.500010424662522546 ) ) ;
#44405=AXIS2_PLACEMENT_3D ( 'NONE', #47494, #20572, #41897 ) ;
#44410=AXIS2_PLACEMENT_3D ( 'NONE', #64689, #31866, #53183 ) ;
#44440=CARTESIAN_POINT ( 'NONE',  ( 9.050000000000000711, -7.679126935408000065, 5.093340497782000043 ) ) ;
#44446=AXIS2_PLACEMENT_3D ( 'NONE', #14005, #12622, #24491 ) ;
#44457=ADVANCED_FACE ( 'NONE', ( #50118 ), #13777, .F. ) ;
#44471=CARTESIAN_POINT ( 'NONE',  ( 10.76587944038000089, -3.166536971515000243, -8.574494061818999313 ) ) ;
#44473=CARTESIAN_POINT ( 'NONE',  ( 10.98768472633000037, -5.449702618601000026, 4.945212061625999134 ) ) ;
#44482=ADVANCED_FACE ( 'NONE', ( #40999 ), #42870, .F. ) ;
#44490=CARTESIAN_POINT ( 'NONE',  ( 9.961463664312999455, -2.787129471086000176, -8.677705025472000955 ) ) ;
#44497=CARTESIAN_POINT ( 'NONE',  ( 10.26948980103999887, -4.629959721010000528, 4.845921682315999846 ) ) ;
#44501=CARTESIAN_POINT ( 'NONE',  ( 10.27968096967000022, -5.739708848514999850, 7.774962785835000112 ) ) ;
#44513=CARTESIAN_POINT ( 'NONE',  ( 10.78636854442000192, -5.666037955714999796, -7.787004779180999314 ) ) ;
#44517=DIRECTION ( 'NONE',  ( 1.000000000000000000, 0.000000000000000000, 0.000000000000000000 ) ) ;
#44519=CARTESIAN_POINT ( 'NONE',  ( 9.130720302798000176, -5.231133027468000130, -6.569831606205999819 ) ) ;
#44525=CARTESIAN_POINT ( 'NONE',  ( 11.00012419157999943, -2.844226485624000045, 5.106573563347000189 ) ) ;
#44530=CARTESIAN_POINT ( 'NONE',  ( 10.96580795178999956, -4.930647899304999804, 6.170539049947000088 ) ) ;
#44533=CARTESIAN_POINT ( 'NONE',  ( 9.882266086202999844, -4.932716797830999589, 6.390980246320999925 ) ) ;
#44534=CARTESIAN_POINT ( 'NONE',  ( 9.759298684490481435, -5.294816862906961852, 8.717541015033191343 ) ) ;
#44541=B_SPLINE_CURVE_WITH_KNOTS ( 'NONE', 3,
 ( #28204, #29601, #61393, #1631 ),
 .UNSPECIFIED., .F., .F.,
 ( 4, 4 ),
 ( 0.000000000000000000, 1.000000000000000000 ),
 .UNSPECIFIED. ) ;
#44544=CARTESIAN_POINT ( 'NONE',  ( 8.753494611379007750, -2.844423643914999023, -6.810303980490998832 ) ) ;
#44545=VECTOR ( 'NONE', #65287, 1000.000000000000114 ) ;
#44546=DIRECTION ( 'NONE',  ( 1.000000000000000000, 0.000000000000000000, 0.000000000000000000 ) ) ;
#44564=ORIENTED_EDGE ( 'NONE', *, *, #46397, .T. ) ;
#44571=CARTESIAN_POINT ( 'NONE',  ( 9.338847651065298905, -5.080747737076881876, -6.285327966759164831 ) ) ;
#44587=CARTESIAN_POINT ( 'NONE',  ( 9.354496976570960243, -3.359497858161771600, 9.117191629812770870 ) ) ;
#44594=CARTESIAN_POINT ( 'NONE',  ( 11.14698053895999941, -5.129799765052999838, 5.886044098803999702 ) ) ;
#44598=EDGE_CURVE ( 'NONE', #33287, #66793, #23251, .T. ) ;
#44604=CARTESIAN_POINT ( 'NONE',  ( 9.758146639703001668, -2.901368778958000050, 6.555068849476000103 ) ) ;
#44605=CARTESIAN_POINT ( 'NONE',  ( 5.599999999999999645, -0.4000000000000000222, 6.406472342878999804 ) ) ;
#44606=CARTESIAN_POINT ( 'NONE',  ( 7.229683059621999419, -2.630475685621000093, 6.995953627589999613 ) ) ;
#44637=CARTESIAN_POINT ( 'NONE',  ( 8.567616298378466055, -3.838977648115872388, 5.766192393133341199 ) ) ;
#44644=CARTESIAN_POINT ( 'NONE',  ( 9.477176340467600824, -5.064601050969631757, 8.332457336712117524 ) ) ;
#44647=ORIENTED_EDGE ( 'NONE', *, *, #15939, .F. ) ;
#44675=CARTESIAN_POINT ( 'NONE',  ( 10.61721988130000049, -5.045606037229999785, -6.386907901056999570 ) ) ;
#44682=CARTESIAN_POINT ( 'NONE',  ( 10.09654241571003119, -5.267280400567660337, -8.036449566519722865 ) ) ;
#44696=CARTESIAN_POINT ( 'NONE',  ( 7.860168146793000687, -2.263562268490999951, 8.007440964304000985 ) ) ;
#44707=ORIENTED_EDGE ( 'NONE', *, *, #21910, .F. ) ;
#44711=CARTESIAN_POINT ( 'NONE',  ( 10.61382642076999971, -3.385081736013999976, 5.849525238167000651 ) ) ;
#44712=CARTESIAN_POINT ( 'NONE',  ( 8.962745559623000347, -5.445226602819000838, 7.703375344019999460 ) ) ;
#44715=CARTESIAN_POINT ( 'NONE',  ( 10.72801694037999987, -3.751276547904999870, -8.836912395451999913 ) ) ;
#44716=CARTESIAN_POINT ( 'NONE',  ( 7.921590741316500761, -2.367433491553081915, 8.106647180208147674 ) ) ;
#44717=CARTESIAN_POINT ( 'NONE',  ( 10.15903154954000165, -4.166415630773999901, 9.114167874391000623 ) ) ;
#44720=ORIENTED_EDGE ( 'NONE', *, *, #32078, .F. ) ;
#44721=CARTESIAN_POINT ( 'NONE',  ( 11.03776785110999903, -5.237767851104999650, 6.571291218949999902 ) ) ;
#44737=CARTESIAN_POINT ( 'NONE',  ( 7.507480646791999668, -3.501517589953999643, 9.055975309745999624 ) ) ;
#44739=ORIENTED_EDGE ( 'NONE', *, *, #59479, .T. ) ;
#44760=CARTESIAN_POINT ( 'NONE',  ( 11.09999999999999964, -0.5000000000000000000, 5.124965750789000296 ) ) ;
#44775=VERTEX_POINT ( 'NONE', #11757 ) ;
#44780=CARTESIAN_POINT ( 'NONE',  ( 8.560879440379000727, -4.228293421747000735, 8.941387937291999322 ) ) ;
#44787=CARTESIAN_POINT ( 'NONE',  ( 11.09049432275999969, -2.710637143123000303, -5.109752498865000270 ) ) ;
#44789=DIRECTION ( 'NONE',  ( 1.000000000000000000, 0.000000000000000000, 0.000000000000000000 ) ) ;
#44792=CARTESIAN_POINT ( 'NONE',  ( 9.421210490158761885, -5.348867133177450661, 7.442204040579022184 ) ) ;
#44797=CARTESIAN_POINT ( 'NONE',  ( 7.420699437778675467, -2.375962897128845785, 8.123829696352604657 ) ) ;
#44800=ORIENTED_EDGE ( 'NONE', *, *, #39187, .T. ) ;
#44815=ORIENTED_EDGE ( 'NONE', *, *, #29333, .T. ) ;
#44819=VERTEX_POINT ( 'NONE', #31137 ) ;
#44828=CARTESIAN_POINT ( 'NONE',  ( 9.910158555493998378, -2.531067292016000003, -7.917737669614999696 ) ) ;
#44835=CARTESIAN_POINT ( 'NONE',  ( 10.27507144281000073, -4.625210729382000174, 5.003494133775000741 ) ) ;
#44837=FACE_OUTER_BOUND ( 'NONE', #18021, .T. ) ;
#44839=CARTESIAN_POINT ( 'NONE',  ( 9.980430903642000473, -4.047223565251000466, 9.090364706348999846 ) ) ;
#44840=ORIENTED_EDGE ( 'NONE', *, *, #68920, .F. ) ;
#44846=CARTESIAN_POINT ( 'NONE',  ( 10.42914842315198243, -5.349767025452218938, 7.570572966693990047 ) ) ;
#44853=VECTOR ( 'NONE', #12663, 1000.000000000000000 ) ;
#44856=CARTESIAN_POINT ( 'NONE',  ( 9.394730517101999467, -2.624921803719999946, -8.200122328058998988 ) ) ;
#44863=CARTESIAN_POINT ( 'NONE',  ( 10.28158534179000050, -3.278999312060000282, 4.850220352478999963 ) ) ;
#44869=CARTESIAN_POINT ( 'NONE',  ( 11.18051369187999988, -5.340070732632000272, 8.416150632189001612 ) ) ;
#44872=CARTESIAN_POINT ( 'NONE',  ( 10.40727044253999978, -3.797905333157999941, 5.889909992361999969 ) ) ;
#44873=CARTESIAN_POINT ( 'NONE',  ( 10.90000000536000080, -2.899999999941999640, -5.157071284930999866 ) ) ;
#44875=EDGE_LOOP ( 'NONE', ( #27494, #23566, #34590, #40308, #68117 ) ) ;
#44883=CARTESIAN_POINT ( 'NONE',  ( 9.617321917839001699, -3.361793157411000266, -5.915550373431999631 ) ) ;
#44894=ORIENTED_EDGE ( 'NONE', *, *, #30497, .T. ) ;
#44895=VECTOR ( 'NONE', #45330, 1000.000000000000000 ) ;
#44902=CARTESIAN_POINT ( 'NONE',  ( 11.09999999999999787, -3.333452946750000478, -8.929141463601279582 ) ) ;
#44906=CARTESIAN_POINT ( 'NONE',  ( 10.90833333333529609, -5.360760283596206932, 7.292330520109904235 ) ) ;
#44908=CARTESIAN_POINT ( 'NONE',  ( 9.323728576950999880, -3.947350124452999598, 6.051857392047999440 ) ) ;
#44914=DIRECTION ( 'NONE',  ( 1.000000000000000000, 0.000000000000000000, 7.522916419415000070E-14 ) ) ;
#44922=EDGE_CURVE ( 'NONE', #6210, #63228, #63220, .T. ) ;
#44923=CARTESIAN_POINT ( 'NONE',  ( 7.602384083408999516, -9.083445339000999041, -5.683146030659999681 ) ) ;
#44928=CARTESIAN_POINT ( 'NONE',  ( 10.87222337084000046, -5.065783434862999535, -5.123851454306000086 ) ) ;
#44941=CARTESIAN_POINT ( 'NONE',  ( 9.199823022402380701, -5.768932760263438375, 7.515113865975768803 ) ) ;
#44942=CARTESIAN_POINT ( 'NONE',  ( 8.770183059623999355, -3.049610585291000042, 6.392533570808999421 ) ) ;
#44946=CARTESIAN_POINT ( 'NONE',  ( 11.12372457444999974, -6.328645827022000070, 5.418228406735999592 ) ) ;
#44947=DIRECTION ( 'NONE',  ( 0.000000000000000000, -1.000000000000000000, 0.000000000000000000 ) ) ;
#44948=ORIENTED_EDGE ( 'NONE', *, *, #28726, .F. ) ;
#44951=CARTESIAN_POINT ( 'NONE',  ( 10.94683815890999945, -2.933330690924000006, -5.178000042639999911 ) ) ;
#44967=CARTESIAN_POINT ( 'NONE',  ( 7.809516811409829451, -3.056020742931339296, 6.488504755083804199 ) ) ;
#44968=CARTESIAN_POINT ( 'NONE',  ( 11.06697824069853375, -2.733021759301466069, 6.467485083839107141 ) ) ;
#44969=CARTESIAN_POINT ( 'NONE',  ( 10.88314899746000108, -5.167567567567999731, 6.822293592207000934 ) ) ;
#44973=CARTESIAN_POINT ( 'NONE',  ( 8.576023037351861333, -4.025143239269920237, 5.760539197808133061 ) ) ;
#44977=CARTESIAN_POINT ( 'NONE',  ( 9.736871746126999128, -2.742172332680000046, 6.839224809731999422 ) ) ;
#44982=EDGE_CURVE ( 'NONE', #5301, #52724, #14183, .T. ) ;
#44986=PLANE ( 'NONE',  #28279 ) ;
#44997=CARTESIAN_POINT ( 'NONE',  ( 8.216851002544000693, -2.832432432432000269, 6.822293592207000934 ) ) ;
#45003=ORIENTED_EDGE ( 'NONE', *, *, #3608, .F. ) ;
#45006=EDGE_CURVE ( 'NONE', #43226, #16623, #19420, .T. ) ;
#45011=EDGE_CURVE ( 'NONE', #60701, #44355, #66579, .T. ) ;
#45013=CARTESIAN_POINT ( 'NONE',  ( 10.10656447933000024, -4.887648864398999926, -6.257283015674000026 ) ) ;
#45020=CARTESIAN_POINT ( 'NONE',  ( 10.66714959198803570, -5.079709024443942234, -8.329714913667055853 ) ) ;
#45021=CARTESIAN_POINT ( 'NONE',  ( 8.883148997460001084, -5.167567567567999731, 6.822293592207000934 ) ) ;
#45032=CARTESIAN_POINT ( 'NONE',  ( 7.330275273710999961, -4.426925773067000414, 9.293310812901001583 ) ) ;
#45037=ORIENTED_EDGE ( 'NONE', *, *, #25253, .F. ) ;
#45047=CARTESIAN_POINT ( 'NONE',  ( 11.09648096125000016, -3.099777420064000033, 6.097103007060000301 ) ) ;
#45052=CARTESIAN_POINT ( 'NONE',  ( 7.914911323226687223, -2.423414753718124093, 8.235095959117245457 ) ) ;
#45053=CONICAL_SURFACE ( 'NONE', #46149, 0.4377388725247000623, 0.7853981633972997312 ) ;
#45054=CARTESIAN_POINT ( 'NONE',  ( 10.96580795178999956, -4.930647899304999804, 6.170539049947000088 ) ) ;
#45061=CARTESIAN_POINT ( 'NONE',  ( 9.120226521874423398, -5.092799636466279090, -6.532201274827058590 ) ) ;
#45063=ORIENTED_EDGE ( 'NONE', *, *, #67214, .F. ) ;
#45066=CARTESIAN_POINT ( 'NONE',  ( 9.974327024990000012, -5.476443305113000370, -7.051545409824000465 ) ) ;
#45068=CARTESIAN_POINT ( 'NONE',  ( 9.433536308084699229, -2.899999999999999911, -6.665341197421564168 ) ) ;
#45074=B_SPLINE_CURVE_WITH_KNOTS ( 'NONE', 3,
 ( #40916, #67475, #29070, #23805 ),
 .UNSPECIFIED., .F., .F.,
 ( 4, 4 ),
 ( 0.000000000000000000, 0.2509294615239107684 ),
 .UNSPECIFIED. ) ;
#45076=ORIENTED_EDGE ( 'NONE', *, *, #13767, .F. ) ;
#45077=CARTESIAN_POINT ( 'NONE',  ( 8.277730646792999636, -4.874569256861000177, 6.119503992241999590 ) ) ;
#45079=ORIENTED_EDGE ( 'NONE', *, *, #58109, .F. ) ;
#45092=VECTOR ( 'NONE', #15760, 1000.000000000000114 ) ;
#45108=EDGE_CURVE ( 'NONE', #51664, #23524, #13231, .T. ) ;
#45114=EDGE_LOOP ( 'NONE', ( #48336, #62043, #12897, #62834 ) ) ;
#45115=AXIS2_PLACEMENT_3D ( 'NONE', #49769, #59213, #44546 ) ;
#45119=CARTESIAN_POINT ( 'NONE',  ( 7.662254440376999653, -2.688354259407999880, 8.140021027181001401 ) ) ;
#45126=CARTESIAN_POINT ( 'NONE',  ( 11.05503063675000064, -2.753313764949999687, -5.052995050064000182 ) ) ;
#45135=CARTESIAN_POINT ( 'NONE',  ( 8.970944094206998898, -5.100000000000000533, 6.571291218949999902 ) ) ;
#45136=CARTESIAN_POINT ( 'NONE',  ( 7.432865048533964014, -2.297794684850921421, 7.857475797735035350 ) ) ;
#45138=CARTESIAN_POINT ( 'NONE',  ( 10.71480780573668312, -2.649489222497538599, 7.676606295960795912 ) ) ;
#45148=CARTESIAN_POINT ( 'NONE',  ( 10.16007944038000055, -4.812966563646999596, -8.526591612524001107 ) ) ;
#45151=EDGE_CURVE ( 'NONE', #16325, #68200, #3131, .T. ) ;
#45152=LINE ( 'NONE', #33279, #8694 ) ;
#45156=ORIENTED_EDGE ( 'NONE', *, *, #55635, .F. ) ;
#45159=ORIENTED_EDGE ( 'NONE', *, *, #24656, .T. ) ;
#45170=CARTESIAN_POINT ( 'NONE',  ( 10.48414299032999963, -4.098653366703000067, -9.351353705206001621 ) ) ;
#45181=CARTESIAN_POINT ( 'NONE',  ( 11.18706725482999964, -3.186788126275999833, 6.232699537089999353 ) ) ;
#45187=DIRECTION ( 'NONE',  ( 1.000000000000000000, 0.000000000000000000, 0.000000000000000000 ) ) ;
#45191=B_SPLINE_SURFACE_WITH_KNOTS ( 'NONE', 3, 3, ( 
 ( #58171, #47688, #10272, #52927 ),
 ( #5023, #42436, #5372, #37189 ),
 ( #58508, #60587, #13396, #2541 ),
 ( #34718, #44863, #34375, #17596 ),
 ( #29131, #33333, #23176, #1509 ),
 ( #34029, #45205, #28789, #66510 ),
 ( #50100, #17944, #43822, #12692 ),
 ( #66169, #55694, #23868, #22827 ),
 ( #7791, #65820, #39264, #44175 ),
 ( #65119, #44525, #27746, #22480 ),
 ( #55342, #7438, #18632, #39961 ) ),
 .UNSPECIFIED., .F., .F., .F.,
 ( 4, 1, 1, 1, 1, 1, 1, 1, 4 ),
 ( 4, 4 ),
 ( -0.01601554030910999973, 0.000000000000000000, 0.06250000000000000000, 0.1250000000000000000, 0.1875000000000000000, 0.2500000000000000000, 0.3125000000000000000, 0.3750000000000000000, 0.4240941240803000056 ),
 ( -0.1689889244683999980, 1.168921279219000020 ),
 .UNSPECIFIED. ) ;
#45194=CARTESIAN_POINT ( 'NONE',  ( 10.90000000346999975, -5.100000000044000892, -5.157071296039999808 ) ) ;
#45205=CARTESIAN_POINT ( 'NONE',  ( 10.42020212696999870, -3.045227368876000096, 4.899674683287999599 ) ) ;
#45209=ORIENTED_EDGE ( 'NONE', *, *, #29333, .F. ) ;
#45212=CARTESIAN_POINT ( 'NONE',  ( 10.59344961228999971, -5.297755890367000120, 8.474197994416998725 ) ) ;
#45217=ORIENTED_EDGE ( 'NONE', *, *, #58109, .T. ) ;
#45226=CARTESIAN_POINT ( 'NONE',  ( 9.526735624254000001, -3.423478821957000040, -6.068694811299999436 ) ) ;
#45232=EDGE_CURVE ( 'NONE', #65709, #10513, #26392, .T. ) ;
#45234=CARTESIAN_POINT ( 'NONE',  ( 9.933148997456999751, -5.167567567567999731, 6.822293592207000934 ) ) ;
#45245=STYLED_ITEM ( 'NONE', ( #40865 ), #42688 ) ;
#45248=CARTESIAN_POINT ( 'NONE',  ( 9.381451725828847898, -5.100000000000000533, -6.394648509984842022 ) ) ;
#45266=CYLINDRICAL_SURFACE ( 'NONE', #56033, 0.5000000000000004441 ) ;
#45272=B_SPLINE_CURVE_WITH_KNOTS ( 'NONE', 3,
 ( #21558, #10383, #69114, #26129, #52690 ),
 .UNSPECIFIED., .F., .F.,
 ( 4, 1, 4 ),
 ( 0.000000000000000000, 0.5000000000000000000, 1.000000000000000000 ),
 .UNSPECIFIED. ) ;
#45274=CARTESIAN_POINT ( 'NONE',  ( 9.013429960698999821, -4.933961117404000341, 8.417889755737999025 ) ) ;
#45281=CARTESIAN_POINT ( 'NONE',  ( 10.73912476064303156, -2.651371201321786941, 7.263709536581201220 ) ) ;
#45288=CARTESIAN_POINT ( 'NONE',  ( 11.12486991174999851, -6.581659117425999739, 5.643192323797999954 ) ) ;
#45290=ORIENTED_EDGE ( 'NONE', *, *, #58779, .F. ) ;
#45291=CARTESIAN_POINT ( 'NONE',  ( 10.97725418964999911, -2.701085748494000072, 4.940122434141000163 ) ) ;
#45296=ORIENTED_EDGE ( 'NONE', *, *, #21218, .T. ) ;
#45309=B_SPLINE_CURVE_WITH_KNOTS ( 'NONE', 3,
 ( #58053, #31833, #10156, #64657 ),
 .UNSPECIFIED., .F., .F.,
 ( 4, 4 ),
 ( 0.000000000000000000, 1.000000000000000000 ),
 .UNSPECIFIED. ) ;
#45325=CARTESIAN_POINT ( 'NONE',  ( 8.406105646793999853, -5.342173944271999986, 8.432314172168000610 ) ) ;
#45328=CARTESIAN_POINT ( 'NONE',  ( 10.44668246007000079, -8.240391359595998111, 6.962948453051999387 ) ) ;
#45330=DIRECTION ( 'NONE',  ( 1.000000000000000000, 0.000000000000000000, 0.000000000000000000 ) ) ;
#45334=CARTESIAN_POINT ( 'NONE',  ( 9.471368011205999693, -2.030678448189000118, 7.549764202121000523 ) ) ;
#45340=ORIENTED_EDGE ( 'NONE', *, *, #11126, .T. ) ;
#45356=CARTESIAN_POINT ( 'NONE',  ( 10.55068143582000140, -2.412180768165999911, -6.919582641217999708 ) ) ;
#45359=CARTESIAN_POINT ( 'NONE',  ( 9.074999999999999289, -4.417172942406000224, 8.783926296998000538 ) ) ;
#45364=CARTESIAN_POINT ( 'NONE',  ( 10.99999218979999860, 0.000000000000000000, -2.784439345760000141E-13 ) ) ;
#45377=CARTESIAN_POINT ( 'NONE',  ( 9.234504440379000201, -5.964711531933999389, 7.776478361891000723 ) ) ;
#45387=CYLINDRICAL_SURFACE ( 'NONE', #20533, 1.350000000000000089 ) ;
#45388=CARTESIAN_POINT ( 'NONE',  ( 9.258050732556000639, -4.895927245463000510, -6.008721945297999412 ) ) ;
#45390=CARTESIAN_POINT ( 'NONE',  ( 10.33537187819000103, -5.153689638257000105, 8.830861236101000600 ) ) ;
#45391=CARTESIAN_POINT ( 'NONE',  ( 11.09999999999999964, -2.685305999535000154, 6.664030027596000494 ) ) ;
#45394=ADVANCED_FACE ( 'NONE', ( #6305 ), #29892, .T. ) ;
#45396=CARTESIAN_POINT ( 'NONE',  ( 10.61442944038000036, -5.287639274524000399, -7.937245019889999753 ) ) ;
#45397=CARTESIAN_POINT ( 'NONE',  ( 7.966961417027972558, -2.304181943332437754, 7.113926501787253720 ) ) ;
#45398=CARTESIAN_POINT ( 'NONE',  ( 9.290195424034999760, -2.377814350880000038, 7.540992175424999999 ) ) ;
#45403=CARTESIAN_POINT ( 'NONE',  ( 10.60972883830999969, -5.134198870706001117, -4.837030643953000641 ) ) ;
#45404=EDGE_CURVE ( 'NONE', #22584, #51958, #8656, .T. ) ;
#45410=CARTESIAN_POINT ( 'NONE',  ( 9.883740731405000091, -5.634417356902000407, -7.003562403358999156 ) ) ;
#45419=CARTESIAN_POINT ( 'NONE',  ( 7.737831853206999178, -5.687202994508999687, 6.847270485579000088 ) ) ;
#45425=CARTESIAN_POINT ( 'NONE',  ( 10.31966935320999923, -4.764591648058999596, -5.997654637741999473 ) ) ;
#45432=CARTESIAN_POINT ( 'NONE',  ( 8.564063803065426583, -5.052895881395312649, 6.264019472755840923 ) ) ;
#45434=( LENGTH_UNIT ( ) NAMED_UNIT ( * ) SI_UNIT ( .MILLI., .METRE. ) );
#45461=CARTESIAN_POINT ( 'NONE',  ( 10.74016332886163383, -5.523909096309798095, 8.356370520113504341 ) ) ;
#45470=CARTESIAN_POINT ( 'NONE',  ( 11.04384236319999957, -1.500344243307999870, 5.035088906224999938 ) ) ;
#45471=DIRECTION ( 'NONE',  ( 0.000000000000000000, 0.2461538461537955413, 0.9692307692307821076 ) ) ;
#45474=CARTESIAN_POINT ( 'NONE',  ( 9.408235422789894997, -5.323194378891031420, 7.228731909742346140 ) ) ;
#45475=CARTESIAN_POINT ( 'NONE',  ( 8.656816940379998826, -5.329429281359999493, 6.027400270608000099 ) ) ;
#45481=CARTESIAN_POINT ( 'NONE',  ( 7.450637537771028995, -2.261141324514762907, 7.466197568434639109 ) ) ;
#45482=VECTOR ( 'NONE', #62960, 1000.000000000000000 ) ;
#45488=CARTESIAN_POINT ( 'NONE',  ( 11.04482279157316604, -2.508505527921017553, -8.445267545976777868 ) ) ;
#45493=CARTESIAN_POINT ( 'NONE',  ( 11.03091694037999915, -5.020463882420000523, -6.601194361798000010 ) ) ;
#45500=VECTOR ( 'NONE', #47718, 1000.000000000000114 ) ;
#45507=EDGE_CURVE ( 'NONE', #2520, #50721, #58971, .T. ) ;
#45510=DIRECTION ( 'NONE',  ( 0.000000000000000000, 0.000000000000000000, -1.000000000000000000 ) ) ;
#45512=CARTESIAN_POINT ( 'NONE',  ( 11.27765354842000001, -3.273798832483999721, 6.368296067120999382 ) ) ;
#45522=CARTESIAN_POINT ( 'NONE',  ( 5.700000000000000178, -0.2999999999999999889, -9.662944685757000940 ) ) ;
#45526=CARTESIAN_POINT ( 'NONE',  ( 9.534903635507999908, -3.030945724184999968, 8.761987396837000119 ) ) ;
#45527=EDGE_LOOP ( 'NONE', ( #58354, #54538, #6921, #34671, #31000 ) ) ;
#45529=VECTOR ( 'NONE', #64913, 1000.000000000000000 ) ;
#45545=CARTESIAN_POINT ( 'NONE',  ( 9.529318513071000751, -2.297586052318000061, -7.360088033824999876 ) ) ;
#45557=CARTESIAN_POINT ( 'NONE',  ( 10.15903154954000165, -4.166415630773999901, 9.114167874391000623 ) ) ;
#45561=PLANE ( 'NONE',  #39952 ) ;
#45572=CARTESIAN_POINT ( 'NONE',  ( 9.795911616191999016, -5.239375073306999475, -6.095351682555999240 ) ) ;
#45587=CARTESIAN_POINT ( 'NONE',  ( 11.09999999999999964, -4.000000000000000000, -7.500000000000000000 ) ) ;
#45596=ORIENTED_EDGE ( 'NONE', *, *, #23269, .F. ) ;
#45609=CARTESIAN_POINT ( 'NONE',  ( 9.409377086007973290, -2.477133334551472110, 8.340513213184692631 ) ) ;
#45617=CARTESIAN_POINT ( 'NONE',  ( 9.352255147285999826, -2.817754448466000206, 6.388456890282999900 ) ) ;
#45619=DIRECTION ( 'NONE',  ( 1.000000000000000000, 0.000000000000000000, 0.000000000000000000 ) ) ;
#45625=EDGE_CURVE ( 'NONE', #48149, #52223, #50691, .T. ) ;
#45626=EDGE_CURVE ( 'NONE', #59620, #7868, #21440, .T. ) ;
#45632=CARTESIAN_POINT ( 'NONE',  ( 11.01655351471000088, -5.424347081247000268, 4.991940595874999609 ) ) ;
#45634=ORIENTED_EDGE ( 'NONE', *, *, #56523, .T. ) ;
#45635=CARTESIAN_POINT ( 'NONE',  ( 10.32998539982999908, -3.095235127366999794, 4.624383164039000071 ) ) ;
#45636=VECTOR ( 'NONE', #64123, 1000.000000000000114 ) ;
#45638=CARTESIAN_POINT ( 'NONE',  ( 10.00107860442999907, -4.626219091573998909, -9.027249334595000008 ) ) ;
#45664=CARTESIAN_POINT ( 'NONE',  ( 10.90638082498000117, -5.227498618488000126, 6.784459667733999666 ) ) ;
#45666=LINE ( 'NONE', #55117, #62991 ) ;
#45667=CARTESIAN_POINT ( 'NONE',  ( 8.213543146793000460, -3.608524635952000459, 5.913372239166000632 ) ) ;
#45674=CARTESIAN_POINT ( 'NONE',  ( 9.101497196731600070, -2.899999999999999911, 6.350512455778112297 ) ) ;
#45677=CARTESIAN_POINT ( 'NONE',  ( 10.65050275296000137, -5.200029647236999786, 5.937716681140000397 ) ) ;
#45686=CARTESIAN_POINT ( 'NONE',  ( 9.073148997461000675, -5.167567567567999731, -6.822293592207000934 ) ) ;
#45698=CARTESIAN_POINT ( 'NONE',  ( 10.31499432720999998, -5.458372854186999135, -8.355103994551999591 ) ) ;
#45700=CARTESIAN_POINT ( 'NONE',  ( 9.626866900951128514, -2.437244704642051119, -6.713792515457897458 ) ) ;
#45704=ADVANCED_FACE ( 'NONE', ( #19505 ), #30016, .T. ) ;
#45711=CARTESIAN_POINT ( 'NONE',  ( 10.90000000000000036, -0.2999999999999999889, -4.902439024389999567 ) ) ;
#45717=ORIENTED_EDGE ( 'NONE', *, *, #22654, .F. ) ;
#45718=CARTESIAN_POINT ( 'NONE',  ( 8.411456853209999807, -3.882020254083999866, 5.870054788755000530 ) ) ;
#45721=DIRECTION ( 'NONE',  ( 1.000000000000000000, 0.000000000000000000, 3.552713678820000309E-14 ) ) ;
#45724=EDGE_CURVE ( 'NONE', #52017, #31558, #40477, .T. ) ;
#45729=ORIENTED_EDGE ( 'NONE', *, *, #58981, .T. ) ;
#45733=CARTESIAN_POINT ( 'NONE',  ( 11.00366278039000001, -2.264082614160999984, 7.798350693290999835 ) ) ;
#45735=ORIENTED_EDGE ( 'NONE', *, *, #701, .F. ) ;
#45737=CARTESIAN_POINT ( 'NONE',  ( 10.34939194037999854, -2.653148377029999949, -7.312413909354000374 ) ) ;
#45738=CARTESIAN_POINT ( 'NONE',  ( 7.931404649784815852, -2.307123594424923319, 7.902069134632180081 ) ) ;
#45739=CARTESIAN_POINT ( 'NONE',  ( 9.352255147285999826, -2.817754448466000206, 6.388456890282999900 ) ) ;
#45747=ORIENTED_EDGE ( 'NONE', *, *, #68687, .F. ) ;
#45748=CARTESIAN_POINT ( 'NONE',  ( 9.795737326637999232, -4.289037785427000316, -5.816478295321999781 ) ) ;
#45755=EDGE_LOOP ( 'NONE', ( #45956, #58807, #26164, #28296, #24932, #29255, #34290, #45063, #52450, #6294 ) ) ;
#45758=CARTESIAN_POINT ( 'NONE',  ( 7.802019353206999241, -5.638700495537999124, 8.266402903491000487 ) ) ;
#45764=CARTESIAN_POINT ( 'NONE',  ( 10.63743064679000128, -3.721475434679999861, -8.997096235511000017 ) ) ;
#45772=CARTESIAN_POINT ( 'NONE',  ( 8.474485200571999499, -5.100000000000000533, 6.560614371780999043 ) ) ;
#45782=CARTESIAN_POINT ( 'NONE',  ( 10.25047016403776823, -3.823336794438516151, -8.849920973562444004 ) ) ;
#45798=CARTESIAN_POINT ( 'NONE',  ( 10.65216644777291854, -5.457257952748706842, 6.517891258330301696 ) ) ;
#45808=CARTESIAN_POINT ( 'NONE',  ( 11.04677151279999947, -2.764386413791999786, -5.039776830043000366 ) ) ;
#45815=CARTESIAN_POINT ( 'NONE',  ( 8.271691940379001906, -5.629389383493999865, 8.631822608164000599 ) ) ;
#45819=CARTESIAN_POINT ( 'NONE',  ( 7.412945637235106133, -2.444942208937388894, 8.282280356623708428 ) ) ;
#45829=CARTESIAN_POINT ( 'NONE',  ( 11.14450444037999866, -5.035425715994000129, -8.381528062715000615 ) ) ;
#45838=VERTEX_POINT ( 'NONE', #61806 ) ;
#45841=CIRCLE ( 'NONE', #33568, 1.949999999999999956 ) ;
#45845=B_SPLINE_CURVE_WITH_KNOTS ( 'NONE', 3,
 ( #11311, #16213, #484, #42107 ),
 .UNSPECIFIED., .F., .F.,
 ( 4, 4 ),
 ( 0.000000000000000000, 1.000000000000000000 ),
 .UNSPECIFIED. ) ;
#45847=CARTESIAN_POINT ( 'NONE',  ( 7.102406491832000235, -0.2966009291953999871, -3.049954386258999950 ) ) ;
#45849=CARTESIAN_POINT ( 'NONE',  ( 10.59303089732000025, -2.436232726560000117, 7.793465286118999913 ) ) ;
#45851=CARTESIAN_POINT ( 'NONE',  ( 10.91623602276999883, -5.459825388708999583, -8.642870457474998602 ) ) ;
#45857=CARTESIAN_POINT ( 'NONE',  ( 10.97044361512000066, -6.159047241444000065, -5.038256385253999881 ) ) ;
#45860=DIRECTION ( 'NONE',  ( -1.000000000000000000, 0.000000000000000000, 0.000000000000000000 ) ) ;
#45863=CARTESIAN_POINT ( 'NONE',  ( 9.910640133503999749, -2.107273866476999657, 7.885282692430999774 ) ) ;
#45889=CARTESIAN_POINT ( 'NONE',  ( 10.99433452212999818, -3.697619272994999928, 5.729306330972000261 ) ) ;
#45893=CARTESIAN_POINT ( 'NONE',  ( 5.700000000000000178, 0.5292307692307999245, -2.083846153846000249 ) ) ;
#45902=CARTESIAN_POINT ( 'NONE',  ( 8.363820752062002484, -3.209969472227002463, -6.508691878251005924 ) ) ;
#45905=CARTESIAN_POINT ( 'NONE',  ( 9.128137413980999426, -5.235394649229000663, -8.110359502241001550 ) ) ;
#45924=EDGE_CURVE ( 'NONE', #50708, #21198, #5485, .T. ) ;
#45929=EDGE_LOOP ( 'NONE', ( #10263, #34527, #32010, #24394 ) ) ;
#45956=ORIENTED_EDGE ( 'NONE', *, *, #58167, .T. ) ;
#45965=CARTESIAN_POINT ( 'NONE',  ( 8.987059360767002403, -5.121592602089997115, -6.365116772834005232 ) ) ;
#45968=CARTESIAN_POINT ( 'NONE',  ( 10.26195629121000152, -3.399999734730999812, 4.591198190832999515 ) ) ;
#45971=CARTESIAN_POINT ( 'NONE',  ( 9.309135711596999485, -5.864995026133001055, -7.324074232821000230 ) ) ;
#45973=CARTESIAN_POINT ( 'NONE',  ( 9.870828026683421186, -2.650036842959835770, -7.402527408165655132 ) ) ;
#45976=CARTESIAN_POINT ( 'NONE',  ( 7.634919074141999218, -4.860412626018001170, 6.427891721055999597 ) ) ;
#45986=CARTESIAN_POINT ( 'NONE',  ( 9.970944094204998720, -5.100000000000000533, 6.571291218949999902 ) ) ;
#45996=CARTESIAN_POINT ( 'NONE',  ( 9.924739995124999936, -5.060461104229999840, 8.686133300732999274 ) ) ;
#45998=CARTESIAN_POINT ( 'NONE',  ( 8.486008579191000933, -3.399999999999999911, 5.976611076844000614 ) ) ;
#45999=CARTESIAN_POINT ( 'NONE',  ( 8.047379440378000126, -4.468370631666999770, 8.882152684713000568 ) ) ;
#46002=EDGE_CURVE ( 'NONE', #60711, #8263, #62318, .T. ) ;
#46006=CARTESIAN_POINT ( 'NONE',  ( 11.03977792510109701, -5.161925716696966759, -8.467638888452240664 ) ) ;
#46012=CARTESIAN_POINT ( 'NONE',  ( 9.719606904206999687, -5.967761543230999166, 7.406644089178000101 ) ) ;
#46016=CARTESIAN_POINT ( 'NONE',  ( 10.64447714202000128, -5.073836261934999925, -8.340686666652999293 ) ) ;
#46036=CARTESIAN_POINT ( 'NONE',  ( 11.19120431613999855, -3.005395205805000192, -6.023553580263000029 ) ) ;
#46044=CARTESIAN_POINT ( 'NONE',  ( 8.271691940379001906, -5.629389383493999865, 8.631822608164000599 ) ) ;
#46050=EDGE_CURVE ( 'NONE', #32140, #48149, #38858, .T. ) ;
#46056=EDGE_CURVE ( 'NONE', #67791, #44355, #31633, .T. ) ;
#46059=CARTESIAN_POINT ( 'NONE',  ( 7.962144353208000069, -4.874569256861000177, 6.119503992241999590 ) ) ;
#46061=CARTESIAN_POINT ( 'NONE',  ( 7.844724262280000637, -4.719412258162999585, 6.357657668295000342 ) ) ;
#46063=ORIENTED_EDGE ( 'NONE', *, *, #1261, .F. ) ;
#46072=CARTESIAN_POINT ( 'NONE',  ( 7.945205862068529967, -5.100061878551159111, 6.648263158528791017 ) ) ;
#46073=CARTESIAN_POINT ( 'NONE',  ( 11.09999999999999964, -5.299839462858000338, -5.135710755876000455 ) ) ;
#46074=VERTEX_POINT ( 'NONE', #5050 ) ;
#46077=CARTESIAN_POINT ( 'NONE',  ( 8.191826018243656193, -5.741591131932793246, 7.347086656645051228 ) ) ;
#46080=ORIENTED_EDGE ( 'NONE', *, *, #53147, .F. ) ;
#46082=CARTESIAN_POINT ( 'NONE',  ( 10.61565784046000083, -5.208090112546999606, -4.717379660883000092 ) ) ;
#46087=CARTESIAN_POINT ( 'NONE',  ( 9.663732219486000474, -2.297586052318000061, -7.360088033824999876 ) ) ;
#46088=CARTESIAN_POINT ( 'NONE',  ( 10.33476917742999923, -3.241264537866999973, -4.626716660091000577 ) ) ;
#46089=CARTESIAN_POINT ( 'NONE',  ( 8.216851002544000693, -2.832432432432000269, 6.822293592207000934 ) ) ;
#46092=EDGE_CURVE ( 'NONE', #15201, #67663, #4721, .T. ) ;
#46099=CARTESIAN_POINT ( 'NONE',  ( 7.609456853206999938, -3.276313010012999793, 5.841993238691999935 ) ) ;
#46104=CARTESIAN_POINT ( 'NONE',  ( 10.01676935320999995, -4.324998011277000565, -9.154075058362000306 ) ) ;
#46114=CARTESIAN_POINT ( 'NONE',  ( 10.26651762500999965, -4.562321397865999550, 4.689499100602000148 ) ) ;
#46138=CARTESIAN_POINT ( 'NONE',  ( 5.699999999579000054, -0.3000000004212000082, -9.662944680462999258 ) ) ;
#46143=CARTESIAN_POINT ( 'NONE',  ( 10.82125723222524449, -4.080988682073267704, 9.237810993546167637 ) ) ;
#46144=CARTESIAN_POINT ( 'NONE',  ( 7.737831853206999178, -5.687202994508999687, 6.847270485579000088 ) ) ;
#46148=ORIENTED_EDGE ( 'NONE', *, *, #19282, .T. ) ;
#46149=AXIS2_PLACEMENT_3D ( 'NONE', #38791, #38088, #5927 ) ;
#46160=CARTESIAN_POINT ( 'NONE',  ( 7.603418146792000343, -5.687202994508999687, 6.847270485579000088 ) ) ;
#46166=CARTESIAN_POINT ( 'NONE',  ( 7.627539246035633269, -5.077375723878345681, 6.132675721286665826 ) ) ;
#46172=CARTESIAN_POINT ( 'NONE',  ( 10.82447135085921097, -5.732128138688877605, -7.156556136856877970 ) ) ;
#46180=ADVANCED_FACE ( 'NONE', ( #62406 ), #57496, .T. ) ;
#46185=ORIENTED_EDGE ( 'NONE', *, *, #65572, .F. ) ;
#46186=EDGE_LOOP ( 'NONE', ( #24017, #25802, #23919, #18721 ) ) ;
#46191=PLANE ( 'NONE',  #2003 ) ;
#46193=CARTESIAN_POINT ( 'NONE',  ( 10.23808992278000041, -2.752437370156000540, 6.820045513931999537 ) ) ;
#46195=CARTESIAN_POINT ( 'NONE',  ( 10.75911128370000114, -4.477561100530000004, -5.708582007447000173 ) ) ;
#46201=CARTESIAN_POINT ( 'NONE',  ( 11.01665855156000084, -5.432782508532000065, -4.991872683331999738 ) ) ;
#46203=DIRECTION ( 'NONE',  ( 1.000000000000000000, 0.000000000000000000, 0.000000000000000000 ) ) ;
#46205=VECTOR ( 'NONE', #36927, 1000.000000000000114 ) ;
#46209=CARTESIAN_POINT ( 'NONE',  ( 10.57893103570000015, -4.649956431060000561, 5.681096060554999383 ) ) ;
#46216=FACE_OUTER_BOUND ( 'NONE', #21603, .T. ) ;
#46219=DIRECTION ( 'NONE',  ( -1.000000000000000000, 0.000000000000000000, 0.000000000000000000 ) ) ;
#46232=EDGE_LOOP ( 'NONE', ( #54420, #45079, #43430, #6994, #1479, #58408 ) ) ;
#46233=AXIS2_PLACEMENT_3D ( 'NONE', #23149, #8457, #13020 ) ;
#46235=CARTESIAN_POINT ( 'NONE',  ( 10.56492304196000021, -4.212244324161999565, 8.933470634735002136 ) ) ;
#46246=CARTESIAN_POINT ( 'NONE',  ( 10.53293305405438218, -4.959011670376446190, -5.009116636279086876 ) ) ;
#46250=AXIS2_PLACEMENT_3D ( 'NONE', #50140, #17279, #38604 ) ;
#46253=CARTESIAN_POINT ( 'NONE',  ( 9.086718600414000591, -4.531444417037000072, -6.133284059228000018 ) ) ;
#46255=CARTESIAN_POINT ( 'NONE',  ( 9.621289888149728853, -3.647081445668406197, 8.849739427182552021 ) ) ;
#46259=ADVANCED_FACE ( 'NONE', ( #57851 ), #65497, .T. ) ;
#46265=VERTEX_POINT ( 'NONE', #64799 ) ;
#46269=VERTEX_POINT ( 'NONE', #43501 ) ;
#46275=DIRECTION ( 'NONE',  ( 0.000000000000000000, 1.000000000000000000, 0.000000000000000000 ) ) ;
#46287=EDGE_CURVE ( 'NONE', #21661, #26111, #50552, .T. ) ;
#46290=CARTESIAN_POINT ( 'NONE',  ( 10.94591266939078267, -8.077553304357570241, -7.023431445364937353 ) ) ;
#46297=CARTESIAN_POINT ( 'NONE',  ( 11.09999999999999964, -5.299524241844999928, -5.124965750789000296 ) ) ;
#46314=CARTESIAN_POINT ( 'NONE',  ( 8.887792786201996975, -4.894798647533995073, -6.157725077911004874 ) ) ;
#46317=CARTESIAN_POINT ( 'NONE',  ( 10.48719816214000033, -2.975817524382000201, -4.781958908427999866 ) ) ;
#46320=CARTESIAN_POINT ( 'NONE',  ( 9.710316810687000810, -2.624921803719999946, -8.200122328058998988 ) ) ;
#46327=CARTESIAN_POINT ( 'NONE',  ( 10.88834686957516418, -2.694378745198784841, -7.104278543674422686 ) ) ;
#46332=VERTEX_POINT ( 'NONE', #34053 ) ;
#46346=CARTESIAN_POINT ( 'NONE',  ( 10.87148543990999983, -5.567571293949000300, 7.772413914480000408 ) ) ;
#46347=ORIENTED_EDGE ( 'NONE', *, *, #30419, .T. ) ;
#46348=CARTESIAN_POINT ( 'NONE',  ( 7.632848000845192438, -2.819393604944880671, 8.180463276640507431 ) ) ;
#46349=CARTESIAN_POINT ( 'NONE',  ( 7.598066940377999678, -3.554853390786000045, 8.889491623367000273 ) ) ;
#46357=CARTESIAN_POINT ( 'NONE',  ( 8.159240506820934158, -3.000393948763773633, 6.388924361663858242 ) ) ;
#46363=CARTESIAN_POINT ( 'NONE',  ( 10.60519595724999853, -5.343977295764999802, -7.731524081231999190 ) ) ;
#46364=CARTESIAN_POINT ( 'NONE',  ( 9.674960421382822418, -2.650268802167429438, 7.499999178247414910 ) ) ;
#46365=VERTEX_POINT ( 'NONE', #33703 ) ;
#46375=CARTESIAN_POINT ( 'NONE',  ( 8.251326917914997949, -4.957166827433998613, 6.172577619222003875 ) ) ;
#46394=AXIS2_PLACEMENT_3D ( 'NONE', #30158, #25234, #51461 ) ;
#46397=EDGE_CURVE ( 'NONE', #7868, #44775, #39289, .T. ) ;
#46403=CARTESIAN_POINT ( 'NONE',  ( 7.935745559623000212, -5.430412429559000387, 7.210798766422999329 ) ) ;
#46405=EDGE_CURVE ( 'NONE', #56474, #27465, #38034, .T. ) ;
#46408=CARTESIAN_POINT ( 'NONE',  ( 27.64127793187000037, -5.599999999999999645, 6.571291218949999902 ) ) ;
#46423=CARTESIAN_POINT ( 'NONE',  ( 8.199057584334923376, -5.747876374591468718, 7.505538406481026215 ) ) ;
#46433=CARTESIAN_POINT ( 'NONE',  ( 9.756901401888999459, -3.283392111224999965, -8.676955243274001361 ) ) ;
#46441=CARTESIAN_POINT ( 'NONE',  ( 10.62947109217999930, -5.100000000000000533, 6.152188490330000370 ) ) ;
#46443=CARTESIAN_POINT ( 'NONE',  ( 7.326308059621999824, -3.394845988290999816, 9.388942682504000103 ) ) ;
#46449=EDGE_CURVE ( 'NONE', #38985, #12348, #8162, .T. ) ;
#46450=CARTESIAN_POINT ( 'NONE',  ( 10.29666814679000097, -2.755511079787000384, -6.622434938646999392 ) ) ;
#46484=EDGE_LOOP ( 'NONE', ( #6511, #57928, #17100, #34429, #63522 ) ) ;
#46488=EDGE_CURVE ( 'NONE', #5900, #28902, #68861, .T. ) ;
#46496=CARTESIAN_POINT ( 'NONE',  ( 10.32332547010959090, -4.027151052029898537, 9.388407014067791323 ) ) ;
#46505=CARTESIAN_POINT ( 'NONE',  ( 5.500000000000000000, -1.406666666667000021, -10.45580168561000001 ) ) ;
#46506=CARTESIAN_POINT ( 'NONE',  ( 7.308879440377999970, -4.847802017252000439, 9.065364004483999594 ) ) ;
#46509=ADVANCED_FACE ( 'NONE', ( #9180 ), #42039, .F. ) ;
#46511=CARTESIAN_POINT ( 'NONE',  ( 11.06205805961999999, -2.154403720901000518, -7.605897512385999981 ) ) ;
#46512=CARTESIAN_POINT ( 'NONE',  ( 7.468325272381751034, -2.307615737728840433, 7.097574564742653358 ) ) ;
#46518=CARTESIAN_POINT ( 'NONE',  ( 10.70559276782025648, -5.069448745120865851, 5.072976836019464031 ) ) ;
#46522=CARTESIAN_POINT ( 'NONE',  ( 9.525000000000000355, -4.417172942406000224, 8.783926296998000538 ) ) ;
#46523=CARTESIAN_POINT ( 'NONE',  ( 10.98745755813032332, -5.203136861518676604, 6.684049838556305190 ) ) ;
#46539=CARTESIAN_POINT ( 'NONE',  ( 10.37026726325999881, -5.571557883540000589, 7.748386351620999868 ) ) ;
#46545=CARTESIAN_POINT ( 'NONE',  ( 7.871384613761001070, -5.129340912189999990, 6.740051747100999968 ) ) ;
#46549=CARTESIAN_POINT ( 'NONE',  ( 11.02039621389999979, -5.798238435757999909, -5.016446396665000584 ) ) ;
#46555=CARTESIAN_POINT ( 'NONE',  ( 10.35616740164000049, -2.777283710737999733, 8.995265811011998736 ) ) ;
#46568=CARTESIAN_POINT ( 'NONE',  ( 9.177304894000000601, -4.588307032459999490, -5.987050435448999508 ) ) ;
#46571=EDGE_CURVE ( 'NONE', #32816, #2080, #16365, .T. ) ;
#46580=B_SPLINE_CURVE_WITH_KNOTS ( 'NONE', 3,
 ( #68961, #53575, #15142, #63711 ),
 .UNSPECIFIED., .F., .F.,
 ( 4, 4 ),
 ( 0.000000000000000000, 1.000000000000000000 ),
 .UNSPECIFIED. ) ;
#46582=CARTESIAN_POINT ( 'NONE',  ( 10.00638553269999953, -5.119272496996000399, 8.420388242270998802 ) ) ;
#46585=CARTESIAN_POINT ( 'NONE',  ( 10.81316193496000011, -3.756072284922999938, 6.071597915422999314 ) ) ;
#46594=CIRCLE ( 'NONE', #11944, 1.250000000000000000 ) ;
#46595=CARTESIAN_POINT ( 'NONE',  ( 10.36409408021999923, -4.600000090830000943, -4.954046131267999087 ) ) ;
#46599=CARTESIAN_POINT ( 'NONE',  ( 8.248383067018009385, -3.479335337562998731, -6.809779439446000282 ) ) ;
#46602=CIRCLE ( 'NONE', #44364, 0.5000000000000001110 ) ;
#46603=CARTESIAN_POINT ( 'NONE',  ( 9.311892889969000109, -5.494586520014999920, -6.370782351137999733 ) ) ;
#46604=CARTESIAN_POINT ( 'NONE',  ( 10.15335805961999860, -3.144986649008000068, -5.860958514434000399 ) ) ;
#46612=ORIENTED_EDGE ( 'NONE', *, *, #9211, .F. ) ;
#46613=CARTESIAN_POINT ( 'NONE',  ( 9.250458951833351762, -3.823380212705907777, -8.850046142581145858 ) ) ;
#46627=AXIS2_PLACEMENT_3D ( 'NONE', #37128, #63684, #31208 ) ;
#46630=VERTEX_POINT ( 'NONE', #19685 ) ;
#46638=CARTESIAN_POINT ( 'NONE',  ( 11.07747771764000078, -8.037387346984001368, -6.930719685002999952 ) ) ;
#46639=ORIENTED_EDGE ( 'NONE', *, *, #21218, .F. ) ;
#46646=CARTESIAN_POINT ( 'NONE',  ( 10.13382174003999836, -5.176455793257000337, -8.189804425074999727 ) ) ;
#46648=ORIENTED_EDGE ( 'NONE', *, *, #45404, .F. ) ;
#46661=ORIENTED_EDGE ( 'NONE', *, *, #53745, .F. ) ;
#46664=CARTESIAN_POINT ( 'NONE',  ( 11.09999999999999964, -6.070676763699000666, 5.236526630994999820 ) ) ;
#46668=CARTESIAN_POINT ( 'NONE',  ( 10.88033927340999973, -5.062718448322000242, 5.083949215177000269 ) ) ;
#46677=ORIENTED_EDGE ( 'NONE', *, *, #14470, .F. ) ;
#46692=VERTEX_POINT ( 'NONE', #38508 ) ;
#46693=CARTESIAN_POINT ( 'NONE',  ( 10.76010362286999822, -4.535387425205000156, 6.001717576299999024 ) ) ;
#46694=ORIENTED_EDGE ( 'NONE', *, *, #15247, .T. ) ;
#46703=CARTESIAN_POINT ( 'NONE',  ( 10.21685100254000034, -2.832432432432000269, 6.822293592207000934 ) ) ;
#46705=CARTESIAN_POINT ( 'NONE',  ( 10.27814441345999974, -5.521593622715999850, 8.751220666652999469 ) ) ;
#46709=CARTESIAN_POINT ( 'NONE',  ( 9.976697000975999430, -4.172225768856000272, -6.147144998063999388 ) ) ;
#46710=CARTESIAN_POINT ( 'NONE',  ( 9.332537864288001472, -2.899999999999999911, 6.571291218949999902 ) ) ;
#46722=CARTESIAN_POINT ( 'NONE',  ( 7.634919074141999218, -4.860412626018001170, 6.427891721055999597 ) ) ;
#46728=CARTESIAN_POINT ( 'NONE',  ( 10.83767365324000131, -5.758089526411000136, -6.911472812823999945 ) ) ;
#46735=ADVANCED_FACE ( 'NONE', ( #54594 ), #53558, .T. ) ;
#46749=CARTESIAN_POINT ( 'NONE',  ( 8.283081853209001366, -2.376522687267000222, 7.686981355459999499 ) ) ;
#46751=CARTESIAN_POINT ( 'NONE',  ( 7.761038909107502271, -3.347566356579097846, 6.284495591795857372 ) ) ;
#46752=VERTEX_POINT ( 'NONE', #37819 ) ;
#46762=CARTESIAN_POINT ( 'NONE',  ( 7.955378155590884681, -4.974460548466400844, 6.453583785422088326 ) ) ;
#46765=CARTESIAN_POINT ( 'NONE',  ( 7.834599687276918800, -4.856173268066945603, 6.415412167053935910 ) ) ;
#46767=CARTESIAN_POINT ( 'NONE',  ( 8.251176002667504505, -5.392147303917279366, 8.543946155412404764 ) ) ;
#46776=CARTESIAN_POINT ( 'NONE',  ( 10.76951263900000022, -2.736336172232000319, -4.838784512614000555 ) ) ;
#46785=CARTESIAN_POINT ( 'NONE',  ( 7.775620559622000272, -4.636725880537000855, 9.378965771357000492 ) ) ;
#46790=CARTESIAN_POINT ( 'NONE',  ( 10.20608185320999972, -2.622355301673999772, -6.528538675937999969 ) ) ;
#46801=ORIENTED_EDGE ( 'NONE', *, *, #39850, .F. ) ;
#46807=DIRECTION ( 'NONE',  ( -1.000000000000000000, 0.000000000000000000, 0.000000000000000000 ) ) ;
#46824=B_SPLINE_CURVE_WITH_KNOTS ( 'NONE', 3,
 ( #3967, #47671, #68630, #20751 ),
 .UNSPECIFIED., .F., .F.,
 ( 4, 4 ),
 ( 0.000000000000000000, 1.000000000000000000 ),
 .UNSPECIFIED. ) ;
#46842=VERTEX_POINT ( 'NONE', #49341 ) ;
#46848=CARTESIAN_POINT ( 'NONE',  ( 7.346668146792000087, -2.374041291348000016, 8.293390875797999939 ) ) ;
#46850=CARTESIAN_POINT ( 'NONE',  ( 9.694277465284496742, -4.746637270850415646, -8.655944162059842739 ) ) ;
#46854=CARTESIAN_POINT ( 'NONE',  ( 7.474209973045660149, -2.340228481589814002, 6.977344112086323769 ) ) ;
#46857=ORIENTED_EDGE ( 'NONE', *, *, #50434, .T. ) ;
#46865=CARTESIAN_POINT ( 'NONE',  ( 10.98478522172274907, -5.203339783596914181, 6.694122711083909216 ) ) ;
#46878=CARTESIAN_POINT ( 'NONE',  ( 9.848253563160000112, -4.436921580929999998, 6.148020168057000134 ) ) ;
#46885=CARTESIAN_POINT ( 'NONE',  ( 10.90076029995999995, -5.100000000044000892, -5.152573207167999492 ) ) ;
#46893=CARTESIAN_POINT ( 'NONE',  ( 10.07771285905000092, -4.622037501707999319, 5.671359981946999973 ) ) ;
#46894=CARTESIAN_POINT ( 'NONE',  ( 9.112942518363999156, -5.100000000000000533, 6.192000867487999827 ) ) ;
#46901=CIRCLE ( 'NONE', #59208, 1.299999999999999822 ) ;
#46902=CARTESIAN_POINT ( 'NONE',  ( 10.53138988903999973, -5.607755226963999640, 7.280101849877000042 ) ) ;
#46906=CARTESIAN_POINT ( 'NONE',  ( 5.000000000000000000, -10.75000000000000000, 0.000000000000000000 ) ) ;
#46910=CARTESIAN_POINT ( 'NONE',  ( 9.355894592352999695, -5.864995026133001055, -7.324074232821000230 ) ) ;
#46922=CARTESIAN_POINT ( 'NONE',  ( 9.820206362952999868, -3.883324525498000224, 6.055606607331999847 ) ) ;
#46926=EDGE_CURVE ( 'NONE', #9447, #21198, #35576, .T. ) ;
#46937=CARTESIAN_POINT ( 'NONE',  ( 8.908091524193990196, -3.442323470413000575, -6.178118798475003004 ) ) ;
#46941=CARTESIAN_POINT ( 'NONE',  ( 10.30480805961999913, -5.828319785709999756, -7.226592660401000678 ) ) ;
#46942=CARTESIAN_POINT ( 'NONE',  ( 11.09999999999999964, -4.000000000000000000, 7.500000000000000000 ) ) ;
#46950=VERTEX_POINT ( 'NONE', #5495 ) ;
#46958=B_SPLINE_CURVE_WITH_KNOTS ( 'NONE', 3,
 ( #36227, #41134, #37259, #68369, #9994 ),
 .UNSPECIFIED., .F., .F.,
 ( 4, 1, 4 ),
 ( 0.000000000000000000, 0.5000000000000000000, 1.000000000000000000 ),
 .UNSPECIFIED. ) ;
#46961=DIRECTION ( 'NONE',  ( 1.000000000000000000, 0.000000000000000000, 0.000000000000000000 ) ) ;
#46975=DIRECTION ( 'NONE',  ( 1.000000000000000000, 0.000000000000000000, 0.000000000000000000 ) ) ;
#46977=ORIENTED_EDGE ( 'NONE', *, *, #27623, .T. ) ;
#46981=CARTESIAN_POINT ( 'NONE',  ( 9.975298369746534277, -5.350379160513648813, 7.499985214262776978 ) ) ;
#46987=CARTESIAN_POINT ( 'NONE',  ( 10.38153277269999997, -2.772136814285999673, -8.408084799892998618 ) ) ;
#46995=DIRECTION ( 'NONE',  ( 0.000000000000000000, 0.8648648648648720183, -0.5020047465136825426 ) ) ;
#46999=CARTESIAN_POINT ( 'NONE',  ( 7.666438387056996540, -3.213133027605000525, 6.349775630263004622 ) ) ;
#47000=ORIENTED_EDGE ( 'NONE', *, *, #46449, .F. ) ;
#47003=CARTESIAN_POINT ( 'NONE',  ( 10.33540755369000053, -3.434008644319000325, -4.713744271798000263 ) ) ;
#47007=ADVANCED_FACE ( 'NONE', ( #63529 ), #50085, .T. ) ;
#47008=DIRECTION ( 'NONE',  ( -1.000000000000000000, 3.552713678678000297E-14, -1.776356839339000149E-14 ) ) ;
#47011=CARTESIAN_POINT ( 'NONE',  ( 8.229954139086000708, -4.681838082657003852, 6.132216288069997745 ) ) ;
#47016=ORIENTED_EDGE ( 'NONE', *, *, #53784, .F. ) ;
#47024=VECTOR ( 'NONE', #35490, 1000.000000000000000 ) ;
#47031=CARTESIAN_POINT ( 'NONE',  ( 9.442085454646999665, -4.742494605615999781, 8.809986937145000141 ) ) ;
#47034=CARTESIAN_POINT ( 'NONE',  ( 8.764831853209999579, -5.808258301303999893, 7.446016267012000256 ) ) ;
#47039=VECTOR ( 'NONE', #16096, 1000.000000000000000 ) ;
#47044=CARTESIAN_POINT ( 'NONE',  ( 9.566960887370999700, -5.215923019114000247, 6.177729435798999802 ) ) ;
#47046=EDGE_CURVE ( 'NONE', #13775, #30230, #35473, .T. ) ;
#47050=CARTESIAN_POINT ( 'NONE',  ( 10.65650106607000147, -5.448187878199999723, -7.015213573792999036 ) ) ;
#47052=EDGE_LOOP ( 'NONE', ( #114, #8452, #10909, #24997, #64391 ) ) ;
#47062=ORIENTED_EDGE ( 'NONE', *, *, #39707, .F. ) ;
#47072=CARTESIAN_POINT ( 'NONE',  ( 9.769471092180999960, -5.100000000000000533, -6.152188490330000370 ) ) ;
#47079=CARTESIAN_POINT ( 'NONE',  ( 7.373066940378000034, -3.394845988290999816, 9.388942682504000103 ) ) ;
#47083=B_SPLINE_CURVE_WITH_KNOTS ( 'NONE', 3,
 ( #11026, #53680, #27116, #48431, #64492, #37937, #59259, #32699, #27453, #48778, #886, #22200, #43537, #64837, #16949, #38280, #59607, #49812, #55058, #18007, #60991, #33743, #50162, #13111, #44587, #66227, #50847, #40353, #34778, #67253, #7159, #34440, #8196, #56087, #2942, #28499, #29546, #29190, #18349, #19026, #61337, #66572, #18691, #50501, #13455, #24622, #40025, #2600, #24275, #61675, #45609, #66915, #55407, #7856, #39672, #55754, #13790, #1923, #23244, #19368, #35122, #23583, #65880 ),
 .UNSPECIFIED., .F., .F.,
 ( 4, 2, 2, 2, 1, 1, 1, 2, 2, 2, 2, 2, 1, 1, 1, 1, 2, 2, 2, 2, 2, 1, 1, 1, 1, 2, 2, 2, 2, 2, 1, 1, 2, 2, 2, 2, 2, 4 ),
 ( 0.000000000000000000, 0.06250000000013906931, 0.09375000000020830559, 0.1093750000002429446, 0.1171875000002602502, 0.1210937500002680495, 0.1230468750002719491, 0.1240234375002725736, 0.1250000000002731981, 0.1875000000003121392, 0.2187500000003317346, 0.2343750000003415046, 0.2421875000003464173, 0.2460937500003494427, 0.2480468750003509415, 0.2490234375003515244, 0.2495117187503518019, 0.2500000000003520517, 0.3125000000003730904, 0.3437500000003835265, 0.3593750000003880229, 0.3671875000003914646, 0.3710937500003949618, 0.3730468750003929634, 0.3740234375003919642, 0.3745117187503915201, 0.3750000000003910205, 0.4375000000003100298, 0.4687500000002691181, 0.4843750000002488010, 0.4921875000002377543, 0.4960937500002333689, 0.4980468750002323697, 0.5000000000002312595, 0.6250000000001735279, 0.7500000000001156852, 0.8750000000000579536, 1.000000000000000000 ),
 .UNSPECIFIED. ) ;
#47092=CARTESIAN_POINT ( 'NONE',  ( 8.796581853210000190, -2.368260286481999710, 7.410200011629000549 ) ) ;
#47100=ORIENTED_EDGE ( 'NONE', *, *, #9073, .T. ) ;
#47111=CARTESIAN_POINT ( 'NONE',  ( 8.288382264724496906, -4.755866256346774179, 9.066382130443654930 ) ) ;
#47121=CARTESIAN_POINT ( 'NONE',  ( 7.763685801543999787, -2.858332342511999968, 6.771142545925000533 ) ) ;
#47125=CARTESIAN_POINT ( 'NONE',  ( 8.650129892594387471, -5.422427387162434442, 6.482324188058413483 ) ) ;
#47132=EDGE_CURVE ( 'NONE', #21322, #34155, #36894, .T. ) ;
#47133=CARTESIAN_POINT ( 'NONE',  ( 7.518870559622000016, -3.206365290996999740, 5.681739161071000410 ) ) ;
#47168=CARTESIAN_POINT ( 'NONE',  ( 9.115728395017272945, -3.733357885829600598, 8.827356134417316369 ) ) ;
#47172=CARTESIAN_POINT ( 'NONE',  ( 11.01356641589999974, -2.786433584103999994, 6.253463831328000211 ) ) ;
#47180=CARTESIAN_POINT ( 'NONE',  ( 10.52052890781999928, -2.899999999999999911, 6.152188490330000370 ) ) ;
#47192=CARTESIAN_POINT ( 'NONE',  ( 8.026331853209001110, -5.601799093797000140, 7.176147756900999930 ) ) ;
#47196=CARTESIAN_POINT ( 'NONE',  ( 10.26694555961999988, -5.500014128486999887, -6.419508248405999318 ) ) ;
#47197=CARTESIAN_POINT ( 'NONE',  ( 7.603848374511878561, -4.618107943694234940, 5.872280490120857621 ) ) ;
#47210=CARTESIAN_POINT ( 'NONE',  ( 10.97843137008999825, -5.235400103863000254, 6.782920672145000829 ) ) ;
#47214=ADVANCED_FACE ( 'NONE', ( #41020 ), #10574, .F. ) ;
#47216=CARTESIAN_POINT ( 'NONE',  ( 9.096071945540000314, -5.102479135096000817, -6.621020973615999061 ) ) ;
#47219=ORIENTED_EDGE ( 'NONE', *, *, #40342, .T. ) ;
#47220=CARTESIAN_POINT ( 'NONE',  ( 10.26195629121000152, -4.600000265269999389, 4.591198190832999515 ) ) ;
#47225=CARTESIAN_POINT ( 'NONE',  ( 10.24478558459999888, -5.265199116477000452, 8.959495174640998982 ) ) ;
#47238=CARTESIAN_POINT ( 'NONE',  ( 10.69031285273999821, -5.903020122789000013, 7.830708506196000229 ) ) ;
#47242=ORIENTED_EDGE ( 'NONE', *, *, #52184, .F. ) ;
#47246=CARTESIAN_POINT ( 'NONE',  ( 11.11845396862999991, -5.767021056207999763, 7.178419201465000121 ) ) ;
#47254=CARTESIAN_POINT ( 'NONE',  ( 10.72180282791710049, -2.874603711572245146, 6.749639981085186591 ) ) ;
#47265=CARTESIAN_POINT ( 'NONE',  ( 10.13050497920000126, -3.092053006542000215, 8.629388195475000245 ) ) ;
#47271=LINE ( 'NONE', #10542, #31972 ) ;
#47274=EDGE_CURVE ( 'NONE', #16661, #7255, #14668, .T. ) ;
#47279=CARTESIAN_POINT ( 'NONE',  ( 9.606596480940037708, -5.179845537100731256, -8.180011290786715961 ) ) ;
#47285=CARTESIAN_POINT ( 'NONE',  ( 10.88932069782000056, -2.940686056611999888, -5.040625135843000315 ) ) ;
#47309=DIRECTION ( 'NONE',  ( 1.000000000000000000, 0.000000000000000000, 0.000000000000000000 ) ) ;
#47331=CARTESIAN_POINT ( 'NONE',  ( 9.898134631442999876, -2.965923230546999800, -6.610863544715000373 ) ) ;
#47343=CARTESIAN_POINT ( 'NONE',  ( 8.149001627428001271, -3.121156835630000348, 6.130053226229998486 ) ) ;
#47349=CARTESIAN_POINT ( 'NONE',  ( 10.49785673611999925, -3.776281940467000275, 5.717636230565000588 ) ) ;
#47374=CARTESIAN_POINT ( 'NONE',  ( 11.09999999999999964, -2.700000000000000178, -5.157071250680000496 ) ) ;
#47375=DIRECTION ( 'NONE',  ( -0.7071067811865474617, -0.7071067811865474617, 1.247903205617082848E-09 ) ) ;
#47379=CARTESIAN_POINT ( 'NONE',  ( 10.41185831014999863, -2.101597930377999912, 7.856264717901999539 ) ) ;
#47381=CARTESIAN_POINT ( 'NONE',  ( 7.570242946765014302, -3.646570892123639052, 8.816260394360254438 ) ) ;
#47382=CARTESIAN_POINT ( 'NONE',  ( 7.454683059621999952, -2.138201851198999748, 6.814774777484000623 ) ) ;
#47390=CARTESIAN_POINT ( 'NONE',  ( 10.74609562913000005, -4.263104965433000437, 9.276976808608999647 ) ) ;
#47394=CIRCLE ( 'NONE', #60761, 10.55000000000000249 ) ;
#47395=CARTESIAN_POINT ( 'NONE',  ( 5.000000000000000000, 0.000000000000000000, 0.000000000000000000 ) ) ;
#47403=DIRECTION ( 'NONE',  ( -1.000000000000000000, 0.000000000000000000, 0.000000000000000000 ) ) ;
#47408=ORIENTED_EDGE ( 'NONE', *, *, #33310, .F. ) ;
#47421=CARTESIAN_POINT ( 'NONE',  ( 9.362879440377000151, -3.677416446733000388, 9.250734868033999803 ) ) ;
#47432=CARTESIAN_POINT ( 'NONE',  ( 8.829019353210000531, -5.290204991635000020, 8.768102264518001121 ) ) ;
#47433=CARTESIAN_POINT ( 'NONE',  ( 8.449245559625000013, -5.458705123429999695, 7.456451825584000659 ) ) ;
#47435=EDGE_CURVE ( 'NONE', #40911, #18837, #30516, .T. ) ;
#47444=ORIENTED_EDGE ( 'NONE', *, *, #6916, .F. ) ;
#47446=CARTESIAN_POINT ( 'NONE',  ( 9.213943921932887804, -5.010983041355907552, -6.200064497110663986 ) ) ;
#47448=CARTESIAN_POINT ( 'NONE',  ( 9.924988015501654104, -5.349815781278972615, 7.500001845592777272 ) ) ;
#47454=CARTESIAN_POINT ( 'NONE',  ( 8.265659026604867066, -5.174540709378380399, 8.786794945891818642 ) ) ;
#47473=ORIENTED_EDGE ( 'NONE', *, *, #2833, .F. ) ;
#47475=CARTESIAN_POINT ( 'NONE',  ( 8.738433059624998833, -5.414909314743000301, 8.890670256079998168 ) ) ;
#47494=CARTESIAN_POINT ( 'NONE',  ( 11.04384236319999957, -1.500234901393999731, -5.035088906224999938 ) ) ;
#47502=CARTESIAN_POINT ( 'NONE',  ( 8.616332388160998335, -5.167567399848000065, -6.822293593032000558 ) ) ;
#47515=ORIENTED_EDGE ( 'NONE', *, *, #26522, .T. ) ;
#47519=EDGE_CURVE ( 'NONE', #59694, #15201, #22071, .T. ) ;
#47526=B_SPLINE_CURVE_WITH_KNOTS ( 'NONE', 3,
 ( #68657, #63756, #31616, #32648 ),
 .UNSPECIFIED., .F., .F.,
 ( 4, 4 ),
 ( 0.000000000000000000, 1.000000000000000000 ),
 .UNSPECIFIED. ) ;
#47533=PLANE ( 'NONE',  #49189 ) ;
#47538=CARTESIAN_POINT ( 'NONE',  ( 9.514108112060000622, -4.887639888682999256, 8.462756667353000140 ) ) ;
#47539=CARTESIAN_POINT ( 'NONE',  ( 9.117519353207999444, -4.954907757874000396, 8.825780921426000347 ) ) ;
#47544=B_SPLINE_CURVE_WITH_KNOTS ( 'NONE', 3,
 ( #16627, #37953, #59273, #22559, #38646, #59970, #12078, #33411, #51541, #67608, #40708, #50864, #3637, #40039, #3304, #24638 ),
 .UNSPECIFIED., .F., .F.,
 ( 4, 2, 2, 2, 1, 2, 1, 2, 4 ),
 ( 0.3333669949959171541, 0.4166961206214276348, 0.5000252462469381154, 0.5833543718724485405, 0.6666834974979589656, 0.7500126231234691687, 0.8333417487489794828, 0.9166708743744896859, 1.000000000000000000 ),
 .UNSPECIFIED. ) ;
#47545=CARTESIAN_POINT ( 'NONE',  ( 7.575903374750492247, -4.040870700566189022, 5.761292496191131818 ) ) ;
#47560=B_SPLINE_CURVE_WITH_KNOTS ( 'NONE', 3,
 ( #28770, #54631, #55677, #64755, #7775, #38197, #39244, #44846, #28418 ),
 .UNSPECIFIED., .F., .F.,
 ( 4, 1, 1, 1, 1, 1, 4 ),
 ( 0.1253844953241992632, 0.1696563387730770645, 0.3365447927375280202, 0.5034332467025710578, 0.6703217006676136513, 0.8372101546320646070, 0.8746253901980668433 ),
 .UNSPECIFIED. ) ;
#47564=ORIENTED_EDGE ( 'NONE', *, *, #32749, .F. ) ;
#47573=CARTESIAN_POINT ( 'NONE',  ( 9.409421956854998825, -2.113407700033000047, 7.914197133433000353 ) ) ;
#47582=AXIS2_PLACEMENT_3D ( 'NONE', #66170, #3235, #34719 ) ;
#47583=LINE ( 'NONE', #68888, #45092 ) ;
#47594=CARTESIAN_POINT ( 'NONE',  ( 9.137549407199999862, -2.995696424181999884, 8.544763501938000161 ) ) ;
#47600=CARTESIAN_POINT ( 'NONE',  ( 9.575903104272999400, -2.330665094450000030, -8.349943402163999551 ) ) ;
#47615=CARTESIAN_POINT ( 'NONE',  ( 7.000000000000000000, 1.250000000000000000, 0.000000000000000000 ) ) ;
#47631=DIRECTION ( 'NONE',  ( 1.000000000000000000, 0.000000000000000000, 0.000000000000000000 ) ) ;
#47632=CARTESIAN_POINT ( 'NONE',  ( 10.83488305961999920, -5.800181157098999840, -7.920538492179999501 ) ) ;
#47633=CARTESIAN_POINT ( 'NONE',  ( 9.070134780760179538, -3.647129767632641517, 8.851447081754429291 ) ) ;
#47634=CARTESIAN_POINT ( 'NONE',  ( 7.883148997456999929, -5.167567567567999731, 6.822293592207000934 ) ) ;
#47645=ORIENTED_EDGE ( 'NONE', *, *, #4519, .T. ) ;
#47648=CARTESIAN_POINT ( 'NONE',  ( 9.996463691907599980, -5.100000000000000533, -6.665341197393335193 ) ) ;
#47662=ADVANCED_FACE ( 'NONE', ( #23282 ), #20914, .F. ) ;
#47664=DIRECTION ( 'NONE',  ( 0.000000000000000000, 0.2461538461537955136, -0.9692307692307821076 ) ) ;
#47666=CARTESIAN_POINT ( 'NONE',  ( 9.009273505393998960, -8.692577137281000788, -6.276257937540999698 ) ) ;
#47671=CARTESIAN_POINT ( 'NONE',  ( 8.428197172116432156, -5.125396288428772706, 6.749639981086941631 ) ) ;
#47677=CARTESIAN_POINT ( 'NONE',  ( 10.93146935944000120, -2.472881306517999978, -7.514158774805000718 ) ) ;
#47688=CARTESIAN_POINT ( 'NONE',  ( 10.27190963261000078, -3.431500491711999778, 4.846768348291999651 ) ) ;
#47689=DIRECTION ( 'NONE',  ( 0.000000000000000000, -1.000000000000000000, 0.000000000000000000 ) ) ;
#47692=CARTESIAN_POINT ( 'NONE',  ( 8.268606633798000871, -2.876811830795998670, 6.331441650266997456 ) ) ;
#47696=CARTESIAN_POINT ( 'NONE',  ( 10.52638330645999964, -2.451090818816000105, 6.282756943804999494 ) ) ;
#47705=CARTESIAN_POINT ( 'NONE',  ( 10.27427156480999848, -3.399999787207999447, 4.944156960757000618 ) ) ;
#47714=ORIENTED_EDGE ( 'NONE', *, *, #42633, .F. ) ;
#47715=CARTESIAN_POINT ( 'NONE',  ( 9.523148997461001741, -5.167567567567999731, -6.822293592207000934 ) ) ;
#47717=LINE ( 'NONE', #38244, #62728 ) ;
#47718=DIRECTION ( 'NONE',  ( 0.7660444431195991832, 0.000000000000000000, 0.6427876096857990662 ) ) ;
#47719=CARTESIAN_POINT ( 'NONE',  ( 27.64127793187000037, -3.399999999999999911, -4.505338571134999803 ) ) ;
#47722=VECTOR ( 'NONE', #15115, 1000.000000000000227 ) ;
#47723=CARTESIAN_POINT ( 'NONE',  ( 9.353731048338000065, -2.823575173856999410, 9.032043499493001448 ) ) ;
#47727=CARTESIAN_POINT ( 'NONE',  ( 7.262120559621999760, -4.847802017252000439, 9.065364004483999594 ) ) ;
#47734=DIRECTION ( 'NONE',  ( -0.5298945030329009764, -0.5996714969964009878, -0.5996715028627009891 ) ) ;
#47737=CARTESIAN_POINT ( 'NONE',  ( 9.786673210037999837, -2.381198102024000285, 7.612749732462000374 ) ) ;
#47739=LINE ( 'NONE', #36551, #4837 ) ;
#47740=ORIENTED_EDGE ( 'NONE', *, *, #34508, .F. ) ;
#47744=CARTESIAN_POINT ( 'NONE',  ( 9.828885904259971440, -2.649665795077092323, -7.263400371928318222 ) ) ;
#47751=CIRCLE ( 'NONE', #58922, 0.8000000000000000444 ) ;
#47752=B_SPLINE_SURFACE_WITH_KNOTS ( 'NONE', 3, 3, ( 
 ( #40599, #4215, #39923, #36037, #8101, #24865, #25553, #46878, #8786, #51433, #51094, #57353, #3530, #30799, #46193, #61924, #18937, #35026, #9457, #62598, #14039, #67504, #35365, #3870, #14722, #56687, #35705, #19621, #40943, #62264, #56341, #8444, #41290, #45512, #67158 ),
 ( #40261, #14385, #3197, #61581, #67845, #52112, #24524, #57022, #13697, #29445, #18597, #51772, #19270, #9122, #30460, #66824, #61242, #25204, #46539, #19967, #13357, #34683, #45849, #55997, #50751, #2848, #24176, #47913, #350, #63969, #26932, #20650, #32519, #10496, #31158 ),
 ( #63281, #37414, #41976, #31488, #37756, #26592, #26245, #37078, #48246, #10, #4904, #15411, #21332, #52811, #59082, #20995, #42331, #32183, #36737, #58056, #10159, #42661, #5932, #10841, #16083, #64309, #16427, #5254, #41630, #62936, #58735, #11183, #53498, #5588, #21667 ),
 ( #31836, #63633, #36383, #43002, #47573, #53835, #27274, #68186, #68878, #20304, #15750, #58390, #15060, #53152, #57699, #9809, #52460, #4555, #25896, #47225, #68528, #38095, #11870, #60466, #49278, #59769, #17473, #48597, #11519, #54176, #33210, #23408, #22012, #28305, #12229 ) ),
 .UNSPECIFIED., .F., .F., .F.,
 ( 4, 4 ),
 ( 4, 1, 1, 1, 1, 1, 1, 1, 1, 1, 1, 1, 1, 1, 1, 1, 1, 1, 1, 1, 1, 1, 1, 1, 1, 1, 1, 1, 1, 1, 1, 1, 4 ),
 ( -0.1039086239011999951, 1.103908623900999864 ),
 ( -0.01735257130020999988, 0.01084535706264999969, 0.03904328542550000031, 0.06724121378835999641, 0.09543914215121999944, 0.1236370705141000004, 0.1518349988768999959, 0.1800329272397999947, 0.2082308556026999935, 0.2364287839655000167, 0.2646267123283999601, 0.2928246406912000110, 0.3210225690540999821, 0.3492204974169000331, 0.3774184257798000042, 0.4056163541427000307, 0.4338142825054999707, 0.4620122108683999973, 0.4902101392311999928, 0.5184080675940999638, 0.5466059959569999904, 0.5748039243197999859, 0.6030018526827000125, 0.6311997810455000080, 0.6593977094084000345, 0.6875956377712000300, 0.7157935661340999456, 0.7439914944969999722, 0.7721894228597999676, 0.8003873512226999942, 0.8285852795854999897, 0.8567832079484000163, 0.8849811363112999318 ),
 .UNSPECIFIED. ) ;
#47756=CARTESIAN_POINT ( 'NONE',  ( 8.046447522772005811, -5.096470895078004659, 6.454903582004997808 ) ) ;
#47773=CARTESIAN_POINT ( 'NONE',  ( 8.528441940379998698, -2.472358291268000219, 6.234202627038999189 ) ) ;
#47776=B_SPLINE_CURVE_WITH_KNOTS ( 'NONE', 3,
 ( #11578, #55977, #28728, #14021, #61562, #65763 ),
 .UNSPECIFIED., .F., .F.,
 ( 4, 2, 4 ),
 ( 0.000000000000000000, 0.5000000000000000000, 1.000000000000000000 ),
 .UNSPECIFIED. ) ;
#47779=CARTESIAN_POINT ( 'NONE',  ( 10.70577346828306453, -5.100000000000000533, -6.304440314035878679 ) ) ;
#47786=CARTESIAN_POINT ( 'NONE',  ( 8.700644353210000403, -5.212258818969000451, 6.157189191035000064 ) ) ;
#47807=CARTESIAN_POINT ( 'NONE',  ( 8.535636967035518552, -3.193321067437692840, 5.957063580949454540 ) ) ;
#47815=CARTESIAN_POINT ( 'NONE',  ( 11.09378572506000005, -2.399999999999999911, 6.571291218949999902 ) ) ;
#47819=CARTESIAN_POINT ( 'NONE',  ( 8.852395121421350765, -3.390746510554502713, 9.167721567650527703 ) ) ;
#47821=ORIENTED_EDGE ( 'NONE', *, *, #20011, .F. ) ;
#47825=CARTESIAN_POINT ( 'NONE',  ( 8.224933059623998233, -5.629389383493999865, 8.631822608164000599 ) ) ;
#47827=ORIENTED_EDGE ( 'NONE', *, *, #45507, .F. ) ;
#47862=CARTESIAN_POINT ( 'NONE',  ( 9.215338062334547331, -2.659994556414565725, 7.664869024387687801 ) ) ;
#47867=CARTESIAN_POINT ( 'NONE',  ( 11.09999999999999964, -4.000000000000000000, -7.500000000000000000 ) ) ;
#47883=CARTESIAN_POINT ( 'NONE',  ( 10.48164908029000131, -4.022873587130999518, 9.090901241422999490 ) ) ;
#47884=CARTESIAN_POINT ( 'NONE',  ( 7.293870559621999483, -3.416208448044999901, 6.162501393933999871 ) ) ;
#47885=VERTEX_POINT ( 'NONE', #22757 ) ;
#47888=CARTESIAN_POINT ( 'NONE',  ( 9.900941392955999731, -4.883847137081999357, -9.070879136699002032 ) ) ;
#47889=CARTESIAN_POINT ( 'NONE',  ( 7.734707008367833758, -5.578007308158791311, 8.234535370972333013 ) ) ;
#47907=CARTESIAN_POINT ( 'NONE',  ( 5.700000000000000178, -1.300000000000000044, 9.662944685757000940 ) ) ;
#47910=CARTESIAN_POINT ( 'NONE',  ( 10.90000000296000060, -5.100000000009000445, 5.160242730682999657 ) ) ;
#47913=CARTESIAN_POINT ( 'NONE',  ( 10.87148543990999983, -5.567571293949000300, 7.772413914480000408 ) ) ;
#47919=EDGE_CURVE ( 'NONE', #17344, #18643, #12626, .T. ) ;
#47927=CARTESIAN_POINT ( 'NONE',  ( 9.237253426484580032, -2.665099273114828193, 7.298819532238196572 ) ) ;
#47933=CARTESIAN_POINT ( 'NONE',  ( 9.944325809452999820, -5.443013936195000291, 7.367349259341000156 ) ) ;
#47949=CIRCLE ( 'NONE', #2191, 10.55000000000000426 ) ;
#47971=CARTESIAN_POINT ( 'NONE',  ( 10.03977055961999909, -2.255583827894000137, -8.111980070942999888 ) ) ;
#47995=ORIENTED_EDGE ( 'NONE', *, *, #53264, .F. ) ;
#48009=CARTESIAN_POINT ( 'NONE',  ( 8.396419424012274035, -5.286796060078613912, 7.027454876807410322 ) ) ;
#48013=CARTESIAN_POINT ( 'NONE',  ( 10.34225158793000077, -3.348983461003999906, -8.881464249475000017 ) ) ;
#48018=CARTESIAN_POINT ( 'NONE',  ( 10.90000000000000036, -1.300000000000000044, -10.66294468575417120 ) ) ;
#48020=CARTESIAN_POINT ( 'NONE',  ( 5.699999999579000054, -0.3000000004212000082, -9.662944680462999258 ) ) ;
#48028=CARTESIAN_POINT ( 'NONE',  ( 8.166819129144998968, -2.890362633264002667, 6.359808956951005676 ) ) ;
#48031=CARTESIAN_POINT ( 'NONE',  ( 11.02286109245999945, -2.398753588646000079, 6.352476128646999065 ) ) ;
#48032=CARTESIAN_POINT ( 'NONE',  ( 9.878359312497996925, -5.126777126181800703, 6.752018918865849706 ) ) ;
#48042=VERTEX_POINT ( 'NONE', #23521 ) ;
#48049=CARTESIAN_POINT ( 'NONE',  ( 8.728568342702292426, -2.857753672535667366, -6.775205634707461400 ) ) ;
#48056=CARTESIAN_POINT ( 'NONE',  ( 10.81905590578999998, -2.899999999999999911, -6.571291218949999902 ) ) ;
#48059=ORIENTED_EDGE ( 'NONE', *, *, #9794, .F. ) ;
#48060=CARTESIAN_POINT ( 'NONE',  ( 10.07771285905000092, -4.622037501707999319, 5.671359981946999973 ) ) ;
#48064=CARTESIAN_POINT ( 'NONE',  ( 8.315519353208999931, -5.485781663882000281, 8.532068390166999805 ) ) ;
#48066=ORIENTED_EDGE ( 'NONE', *, *, #65815, .T. ) ;
#48072=CARTESIAN_POINT ( 'NONE',  ( 10.00137895011999944, -3.855365288061999962, 5.709482985498999241 ) ) ;
#48076=LINE ( 'NONE', #59245, #9118 ) ;
#48077=CARTESIAN_POINT ( 'NONE',  ( 10.91732944037999964, -3.256268970540999952, -6.361552695759000287 ) ) ;
#48080=CARTESIAN_POINT ( 'NONE',  ( 7.674792391072008613, -2.650477653308784376, 7.499986425013215552 ) ) ;
#48095=CARTESIAN_POINT ( 'NONE',  ( 11.09999999999999964, -5.350000000000000533, 7.500000000000000000 ) ) ;
#48108=CARTESIAN_POINT ( 'NONE',  ( 7.191894353207000101, -3.501517589953999643, 9.055975309745999624 ) ) ;
#48117=ORIENTED_EDGE ( 'NONE', *, *, #62115, .T. ) ;
#48118=CARTESIAN_POINT ( 'NONE',  ( 7.609456853206999938, -3.276313010012999793, 5.841993238691999935 ) ) ;
#48119=CARTESIAN_POINT ( 'NONE',  ( 8.577620559625000141, -3.981661727120999750, 8.959239802162999311 ) ) ;
#48133=CARTESIAN_POINT ( 'NONE',  ( 7.955340622697639752, -4.963707560450432155, 6.442270077056470257 ) ) ;
#48140=CARTESIAN_POINT ( 'NONE',  ( 8.416338094939373349, -2.406415503492966845, 8.196916887838668231 ) ) ;
#48145=ORIENTED_EDGE ( 'NONE', *, *, #45924, .T. ) ;
#48149=VERTEX_POINT ( 'NONE', #20336 ) ;
#48171=ORIENTED_EDGE ( 'NONE', *, *, #62265, .F. ) ;
#48172=CARTESIAN_POINT ( 'NONE',  ( 7.642284736835422088, -9.077862420372133201, 5.774202551531083749 ) ) ;
#48173=ORIENTED_EDGE ( 'NONE', *, *, #10045, .T. ) ;
#48176=B_SPLINE_CURVE_WITH_KNOTS ( 'NONE', 3,
 ( #27692, #23126, #65064, #38872, #55295 ),
 .UNSPECIFIED., .F., .F.,
 ( 4, 1, 4 ),
 ( 0.000000000000000000, 0.5000000000000000000, 1.000000000000000000 ),
 .UNSPECIFIED. ) ;
#48190=CARTESIAN_POINT ( 'NONE',  ( 11.09999999999999964, -2.700158290619000034, -5.135706284511000419 ) ) ;
#48213=CARTESIAN_POINT ( 'NONE',  ( 9.701976361057999654, -3.399137684422000039, 6.026753338319999820 ) ) ;
#48214=CARTESIAN_POINT ( 'NONE',  ( 8.732394353210001015, -2.806079842068999852, 8.615883328687999665 ) ) ;
#48218=ADVANCED_FACE ( 'NONE', ( #11555 ), #1083, .T. ) ;
#48220=CARTESIAN_POINT ( 'NONE',  ( 10.44811814679000150, -5.235603901491000300, -6.609968500665999613 ) ) ;
#48221=CARTESIAN_POINT ( 'NONE',  ( 7.855373981381045034, -3.323613655148000667, 9.112573541682413847 ) ) ;
#48222=CARTESIAN_POINT ( 'NONE',  ( 10.15402496696000156, -5.267980706381999667, 5.992344456606999437 ) ) ;
#48237=CARTESIAN_POINT ( 'NONE',  ( 7.555275273711000494, -4.314043295739000250, 8.819145559946001356 ) ) ;
#48240=CARTESIAN_POINT ( 'NONE',  ( 10.11344336607715988, -2.323991353769818247, -6.990216894119677171 ) ) ;
#48246=CARTESIAN_POINT ( 'NONE',  ( 9.722771884505998941, -5.493781611190000191, 6.566828939965000167 ) ) ;
#48268=CARTESIAN_POINT ( 'NONE',  ( 10.75110221171000013, -2.822135527917999820, 6.655890318096999714 ) ) ;
#48307=CARTESIAN_POINT ( 'NONE',  ( 10.63743064679000128, -3.721475434679999861, -8.997096235511000017 ) ) ;
#48314=ORIENTED_EDGE ( 'NONE', *, *, #39934, .T. ) ;
#48331=VERTEX_POINT ( 'NONE', #18200 ) ;
#48336=ORIENTED_EDGE ( 'NONE', *, *, #22188, .T. ) ;
#48351=CARTESIAN_POINT ( 'NONE',  ( 10.40558062080000035, -5.599331384652000310, -8.437753779290000367 ) ) ;
#48352=ADVANCED_FACE ( 'NONE', ( #55948 ), #33422, .T. ) ;
#48357=CARTESIAN_POINT ( 'NONE',  ( 8.637503779817164329, -3.056533381831490814, -6.534278797312786047 ) ) ;
#48361=CARTESIAN_POINT ( 'NONE',  ( 5.500000000000000000, 1.449999999999999956, 0.000000000000000000 ) ) ;
#48365=CARTESIAN_POINT ( 'NONE',  ( 7.905017292225999803, -2.916160783733999562, 6.437838678341997856 ) ) ;
#48366=VERTEX_POINT ( 'NONE', #33773 ) ;
#48369=CARTESIAN_POINT ( 'NONE',  ( 7.100000000000000533, -4.000000000000000000, -7.500000000000000000 ) ) ;
#48370=CARTESIAN_POINT ( 'NONE',  ( 9.533427734455999669, -2.564762519363000148, 6.150594768287000136 ) ) ;
#48373=CARTESIAN_POINT ( 'NONE',  ( 10.96080136920999948, -2.054580854576999904, 7.810082699133999995 ) ) ;
#48400=CARTESIAN_POINT ( 'NONE',  ( 9.834153701540001791, -5.173926576843999925, 8.813045240277000758 ) ) ;
#48405=CARTESIAN_POINT ( 'NONE',  ( 9.497293146791999874, -3.734278838175999482, 8.942129638874000364 ) ) ;
#48413=CARTESIAN_POINT ( 'NONE',  ( 11.15982711745999900, -5.578228817597000955, 8.067792329320999656 ) ) ;
#48430=ORIENTED_EDGE ( 'NONE', *, *, #14747, .F. ) ;
#48431=CARTESIAN_POINT ( 'NONE',  ( 9.321533510307233428, -4.073328655874168369, 9.239113755467350586 ) ) ;
#48440=DIRECTION ( 'NONE',  ( 1.000000000000000000, 0.000000000000000000, 0.000000000000000000 ) ) ;
#48443=CARTESIAN_POINT ( 'NONE',  ( 9.266298948830003823, -5.052976874734789625, -6.103419532891559030 ) ) ;
#48444=EDGE_CURVE ( 'NONE', #19018, #46752, #6979, .T. ) ;
#48452=CARTESIAN_POINT ( 'NONE',  ( 8.849379440379999906, -3.975070057433999438, 9.483761758588999058 ) ) ;
#48454=CARTESIAN_POINT ( 'NONE',  ( 7.866263695695000280, -4.690788429020999573, 6.339954069160000039 ) ) ;
#48457=CARTESIAN_POINT ( 'NONE',  ( 7.000000000000000000, 0.8000000000000000444, -3.149999999999999911 ) ) ;
#48461=CARTESIAN_POINT ( 'NONE',  ( 11.09999999999999964, -5.520231155209834206, 6.955941087530958633 ) ) ;
#48464=CARTESIAN_POINT ( 'NONE',  ( 7.930394353207000258, -3.164807285701999984, 9.104732190648000767 ) ) ;
#48467=CARTESIAN_POINT ( 'NONE',  ( 10.98768553379999879, -5.299329486732999861, 4.945210549701000602 ) ) ;
#48476=DIRECTION ( 'NONE',  ( 1.000000000000000000, 0.000000000000000000, 0.000000000000000000 ) ) ;
#48483=CARTESIAN_POINT ( 'NONE',  ( 8.449875654718679741, -2.260415483100814082, 7.498025105998177509 ) ) ;
#48492=CARTESIAN_POINT ( 'NONE',  ( 7.717918984469999799, -2.852331559125000027, 6.784354950350999225 ) ) ;
#48497=CARTESIAN_POINT ( 'NONE',  ( 8.893204545404998385, -3.399999999998999822, -6.188268997420999007 ) ) ;
#48506=CARTESIAN_POINT ( 'NONE',  ( 9.009297488802992859, -5.100000000000000533, 6.455145051482742424 ) ) ;
#48516=EDGE_LOOP ( 'NONE', ( #40118, #15313, #46977, #11502, #55324 ) ) ;
#48520=CARTESIAN_POINT ( 'NONE',  ( 5.700000000000000178, 0.000000000000000000, 0.000000000000000000 ) ) ;
#48524=CARTESIAN_POINT ( 'NONE',  ( 10.29094647910999782, -2.903513699412000104, -8.310923036409999298 ) ) ;
#48528=LINE ( 'NONE', #43284, #6540 ) ;
#48533=EDGE_CURVE ( 'NONE', #4646, #49898, #27913, .T. ) ;
#48538=VECTOR ( 'NONE', #49732, 1000.000000000000000 ) ;
#48546=FACE_OUTER_BOUND ( 'NONE', #7662, .T. ) ;
#48564=CARTESIAN_POINT ( 'NONE',  ( 10.57223537388000167, -4.020426196685999543, 8.920680607665000039 ) ) ;
#48565=CARTESIAN_POINT ( 'NONE',  ( 9.079730646793999327, -5.421531391267000011, 6.381128921159999301 ) ) ;
#48569=CARTESIAN_POINT ( 'NONE',  ( 10.33453064679000200, -3.295701412239999684, -6.149875347297999895 ) ) ;
#48570=CARTESIAN_POINT ( 'NONE',  ( 7.898140067141143028, -2.604783987062581296, 8.538297895486305578 ) ) ;
#48571=CARTESIAN_POINT ( 'NONE',  ( 10.34020413671000149, -4.202027362542999356, 9.459588031742001135 ) ) ;
#48572=CARTESIAN_POINT ( 'NONE',  ( 10.04762827527057212, -4.043475410182937324, 8.964136762659371982 ) ) ;
#48578=MECHANICAL_DESIGN_GEOMETRIC_PRESENTATION_REPRESENTATION('',(#45245),#25117);
#48588=CARTESIAN_POINT ( 'NONE',  ( 8.753441940380000119, -2.876278577719999952, 6.568889245344999850 ) ) ;
#48597=CARTESIAN_POINT ( 'NONE',  ( 10.69031285273999821, -5.903020122789000013, 7.830708506196000229 ) ) ;
#48617=ORIENTED_EDGE ( 'NONE', *, *, #34586, .T. ) ;
#48631=ADVANCED_FACE ( 'NONE', ( #8570 ), #7191, .F. ) ;
#48635=B_SPLINE_CURVE_WITH_KNOTS ( 'NONE', 3,
 ( #57191, #9638, #29623, #66993, #14896 ),
 .UNSPECIFIED., .F., .F.,
 ( 4, 1, 4 ),
 ( 0.000000000000000000, 0.5000000000000000000, 1.000000000000000000 ),
 .UNSPECIFIED. ) ;
#48641=AXIS2_PLACEMENT_3D ( 'NONE', #1503, #17590, #5366 ) ;
#48656=CARTESIAN_POINT ( 'NONE',  ( 10.24394435321000074, -3.220344030624999743, -6.005416930865999703 ) ) ;
#48659=LINE ( 'NONE', #22078, #65431 ) ;
#48662=ORIENTED_EDGE ( 'NONE', *, *, #33730, .F. ) ;
#48677=CARTESIAN_POINT ( 'NONE',  ( 10.14584566409999944, -5.370505908760000224, -6.826219946961000318 ) ) ;
#48681=ORIENTED_EDGE ( 'NONE', *, *, #3274, .F. ) ;
#48693=CARTESIAN_POINT ( 'NONE',  ( 11.29621718459000057, -3.561654022787999807, 6.266039799355000106 ) ) ;
#48697=EDGE_CURVE ( 'NONE', #28877, #8998, #4342, .T. ) ;
#48705=CARTESIAN_POINT ( 'NONE',  ( 10.62924380535000068, -3.609488729914999805, -5.855142811286000004 ) ) ;
#48711=LINE ( 'NONE', #59538, #18510 ) ;
#48715=EDGE_CURVE ( 'NONE', #49491, #27465, #21210, .T. ) ;
#48724=CARTESIAN_POINT ( 'NONE',  ( 10.71256247620999957, -5.951803124515000043, 7.233045248871000865 ) ) ;
#48727=CARTESIAN_POINT ( 'NONE',  ( 11.25041341105000114, -5.730771985297000271, 8.122672103119001008 ) ) ;
#48728=CARTESIAN_POINT ( 'NONE',  ( 10.90378878155999942, -2.900209876291999667, -5.134763467624999578 ) ) ;
#48732=B_SPLINE_CURVE_WITH_KNOTS ( 'NONE', 3,
 ( #58192, #53635, #5046, #5730 ),
 .UNSPECIFIED., .F., .F.,
 ( 4, 4 ),
 ( 0.000000000000000000, 0.1254132184345819190 ),
 .UNSPECIFIED. ) ;
#48735=CARTESIAN_POINT ( 'NONE',  ( 5.500000000000000000, -7.849276784099999367E-14, -1.865174681369999824E-14 ) ) ;
#48738=CARTESIAN_POINT ( 'NONE',  ( 6.877770285292999830, -9.263688577134999491, -5.299267108162999840 ) ) ;
#48740=DIRECTION ( 'NONE',  ( -1.000000000000000000, 0.000000000000000000, 0.000000000000000000 ) ) ;
#48742=CARTESIAN_POINT ( 'NONE',  ( 5.000000000000000000, 0.000000000000000000, 0.000000000000000000 ) ) ;
#48761=CARTESIAN_POINT ( 'NONE',  ( 10.62698276521000196, -3.142914536759000121, 8.668455626664998803 ) ) ;
#48777=EDGE_CURVE ( 'NONE', #61687, #27541, #17887, .T. ) ;
#48778=CARTESIAN_POINT ( 'NONE',  ( 9.327269112000164952, -3.948692165092429374, 9.238904779716392568 ) ) ;
#48787=CARTESIAN_POINT ( 'NONE',  ( 10.96080136920999948, -2.054580854576999904, 7.810082699133999995 ) ) ;
#48795=CARTESIAN_POINT ( 'NONE',  ( 9.385788300200999856, -4.980873770300999759, 6.433336655958999728 ) ) ;
#48797=CARTESIAN_POINT ( 'NONE',  ( 7.897956853208000005, -3.608524635952000459, 5.913372239166000632 ) ) ;
#48802=EDGE_CURVE ( 'NONE', #41119, #67742, #17955, .T. ) ;
#48812=DIRECTION ( 'NONE',  ( -2.017751170287999915E-09, -7.180968446191999491E-11, 1.000000000000000000 ) ) ;
#48829=CARTESIAN_POINT ( 'NONE',  ( 8.442993682891730245, -2.265460329437196219, 7.647905870472889944 ) ) ;
#48842=CARTESIAN_POINT ( 'NONE',  ( 10.83253786428999987, -2.899999999999999911, 6.571291218949999902 ) ) ;
#48843=B_SPLINE_CURVE_WITH_KNOTS ( 'NONE', 3,
 ( #26969, #10195, #20685, #21031 ),
 .UNSPECIFIED., .F., .F.,
 ( 4, 4 ),
 ( 0.000000000000000000, 1.000000000000000000 ),
 .UNSPECIFIED. ) ;
#48844=AXIS2_PLACEMENT_3D ( 'NONE', #59422, #32864, #47309 ) ;
#48846=CARTESIAN_POINT ( 'NONE',  ( 8.919816864363674824, -2.358207424585543777, 8.150886335909103053 ) ) ;
#48855=ORIENTED_EDGE ( 'NONE', *, *, #43001, .F. ) ;
#48866=EDGE_CURVE ( 'NONE', #1541, #46332, #2031, .T. ) ;
#48867=ORIENTED_EDGE ( 'NONE', *, *, #15179, .T. ) ;
#48872=CARTESIAN_POINT ( 'NONE',  ( 10.70780617489000086, -5.157482071823000780, -6.267811103859000532 ) ) ;
#48883=CARTESIAN_POINT ( 'NONE',  ( 11.09999999999999964, -2.700000001949000250, -5.146415525425999782 ) ) ;
#48890=CARTESIAN_POINT ( 'NONE',  ( 5.700000000378000031, -0.2999999996220999443, 3.150000004979999879 ) ) ;
#48909=CARTESIAN_POINT ( 'NONE',  ( 9.903944471677000649, -5.205019707614999547, 6.747219600580999455 ) ) ;
#48910=CARTESIAN_POINT ( 'NONE',  ( 8.320870559624999885, -3.894643656844000379, 6.044452984962999764 ) ) ;
#48914=CARTESIAN_POINT ( 'NONE',  ( 11.17788601987000163, -2.412142864687000010, -7.075602314719000141 ) ) ;
#48915=CARTESIAN_POINT ( 'NONE',  ( 7.645471844114070770, -5.358564433078305100, 6.414118424940338237 ) ) ;
#48934=ORIENTED_EDGE ( 'NONE', *, *, #10025, .T. ) ;
#48935=CARTESIAN_POINT ( 'NONE',  ( 9.331129440379999807, -4.141908960411000429, 6.047561724438000219 ) ) ;
#48938=CARTESIAN_POINT ( 'NONE',  ( 10.12284001496798780, -2.396628744330400629, -6.794529262851803253 ) ) ;
#48947=DIRECTION ( 'NONE',  ( -0.000000000000000000, 1.000000000000000000, 0.000000000000000000 ) ) ;
#48965=ADVANCED_FACE ( 'NONE', ( #39972 ), #14085, .F. ) ;
#48978=FACE_OUTER_BOUND ( 'NONE', #16317, .T. ) ;
#48987=CARTESIAN_POINT ( 'NONE',  ( 8.688612068284298218, -2.650857310365693831, 7.263856826349748275 ) ) ;
#48999=CARTESIAN_POINT ( 'NONE',  ( 11.26847231345999845, -2.565616654150999931, -7.116622328138999976 ) ) ;
#49002=CARTESIAN_POINT ( 'NONE',  ( 9.881157842586999251, -5.290169207169999943, -8.858081286661999343 ) ) ;
#49010=ORIENTED_EDGE ( 'NONE', *, *, #44922, .F. ) ;
#49022=CARTESIAN_POINT ( 'NONE',  ( 9.766127544684000128, -4.735430008785999512, -8.791396910319001279 ) ) ;
#49023=LINE ( 'NONE', #49360, #17300 ) ;
#49047=CARTESIAN_POINT ( 'NONE',  ( 10.01276877312999858, -3.440626575163999945, -9.267592337498999910 ) ) ;
#49049=CARTESIAN_POINT ( 'NONE',  ( 6.953052440528999512, -9.233022020364000326, -5.200634764108000851 ) ) ;
#49050=CARTESIAN_POINT ( 'NONE',  ( 10.90000000000000036, -5.100000000000000533, -6.436740704805999691 ) ) ;
#49061=ORIENTED_EDGE ( 'NONE', *, *, #59962, .T. ) ;
#49063=CARTESIAN_POINT ( 'NONE',  ( 10.40226385995999969, -2.765692573780999641, 9.035345396600000356 ) ) ;
#49066=CARTESIAN_POINT ( 'NONE',  ( 9.724613486786999772, -2.928302463146000179, 8.718481221599999387 ) ) ;
#49067=CARTESIAN_POINT ( 'NONE',  ( 9.718562776053557783, -5.699238565681682189, 7.915948022123772354 ) ) ;
#49080=CARTESIAN_POINT ( 'NONE',  ( 7.683561622480320707, -2.820687929279365846, 8.178835501142698305 ) ) ;
#49086=CARTESIAN_POINT ( 'NONE',  ( 7.933148997457998952, -5.167567567567999731, 6.822293592207000934 ) ) ;
#49089=ORIENTED_EDGE ( 'NONE', *, *, #55802, .T. ) ;
#49092=EDGE_LOOP ( 'NONE', ( #45729, #13141, #36890, #43676, #4018 ) ) ;
#49096=FACE_OUTER_BOUND ( 'NONE', #36125, .T. ) ;
#49100=CARTESIAN_POINT ( 'NONE',  ( 10.99166666666866909, -4.098468854244173620, 8.958105619229149497 ) ) ;
#49101=ORIENTED_EDGE ( 'NONE', *, *, #54172, .T. ) ;
#49105=EDGE_CURVE ( 'NONE', #26424, #873, #47271, .T. ) ;
#49112=CARTESIAN_POINT ( 'NONE',  ( 8.474485200571999499, -5.100000000000000533, 6.560614371780999043 ) ) ;
#49124=CARTESIAN_POINT ( 'NONE',  ( 10.40226385995999969, -2.765692573780999641, 9.035345396600000356 ) ) ;
#49129=CARTESIAN_POINT ( 'NONE',  ( 11.09999999999999964, -1.406666666667000021, -10.45580168561000001 ) ) ;
#49135=CARTESIAN_POINT ( 'NONE',  ( 7.000000000000000000, -0.2897247358851999799, 3.000000000000000000 ) ) ;
#49137=VECTOR ( 'NONE', #63881, 1000.000000000000000 ) ;
#49140=FACE_OUTER_BOUND ( 'NONE', #65168, .T. ) ;
#49146=EDGE_LOOP ( 'NONE', ( #4485, #50759, #37149, #357 ) ) ;
#49160=CARTESIAN_POINT ( 'NONE',  ( 7.142264750549939478, -3.320997592312212365, 8.680193631428091194 ) ) ;
#49167=CARTESIAN_POINT ( 'NONE',  ( 8.520843751322205506, -2.921428602731328539, 6.124930925903640855 ) ) ;
#49173=CARTESIAN_POINT ( 'NONE',  ( 10.07101719722999889, -4.042170815906999337, 8.920201479886998186 ) ) ;
#49174=ORIENTED_EDGE ( 'NONE', *, *, #49735, .T. ) ;
#49183=CARTESIAN_POINT ( 'NONE',  ( 9.020964430773000586, -2.907392932634000005, 6.146188468825999784 ) ) ;
#49189=AXIS2_PLACEMENT_3D ( 'NONE', #41249, #31117, #52420 ) ;
#49199=CARTESIAN_POINT ( 'NONE',  ( 7.100000000000000533, -2.649999999999999911, -7.500000000000000000 ) ) ;
#49209=CARTESIAN_POINT ( 'NONE',  ( 10.57793869653000129, -4.393380534095000733, -6.024358525186999991 ) ) ;
#49213=VERTEX_POINT ( 'NONE', #16814 ) ;
#49226=ORIENTED_EDGE ( 'NONE', *, *, #43260, .F. ) ;
#49227=CARTESIAN_POINT ( 'NONE',  ( 8.656816940379998826, -5.329429281359999493, 6.027400270608000099 ) ) ;
#49243=CARTESIAN_POINT ( 'NONE',  ( 10.12670810574000058, -3.117521507207000386, 8.613544937223998943 ) ) ;
#49250=CARTESIAN_POINT ( 'NONE',  ( 11.20536814679000059, -2.688541832249000230, -8.273932507170000505 ) ) ;
#49251=CARTESIAN_POINT ( 'NONE',  ( 7.762804160121919317, -5.211073624054318287, 8.750271362508501127 ) ) ;
#49252=CARTESIAN_POINT ( 'NONE',  ( 9.215289122285998502, -4.861979632688999686, 8.938813901364000003 ) ) ;
#49267=CARTESIAN_POINT ( 'NONE',  ( 27.64127793187000037, -4.599999999999999645, 8.890528821780000257 ) ) ;
#49271=VERTEX_POINT ( 'NONE', #65045 ) ;
#49272=CARTESIAN_POINT ( 'NONE',  ( 9.953700334934390881, -4.258430994261761526, -9.268957274791640444 ) ) ;
#49275=CARTESIAN_POINT ( 'NONE',  ( 10.11549555961999936, -2.489199523559999960, -6.434642413229999747 ) ) ;
#49278=CARTESIAN_POINT ( 'NONE',  ( 10.52324012719000024, -3.325647021086999722, 5.689999163383999026 ) ) ;
#49300=B_SPLINE_CURVE_WITH_KNOTS ( 'NONE', 3,
 ( #43348, #64649, #15402, #58046 ),
 .UNSPECIFIED., .F., .F.,
 ( 4, 4 ),
 ( 0.000000000000000000, 0.1254120260046326096 ),
 .UNSPECIFIED. ) ;
#49316=ORIENTED_EDGE ( 'NONE', *, *, #24784, .F. ) ;
#49329=FACE_OUTER_BOUND ( 'NONE', #16064, .T. ) ;
#49330=CIRCLE ( 'NONE', #67197, 10.55000000000000426 ) ;
#49340=CARTESIAN_POINT ( 'NONE',  ( 9.991527686541001430, -4.805948463426999773, -8.932428271061001013 ) ) ;
#49341=CARTESIAN_POINT ( 'NONE',  ( 8.893204545428000429, -4.599999999999999645, -6.188268997401999982 ) ) ;
#49343=DIRECTION ( 'NONE',  ( 0.000000000000000000, -1.000000000000000000, 0.000000000000000000 ) ) ;
#49353=CARTESIAN_POINT ( 'NONE',  ( 10.31905590579000176, -2.899999999999999911, -6.571291218949999902 ) ) ;
#49358=CARTESIAN_POINT ( 'NONE',  ( 10.86493091395000121, -4.678465004315999209, -9.048463592221999363 ) ) ;
#49360=CARTESIAN_POINT ( 'NONE',  ( 11.10000000044000146, -0.5000000004447999746, 9.662944680343001025 ) ) ;
#49363=VERTEX_POINT ( 'NONE', #51058 ) ;
#49367=ORIENTED_EDGE ( 'NONE', *, *, #23853, .T. ) ;
#49382=CARTESIAN_POINT ( 'NONE',  ( 11.09999999999999964, -4.000000000000000000, 7.500000000000000000 ) ) ;
#49384=CARTESIAN_POINT ( 'NONE',  ( 10.47211906628000122, -2.640759929160000130, -8.505246563374999624 ) ) ;
#49387=CARTESIAN_POINT ( 'NONE',  ( 7.883148997456999929, -5.167567567567999731, 6.822293592207000934 ) ) ;
#49388=CARTESIAN_POINT ( 'NONE',  ( 8.296466976089000411, -2.897909218876999926, 6.617342437405000055 ) ) ;
#49402=CARTESIAN_POINT ( 'NONE',  ( 9.629020610622001541, -5.794331084664000819, 7.414872097535999629 ) ) ;
#49405=CARTESIAN_POINT ( 'NONE',  ( 10.25462442569999943, -2.860634389522000109, 6.604605425112000994 ) ) ;
#49414=CARTESIAN_POINT ( 'NONE',  ( 9.573148997458000409, -5.167567567567999731, -6.822293592207000934 ) ) ;
#49429=VERTEX_POINT ( 'NONE', #66790 ) ;
#49433=CARTESIAN_POINT ( 'NONE',  ( 10.47094409420000005, -5.100000000000000533, 6.571291218949999902 ) ) ;
#49437=CARTESIAN_POINT ( 'NONE',  ( 11.09999999999999964, -2.274006712557999688, -7.281956340829000673 ) ) ;
#49440=CARTESIAN_POINT ( 'NONE',  ( 9.323795176894432046, -5.066048497541554063, -6.242748793373607441 ) ) ;
#49448=ORIENTED_EDGE ( 'NONE', *, *, #11731, .T. ) ;
#49470=ORIENTED_EDGE ( 'NONE', *, *, #39979, .F. ) ;
#49477=CARTESIAN_POINT ( 'NONE',  ( 10.62698276521000196, -3.142914536759000121, 8.668455626664998803 ) ) ;
#49478=CARTESIAN_POINT ( 'NONE',  ( 9.228231092913778966, -5.653336912713888829, 8.124910183455536838 ) ) ;
#49479=CARTESIAN_POINT ( 'NONE',  ( 8.898558059623999483, -5.146736128384000075, 6.597417125647000447 ) ) ;
#49484=CARTESIAN_POINT ( 'NONE',  ( 8.974845122786007323, -5.117933181718998803, -6.719699903140006647 ) ) ;
#49489=CARTESIAN_POINT ( 'NONE',  ( 8.379867906070000316, -2.923743482135000349, 6.439439799216000182 ) ) ;
#49491=VERTEX_POINT ( 'NONE', #29061 ) ;
#49492=CARTESIAN_POINT ( 'NONE',  ( 9.187745559622999991, -5.964711531933999389, 7.776478361891000723 ) ) ;
#49516=CARTESIAN_POINT ( 'NONE',  ( 9.681180837610000367, -2.612237299844000216, 7.804680206899999639 ) ) ;
#49521=ORIENTED_EDGE ( 'NONE', *, *, #25790, .F. ) ;
#49528=ORIENTED_EDGE ( 'NONE', *, *, #58253, .F. ) ;
#49547=EDGE_LOOP ( 'NONE', ( #60357, #58658, #60113, #58160 ) ) ;
#49552=CARTESIAN_POINT ( 'NONE',  ( 10.42081395746000005, -2.488448635474999726, -7.717895569088000229 ) ) ;
#49564=CARTESIAN_POINT ( 'NONE',  ( 5.500000000000000000, -1.300000000000000044, -9.662944685757000940 ) ) ;
#49573=VERTEX_POINT ( 'NONE', #27853 ) ;
#49574=CARTESIAN_POINT ( 'NONE',  ( 8.822980646795000936, -2.678334737187000325, 8.735278777293000729 ) ) ;
#49575=CARTESIAN_POINT ( 'NONE',  ( 9.529144223516999190, -2.330665094450000030, -8.349943402163999551 ) ) ;
#49578=CARTESIAN_POINT ( 'NONE',  ( 11.09999999999999964, -2.685305999535000154, 6.664030027596000494 ) ) ;
#49592=CARTESIAN_POINT ( 'NONE',  ( 10.44675369521999997, -2.885048926231000177, 8.863479194807000638 ) ) ;
#49595=VERTEX_POINT ( 'NONE', #23466 ) ;
#49598=CARTESIAN_POINT ( 'NONE',  ( 10.28180685320999999, -3.991526694881000203, -5.814304247846999729 ) ) ;
#49599=CARTESIAN_POINT ( 'NONE',  ( 8.091091889490169109, -4.367519155558725608, 5.800091099343307022 ) ) ;
#49600=CARTESIAN_POINT ( 'NONE',  ( 11.20904026220999938, -5.937811873294999820, 7.147336919140999001 ) ) ;
#49615=CARTESIAN_POINT ( 'NONE',  ( 8.832537864289999874, -2.899999999999999911, 6.571291218949999902 ) ) ;
#49638=CARTESIAN_POINT ( 'NONE',  ( 7.933148997457998952, -5.167567567567999731, 6.822293592207000934 ) ) ;
#49654=ORIENTED_EDGE ( 'NONE', *, *, #43586, .F. ) ;
#49668=VECTOR ( 'NONE', #28887, 999.9999999999998863 ) ;
#49682=LINE ( 'NONE', #6679, #60917 ) ;
#49693=CARTESIAN_POINT ( 'NONE',  ( 10.62256935321000029, -2.471463903746000224, -8.210787855397999380 ) ) ;
#49697=ORIENTED_EDGE ( 'NONE', *, *, #21997, .F. ) ;
#49706=EDGE_CURVE ( 'NONE', #3171, #43113, #28373, .T. ) ;
#49713=CARTESIAN_POINT ( 'NONE',  ( 10.15786958814999963, -4.213496663054999480, -5.822956951053000374 ) ) ;
#49715=VECTOR ( 'NONE', #16616, 1000.000000000000000 ) ;
#49720=CARTESIAN_POINT ( 'NONE',  ( 11.00127285756000006, -5.155741062898000493, 5.106993030795000443 ) ) ;
#49725=CARTESIAN_POINT ( 'NONE',  ( 10.16829915263999951, -4.567213659083999566, 5.832528837986999726 ) ) ;
#49726=ORIENTED_EDGE ( 'NONE', *, *, #54379, .T. ) ;
#49729=ORIENTED_EDGE ( 'NONE', *, *, #54528, .F. ) ;
#49731=EDGE_CURVE ( 'NONE', #42529, #60343, #53657, .T. ) ;
#49732=DIRECTION ( 'NONE',  ( -0.7071067811864980568, 0.7071067811865969777, 6.440255933040979921E-09 ) ) ;
#49735=EDGE_CURVE ( 'NONE', #2498, #51230, #55270, .T. ) ;
#49737=CIRCLE ( 'NONE', #66498, 0.2999999999999999889 ) ;
#49739=CARTESIAN_POINT ( 'NONE',  ( 10.52342417510000061, -3.209670667763000029, -9.177087527572998837 ) ) ;
#49740=CARTESIAN_POINT ( 'NONE',  ( 9.550978115722108086, -5.350351920099831737, -7.263395478037801389 ) ) ;
#49741=CARTESIAN_POINT ( 'NONE',  ( 8.256788585354000176, -2.896778558933000181, 6.628796229400999884 ) ) ;
#49751=EDGE_LOOP ( 'NONE', ( #57274, #11413, #55046, #52740 ) ) ;
#49754=FACE_OUTER_BOUND ( 'NONE', #13059, .T. ) ;
#49757=CARTESIAN_POINT ( 'NONE',  ( 9.385788300200999856, -4.980873770300999759, 6.433336655958999728 ) ) ;
#49766=B_SPLINE_SURFACE_WITH_KNOTS ( 'NONE', 3, 3, ( 
 ( #10789, #5544, #51218, #23002, #9238, #56811, #60074, #30579, #60417, #28255, #49575, #14164, #8907, #33508, #62387, #45971, #30248, #24300, #14504 ),
 ( #54824, #45638, #24649, #57140, #33853, #51892, #6923, #8567, #35823, #22652, #43997, #67280, #12178, #29913, #24986, #65304, #17419, #51551, #19398 ),
 ( #28612, #2037, #38745, #3649, #44351, #35489, #40719, #55167, #17774, #1685, #46320, #13820, #67620, #62047, #19745, #61703, #41068, #66941, #19052 ),
 ( #65650, #39092, #12522, #7272, #49926, #40379, #35149, #56464, #3314, #20425, #52933, #3990, #58514, #37532, #9934, #14842, #10969, #42102, #5028 ) ),
 .UNSPECIFIED., .F., .F., .F.,
 ( 4, 4 ),
 ( 4, 1, 1, 1, 1, 1, 1, 1, 1, 1, 1, 1, 1, 1, 1, 1, 4 ),
 ( -0.1039086239011999951, 1.103908623900999864 ),
 ( -0.008849010032007000384, 0.01991027257200999809, 0.04866955517603999831, 0.07742883778006000306, 0.1061881203840999988, 0.1349474029881000126, 0.1637066855920999986, 0.1924659681960999846, 0.2212252508002000018, 0.2499845334042000156, 0.2787438160081999738, 0.3075030986121999876, 0.3362623812162000014, 0.3650216638202999908, 0.3937809464243000046, 0.4225402290282999629, 0.4512995116322999767 ),
 .UNSPECIFIED. ) ;
#49769=CARTESIAN_POINT ( 'NONE',  ( 0.000000000000000000, -5.100000000000000533, 7.500000000000000000 ) ) ;
#49783=ORIENTED_EDGE ( 'NONE', *, *, #7426, .T. ) ;
#49785=DIRECTION ( 'NONE',  ( -1.000000000000000000, 0.000000000000000000, 0.000000000000000000 ) ) ;
#49789=CARTESIAN_POINT ( 'NONE',  ( 8.995183059623999000, -2.707994276285999646, 5.994456121676999594 ) ) ;
#49798=CARTESIAN_POINT ( 'NONE',  ( 10.90000000000000036, -5.283926297003000094, 7.082827057608000132 ) ) ;
#49800=CARTESIAN_POINT ( 'NONE',  ( 9.385788300200999856, -4.980873770300999759, 6.433336655958999728 ) ) ;
#49801=DIRECTION ( 'NONE',  ( 1.000000000000000000, 0.000000000000000000, 0.000000000000000000 ) ) ;
#49812=CARTESIAN_POINT ( 'NONE',  ( 9.348645089171384370, -3.479920518481517178, 9.160150987731649153 ) ) ;
#49816=CARTESIAN_POINT ( 'NONE',  ( 11.13359725006000112, -5.335216433401000380, -5.114389220295000982 ) ) ;
#49819=CARTESIAN_POINT ( 'NONE',  ( 10.52638330645999964, -2.451090818816000105, 6.282756943804999494 ) ) ;
#49821=CIRCLE ( 'NONE', #25261, 1.350000000000000089 ) ;
#49828=CARTESIAN_POINT ( 'NONE',  ( 10.93728138146000006, -5.425439422033999648, 7.240583766112999697 ) ) ;
#49830=CARTESIAN_POINT ( 'NONE',  ( 9.160311019873999427, -4.122021308488999836, 9.013573548576999883 ) ) ;
#49833=CARTESIAN_POINT ( 'NONE',  ( 10.96256888877000080, -5.431976784349000553, 4.905455483671000039 ) ) ;
#49835=VECTOR ( 'NONE', #1796, 1000.000000000000000 ) ;
#49840=CARTESIAN_POINT ( 'NONE',  ( 11.09999999999999964, -5.435899401150079413, 6.701932011082668339 ) ) ;
#49841=ADVANCED_FACE ( 'NONE', ( #34310 ), #3175, .F. ) ;
#49844=CARTESIAN_POINT ( 'NONE',  ( 8.995183059623999000, -2.707994276285999646, 5.994456121676999594 ) ) ;
#49847=CARTESIAN_POINT ( 'NONE',  ( 7.550000000000000711, -4.000000000000000000, 8.849999999999999645 ) ) ;
#49858=ORIENTED_EDGE ( 'NONE', *, *, #63158, .T. ) ;
#49861=CARTESIAN_POINT ( 'NONE',  ( 8.572516478978494447, -3.946509990130368184, 5.760726263960903815 ) ) ;
#49868=CARTESIAN_POINT ( 'NONE',  ( 9.489405368643582861, -4.927979915958162316, 8.480323300091150429 ) ) ;
#49872=ORIENTED_EDGE ( 'NONE', *, *, #61002, .F. ) ;
#49882=CARTESIAN_POINT ( 'NONE',  ( 7.100000000000000533, -4.000000000000000000, 7.500000000000000000 ) ) ;
#49890=CARTESIAN_POINT ( 'NONE',  ( 10.96685777392725036, -2.822345360332068509, -6.668352631380622064 ) ) ;
#49893=CARTESIAN_POINT ( 'NONE',  ( 6.877497653516999598, -9.263786119211999903, 5.299649687518000363 ) ) ;
#49898=VERTEX_POINT ( 'NONE', #9659 ) ;
#49903=CARTESIAN_POINT ( 'NONE',  ( 10.18512684885999953, -5.526147823900999789, -7.556025229989000280 ) ) ;
#49908=CARTESIAN_POINT ( 'NONE',  ( 11.09999999999999964, -2.700469802787999640, -5.124965750789000296 ) ) ;
#49911=CARTESIAN_POINT ( 'NONE',  ( 11.00000000066999917, -1.300000000000000044, 9.662944685757000940 ) ) ;
#49925=CARTESIAN_POINT ( 'NONE',  ( 7.218293146793000048, -4.773080213113000347, 8.927399220053999329 ) ) ;
#49926=CARTESIAN_POINT ( 'NONE',  ( 10.06491331857999860, -5.318469253323000245, -7.099528416287999910 ) ) ;
#49931=DIRECTION ( 'NONE',  ( 0.000000000000000000, 0.000000000000000000, -1.000000000000000000 ) ) ;
#49938=VECTOR ( 'NONE', #6165, 1000.000000000000000 ) ;
#49941=CARTESIAN_POINT ( 'NONE',  ( 9.778462793022999477, -5.743713977826000239, 7.748300060190000060 ) ) ;
#49946=CARTESIAN_POINT ( 'NONE',  ( 7.934858580180682353, -2.291129595918548922, 7.825900736742252839 ) ) ;
#49947=CARTESIAN_POINT ( 'NONE',  ( 10.22109127278999807, -2.983266195621000261, 8.764707262515999631 ) ) ;
#49948=CARTESIAN_POINT ( 'NONE',  ( 10.16967105008495587, -2.650360704944366042, 7.590422644555561149 ) ) ;
#49962=EDGE_CURVE ( 'NONE', #62127, #2041, #34223, .T. ) ;
#49966=CARTESIAN_POINT ( 'NONE',  ( 7.545269353206999874, -2.302293129340000188, 6.875167727519000849 ) ) ;
#49968=ORIENTED_EDGE ( 'NONE', *, *, #65652, .F. ) ;
#49979=AXIS2_PLACEMENT_3D ( 'NONE', #10955, #21105, #58847 ) ;
#49981=B_SPLINE_CURVE_WITH_KNOTS ( 'NONE', 3,
 ( #38772, #49948, #54501, #12546, #48572, #64972, #28281, #39116, #66015 ),
 .UNSPECIFIED., .F., .F.,
 ( 4, 1, 1, 1, 1, 1, 4 ),
 ( 0.1253905405517105054, 0.1733119344633363701, 0.3402003772241184443, 0.5070888199843091027, 0.6739772627450910658, 0.8408657055052815021, 0.8746295857519847949 ),
 .UNSPECIFIED. ) ;
#49986=AXIS2_PLACEMENT_3D ( 'NONE', #54204, #17146, #10871 ) ;
#50009=ORIENTED_EDGE ( 'NONE', *, *, #62888, .T. ) ;
#50017=B_SPLINE_CURVE_WITH_KNOTS ( 'NONE', 3,
 ( #7335, #33572, #59097, #38464, #65011 ),
 .UNSPECIFIED., .F., .F.,
 ( 4, 1, 4 ),
 ( 0.000000000000000000, 0.4040625160519999981, 1.000000000000000000 ),
 .UNSPECIFIED. ) ;
#50028=CARTESIAN_POINT ( 'NONE',  ( 9.422954534637428381, -5.349869571284899372, 7.471026763531456893 ) ) ;
#50034=CARTESIAN_POINT ( 'NONE',  ( 7.448092524957871774, -2.260623559829979090, 7.520946136199704313 ) ) ;
#50042=CARTESIAN_POINT ( 'NONE',  ( 9.525000000000000355, -4.417172942406000224, 8.783926296998000538 ) ) ;
#50044=CARTESIAN_POINT ( 'NONE',  ( 10.99245660749487463, -6.449695542863823405, 5.237054987098043846 ) ) ;
#50061=CARTESIAN_POINT ( 'NONE',  ( 10.36409408021999923, -3.399999909169000301, -4.954046131279000065 ) ) ;
#50065=CARTESIAN_POINT ( 'NONE',  ( 11.17811058788999823, -2.762459764047000110, -6.187206491620000470 ) ) ;
#50072=CARTESIAN_POINT ( 'NONE',  ( 10.95931585633000083, -5.066484979568000035, 5.182226135408999568 ) ) ;
#50077=CARTESIAN_POINT ( 'NONE',  ( 10.03612181215999932, -3.011786236723999810, 8.746965724352000038 ) ) ;
#50085=CONICAL_SURFACE ( 'NONE', #54517, 0.3062142749367001149, 0.7853981633972997312 ) ;
#50094=CARTESIAN_POINT ( 'NONE',  ( 9.790745838555999114, -4.301175052434000001, -8.935144319903001175 ) ) ;
#50100=CARTESIAN_POINT ( 'NONE',  ( 10.53455565919999870, -3.019620544914000337, 5.071252824073000376 ) ) ;
#50105=CARTESIAN_POINT ( 'NONE',  ( 11.05639424537999993, -5.030223832177999732, 6.028291574375000295 ) ) ;
#50110=CARTESIAN_POINT ( 'NONE',  ( 10.53138988903999973, -5.607755226963999640, 7.280101849877000042 ) ) ;
#50111=CARTESIAN_POINT ( 'NONE',  ( 9.637090959179923644, -5.238013552912343940, 6.265105236445105419 ) ) ;
#50118=FACE_OUTER_BOUND ( 'NONE', #37928, .T. ) ;
#50119=FACE_OUTER_BOUND ( 'NONE', #61719, .T. ) ;
#50121=CARTESIAN_POINT ( 'NONE',  ( 7.773264358664000007, -2.859518314699000197, 6.768377407145999669 ) ) ;
#50123=CARTESIAN_POINT ( 'NONE',  ( 9.174722005181999762, -5.536248950452999473, -7.355084988757000453 ) ) ;
#50130=ADVANCED_FACE ( 'NONE', ( #21596 ), #21261, .T. ) ;
#50140=CARTESIAN_POINT ( 'NONE',  ( 11.09999999999999964, -4.000000000000000000, -7.500000000000000000 ) ) ;
#50151=EDGE_LOOP ( 'NONE', ( #24152, #20565, #4058, #649, #3216, #18896 ) ) ;
#50162=CARTESIAN_POINT ( 'NONE',  ( 9.354106685273835708, -3.367328683712668802, 9.120272287704549896 ) ) ;
#50167=CARTESIAN_POINT ( 'NONE',  ( 10.95345670791000003, -5.155055429684999524, -5.171522713314000264 ) ) ;
#50170=CARTESIAN_POINT ( 'NONE',  ( 10.09196524370999981, -3.841385669346000231, 5.536421174581999338 ) ) ;
#50174=ORIENTED_EDGE ( 'NONE', *, *, #22958, .T. ) ;
#50180=CARTESIAN_POINT ( 'NONE',  ( 7.293870559621999483, -3.416208448044999901, 6.162501393933999871 ) ) ;
#50181=LINE ( 'NONE', #65557, #22614 ) ;
#50184=DIRECTION ( 'NONE',  ( 0.8480635683784220058, 0.000000000000000000, -0.5298945026977139872 ) ) ;
#50191=B_SPLINE_SURFACE_WITH_KNOTS ( 'NONE', 3, 3, ( 
 ( #47538, #63939, #43321, #58703, #64625, #59734, #27583, #65318, #48909, #17434, #16733, #22325, #49243, #1017, #64964, #37381, #16050, #42971, #6241, #38763, #48564, #11487, #59051, #53801, #21980, #5898, #11835, #38062, #42629, #59387, #43667, #10806, #32827, #32150, #54143 ),
 ( #26901, #17078, #64278, #1353, #32488, #22670, #48213, #33175, #44014, #26556, #38410, #53466, #5559, #54492, #6593, #27934, #10460, #53118, #5220, #31802, #47883, #69187, #21299, #320, #21636, #16395, #37722, #11153, #27240, #668, #55879, #1700, #18823, #23019, #40149 ),
 ( #39453, #29671, #34216, #29318, #56218, #2052, #66008, #61124, #60431, #49941, #33522, #34902, #28272, #13582, #13241, #28980, #55536, #60772, #18131, #45390, #7633, #49592, #23371, #50287, #44711, #2732, #12887, #2388, #23712, #24057, #7985, #45733, #50974, #45047, #33868 ),
 ( #39800, #7288, #28628, #8328, #17789, #66355, #39107, #12539, #54841, #60088, #3070, #18474, #34566, #44367, #66701, #50631, #12194, #61463, #24403, #67042, #6937, #65666, #19152, #55183, #68403, #20526, #51652, #4780, #68065, #20181, #57937, #8668, #68754, #14263, #19502 ) ),
 .UNSPECIFIED., .F., .F., .F.,
 ( 4, 4 ),
 ( 4, 1, 1, 1, 1, 1, 1, 1, 1, 1, 1, 1, 1, 1, 1, 1, 1, 1, 1, 1, 1, 1, 1, 1, 1, 1, 1, 1, 1, 1, 1, 1, 4 ),
 ( -0.1039086239011999951, 1.103908623900999864 ),
 ( -0.01735257130020999988, 0.01084535706264999969, 0.03904328542550000031, 0.06724121378835999641, 0.09543914215121999944, 0.1236370705141000004, 0.1518349988768999959, 0.1800329272397999947, 0.2082308556026999935, 0.2364287839655000167, 0.2646267123283999601, 0.2928246406912000110, 0.3210225690540999821, 0.3492204974169000331, 0.3774184257798000042, 0.4056163541427000307, 0.4338142825054999707, 0.4620122108683999973, 0.4902101392311999928, 0.5184080675940999638, 0.5466059959569999904, 0.5748039243197999859, 0.6030018526827000125, 0.6311997810455000080, 0.6593977094084000345, 0.6875956377712000300, 0.7157935661340999456, 0.7439914944969999722, 0.7721894228597999676, 0.8003873512226999942, 0.8285852795854999897, 0.8567832079484000163, 0.8849811363112999318 ),
 .UNSPECIFIED. ) ;
#50201=B_SPLINE_SURFACE_WITH_KNOTS ( 'NONE', 3, 3, ( 
 ( #17362, #1284, #6519, #60356, #49516, #44977, #12464, #50559, #23302, #23987, #27864, #49173, #33798, #22598, #43942, #55114, #35175, #56488, #25699, #35850, #25354, #8593, #14188, #20112, #24332, #35516, #45664, #19772, #19077, #30273, #41097, #36191, #29943, #62413, #8936 ),
 ( #51246, #47031, #34832, #3341, #13847, #57167, #24676, #9264, #56143, #61391, #45996, #67308, #18750, #41441, #51579, #62749, #14534, #30606, #56838, #51920, #19426, #62072, #40748, #3673, #4017, #46693, #25015, #46346, #14868, #67647, #67996, #40082, #57503, #9612, #30956 ),
 ( #52269, #4365, #13512, #8252, #29599, #50902, #2999, #66970, #40404, #61727, #48400, #68682, #10647, #163, #16584, #15562, #21479, #58541, #15209, #53305, #68334, #37560, #27086, #43155, #42133, #41780, #5742, #37224, #31993, #36887, #32337, #36536, #63781, #20453, #63085 ),
 ( #10996, #5408, #42814, #47723, #42474, #5059, #58203, #64122, #16236, #26396, #10306, #21822, #69035, #53646, #57861, #31640, #48060, #26744, #507, #58893, #21147, #9964, #47379, #15893, #27425, #59229, #31301, #11331, #52611, #64461, #37908, #32673, #53986, #20800, #4705 ) ),
 .UNSPECIFIED., .F., .F., .F.,
 ( 4, 4 ),
 ( 4, 1, 1, 1, 1, 1, 1, 1, 1, 1, 1, 1, 1, 1, 1, 1, 1, 1, 1, 1, 1, 1, 1, 1, 1, 1, 1, 1, 1, 1, 1, 1, 4 ),
 ( -0.1039086239011999951, 1.103908623900999864 ),
 ( -0.01735257130020999988, 0.01084535706264999969, 0.03904328542550000031, 0.06724121378835999641, 0.09543914215121999944, 0.1236370705141000004, 0.1518349988768999959, 0.1800329272397999947, 0.2082308556026999935, 0.2364287839655000167, 0.2646267123283999601, 0.2928246406912000110, 0.3210225690540999821, 0.3492204974169000331, 0.3774184257798000042, 0.4056163541427000307, 0.4338142825054999707, 0.4620122108683999973, 0.4902101392311999928, 0.5184080675940999638, 0.5466059959569999904, 0.5748039243197999859, 0.6030018526827000125, 0.6311997810455000080, 0.6593977094084000345, 0.6875956377712000300, 0.7157935661340999456, 0.7439914944969999722, 0.7721894228597999676, 0.8003873512226999942, 0.8285852795854999897, 0.8567832079484000163, 0.8849811363112999318 ),
 .UNSPECIFIED. ) ;
#50217=DIRECTION ( 'NONE',  ( 1.000000000000000000, 0.000000000000000000, 0.000000000000000000 ) ) ;
#50218=VERTEX_POINT ( 'NONE', #59015 ) ;
#50219=CARTESIAN_POINT ( 'NONE',  ( 9.458880069675531743, -5.224811350022368295, 8.067608271712991552 ) ) ;
#50225=CARTESIAN_POINT ( 'NONE',  ( 11.09999999999999964, -2.649999999999999911, -7.500000000000000000 ) ) ;
#50226=CARTESIAN_POINT ( 'NONE',  ( 9.051550650638001017, -2.899999999999999911, 6.227445478845999638 ) ) ;
#50234=CARTESIAN_POINT ( 'NONE',  ( 10.43353630809276922, -2.899999999999999911, -6.665341197409489382 ) ) ;
#50238=CARTESIAN_POINT ( 'NONE',  ( 10.17905590578999941, -2.899999999999999911, 6.571291218949999902 ) ) ;
#50239=CARTESIAN_POINT ( 'NONE',  ( 6.928038431245999718, -9.243192864701999412, 5.233546977967000302 ) ) ;
#50246=B_SPLINE_CURVE_WITH_KNOTS ( 'NONE', 3,
 ( #51075, #23469, #8427, #13340 ),
 .UNSPECIFIED., .F., .F.,
 ( 4, 4 ),
 ( 0.8746253901980668433, 1.000000000000000000 ),
 .UNSPECIFIED. ) ;
#50250=CARTESIAN_POINT ( 'NONE',  ( 9.792315001194999979, -4.284154785471999460, -9.000488933596999530 ) ) ;
#50253=DIRECTION ( 'NONE',  ( -1.000000000000000000, 0.000000000000000000, 0.000000000000000000 ) ) ;
#50258=CARTESIAN_POINT ( 'NONE',  ( 10.69839231854608563, -4.679932939043313311, -8.679767489841967887 ) ) ;
#50260=CYLINDRICAL_SURFACE ( 'NONE', #3839, 1.350000000000000089 ) ;
#50271=CARTESIAN_POINT ( 'NONE',  ( 9.106129440379998385, -4.192917962110999319, 5.525484568403999930 ) ) ;
#50272=ADVANCED_FACE ( 'NONE', ( #59351 ), #4885, .F. ) ;
#50287=CARTESIAN_POINT ( 'NONE',  ( 10.55813551225999980, -2.466564559586000183, 6.633531786299999844 ) ) ;
#50295=CARTESIAN_POINT ( 'NONE',  ( 8.056002428396427106, -3.587487886595424058, 5.808910377708588868 ) ) ;
#50296=CARTESIAN_POINT ( 'NONE',  ( 10.80815535238000002, -2.937528991339000140, 8.948455587554001056 ) ) ;
#50303=ORIENTED_EDGE ( 'NONE', *, *, #34943, .T. ) ;
#50306=CARTESIAN_POINT ( 'NONE',  ( 9.971744136172999262, -5.176458967229000230, -8.738385553646999426 ) ) ;
#50309=CARTESIAN_POINT ( 'NONE',  ( 11.00000000058999916, -1.300000000000000044, -9.662944685757000940 ) ) ;
#50313=ORIENTED_EDGE ( 'NONE', *, *, #69128, .T. ) ;
#50315=ORIENTED_EDGE ( 'NONE', *, *, #20598, .T. ) ;
#50316=CARTESIAN_POINT ( 'NONE',  ( 7.828418146791999099, -5.524126964933000927, 6.910359834012999691 ) ) ;
#50321=EDGE_CURVE ( 'NONE', #61617, #10663, #19352, .T. ) ;
#50322=CARTESIAN_POINT ( 'NONE',  ( 10.30480805961999913, -5.828319785709999756, -7.226592660401000678 ) ) ;
#50333=CARTESIAN_POINT ( 'NONE',  ( 8.445434020356069382, -4.175608670059299143, 6.000036809310114627 ) ) ;
#50334=CARTESIAN_POINT ( 'NONE',  ( 10.57314899745999881, -5.167567567567999731, -6.822293592207000934 ) ) ;
#50340=AXIS2_PLACEMENT_3D ( 'NONE', #49382, #12335, #59532 ) ;
#50353=CARTESIAN_POINT ( 'NONE',  ( 8.832537864289999874, -2.899999999999999911, 6.571291218949999902 ) ) ;
#50368=DIRECTION ( 'NONE',  ( 1.000000000000000000, 0.000000000000000000, 0.000000000000000000 ) ) ;
#50372=FACE_OUTER_BOUND ( 'NONE', #34869, .T. ) ;
#50384=CARTESIAN_POINT ( 'NONE',  ( 10.90437023801000116, -5.099522774867000230, 5.132565236215000049 ) ) ;
#50389=CARTESIAN_POINT ( 'NONE',  ( 10.23580444037999904, -3.621838308198000345, -8.806219190581000333 ) ) ;
#50399=CARTESIAN_POINT ( 'NONE',  ( 8.975133088423635996, -5.349981448246158955, 7.499992563499107590 ) ) ;
#50408=CARTESIAN_POINT ( 'NONE',  ( 10.32701825126999928, -5.663784181836000187, -6.682035927671000408 ) ) ;
#50410=VERTEX_POINT ( 'NONE', #26784 ) ;
#50411=CARTESIAN_POINT ( 'NONE',  ( 11.03765229723000019, -2.753052473772000130, -5.025182086257999892 ) ) ;
#50416=CARTESIAN_POINT ( 'NONE',  ( 9.869049086607999399, -5.575175898444999945, 7.724300702620999104 ) ) ;
#50434=EDGE_CURVE ( 'NONE', #51958, #46074, #11986, .T. ) ;
#50442=DIRECTION ( 'NONE',  ( -0.8660254037930258386, -1.085712934586031895E-07, 0.4999999999851149068 ) ) ;
#50444=CARTESIAN_POINT ( 'NONE',  ( 10.28315099603999982, -2.387772357283999725, 7.684266429524000408 ) ) ;
#50447=CARTESIAN_POINT ( 'NONE',  ( 9.786673210037999837, -2.381198102024000285, 7.612749732462000374 ) ) ;
#50451=ADVANCED_FACE ( 'NONE', ( #59266 ), #31695, .T. ) ;
#50461=CARTESIAN_POINT ( 'NONE',  ( 9.221306596384000187, -5.362859773739999447, -6.470306978669999154 ) ) ;
#50470=CARTESIAN_POINT ( 'NONE',  ( 8.241912900173000267, -4.599999999999999645, 6.117539782833000928 ) ) ;
#50473=CARTESIAN_POINT ( 'NONE',  ( 9.187962132612033983, -4.829473580601618465, -8.579511985892374071 ) ) ;
#50479=CARTESIAN_POINT ( 'NONE',  ( 11.10000000000000142, -2.546822617228925001, -8.294562688910756876 ) ) ;
#50481=CARTESIAN_POINT ( 'NONE',  ( 9.368002778646790318, -5.097707675583217579, -6.362033401427927615 ) ) ;
#50484=CARTESIAN_POINT ( 'NONE',  ( 10.11501430098003773, -5.350017391163235381, -7.499999134156934311 ) ) ;
#50497=CARTESIAN_POINT ( 'NONE',  ( 10.37835931247723309, -5.126777126138700957, 6.752018918791596214 ) ) ;
#50501=CARTESIAN_POINT ( 'NONE',  ( 9.395841836927720792, -2.641307054571064850, 8.590477017151444628 ) ) ;
#50505=B_SPLINE_CURVE_WITH_KNOTS ( 'NONE', 3,
 ( #14379, #14713, #25546, #15050 ),
 .UNSPECIFIED., .F., .F.,
 ( 4, 4 ),
 ( 0.000000000000000000, 1.000000000000000000 ),
 .UNSPECIFIED. ) ;
#50506=CARTESIAN_POINT ( 'NONE',  ( 11.04878770808000077, -5.241617395113999933, -5.060603459065999843 ) ) ;
#50509=CARTESIAN_POINT ( 'NONE',  ( 10.31167756636999933, -2.874479384703000129, 8.900026329558999194 ) ) ;
#50517=PLANE ( 'NONE',  #50676 ) ;
#50534=CARTESIAN_POINT ( 'NONE',  ( 10.87173209806000074, -5.066009632528999163, 5.128393832781000583 ) ) ;
#50538=CARTESIAN_POINT ( 'NONE',  ( 7.613711861438999584, -4.858906194260998568, 6.437673909214002954 ) ) ;
#50546=CARTESIAN_POINT ( 'NONE',  ( 7.808687732304345985, -3.149842433176995193, 6.423753202348916780 ) ) ;
#50552=B_SPLINE_CURVE_WITH_KNOTS ( 'NONE', 3,
 ( #6421, #43148, #28109, #38240, #37550, #1534, #10639, #17624, #33359, #844, #59569, #37900, #58533, #21814, #49080, #59914, #64113, #17267 ),
 .UNSPECIFIED., .F., .F.,
 ( 4, 2, 2, 2, 2, 2, 2, 2, 4 ),
 ( 0.000000000000000000, 0.1070823790245061802, 0.2141647580490123604, 0.3212471370735185405, 0.4283295160980247207, 0.5354118951225302903, 0.6424942741470358598, 0.7495766531715415404, 0.8566590321960471099 ),
 .UNSPECIFIED. ) ;
#50554=CARTESIAN_POINT ( 'NONE',  ( 8.601293559883481876, -4.584462925737535777, 5.854726763232750208 ) ) ;
#50559=CARTESIAN_POINT ( 'NONE',  ( 9.848253563160000112, -4.436921580929999998, 6.148020168057000134 ) ) ;
#50560=ORIENTED_EDGE ( 'NONE', *, *, #48533, .T. ) ;
#50562=CARTESIAN_POINT ( 'NONE',  ( 9.587879440377001572, -3.762710033898000184, 8.787827024292999667 ) ) ;
#50573=FACE_OUTER_BOUND ( 'NONE', #50621, .T. ) ;
#50576=CARTESIAN_POINT ( 'NONE',  ( 9.765375278055641317, -5.100000000000000533, 6.445686799077642526 ) ) ;
#50586=B_SPLINE_CURVE_WITH_KNOTS ( 'NONE', 3,
 ( #21097, #36481, #48009, #109 ),
 .UNSPECIFIED., .F., .F.,
 ( 4, 4 ),
 ( 0.8744711628437967788, 1.000000000000000000 ),
 .UNSPECIFIED. ) ;
#50596=CARTESIAN_POINT ( 'NONE',  ( 10.09133114265999964, -2.216726401468000152, -8.007130485478999304 ) ) ;
#50598=CARTESIAN_POINT ( 'NONE',  ( 9.051836062923225512, -4.773613032258291256, 8.611988568103887687 ) ) ;
#50604=FACE_OUTER_BOUND ( 'NONE', #15883, .T. ) ;
#50609=CARTESIAN_POINT ( 'NONE',  ( 5.700000001242999659, 1.249999998757000075, -1.883720587326999896E-09 ) ) ;
#50616=CARTESIAN_POINT ( 'NONE',  ( 7.694004440376999376, -5.850279024084999335, 6.784181137144999596 ) ) ;
#50617=AXIS2_PLACEMENT_3D ( 'NONE', #49267, #1040, #13862 ) ;
#50621=EDGE_LOOP ( 'NONE', ( #68290, #33753, #58481, #23735, #23893, #37222, #64568 ) ) ;
#50623=EDGE_CURVE ( 'NONE', #8532, #27164, #16074, .T. ) ;
#50631=CARTESIAN_POINT ( 'NONE',  ( 10.02202195053999922, -3.298019507654999849, 5.700533868754000366 ) ) ;
#50634=CARTESIAN_POINT ( 'NONE',  ( -14.79345512259999929, -10.48174933044999868, 5.405686454350000503 ) ) ;
#50636=CARTESIAN_POINT ( 'NONE',  ( 7.965749382700749059, -2.298601573531716458, 7.139296998118509485 ) ) ;
#50638=CARTESIAN_POINT ( 'NONE',  ( 9.476374593785998002, -5.098398394707999159, 6.305533045879999854 ) ) ;
#50644=ORIENTED_EDGE ( 'NONE', *, *, #21304, .F. ) ;
#50645=CARTESIAN_POINT ( 'NONE',  ( 9.136057238048000073, -5.084840204920000772, -6.477689566282000655 ) ) ;
#50648=CARTESIAN_POINT ( 'NONE',  ( 9.443723707566000769, -5.531435376468999188, -8.256621485025000595 ) ) ;
#50656=EDGE_LOOP ( 'NONE', ( #14656, #37180, #3333, #27782, #612 ) ) ;
#50659=ORIENTED_EDGE ( 'NONE', *, *, #48444, .F. ) ;
#50660=CARTESIAN_POINT ( 'NONE',  ( 7.930394353207000258, -3.164807285701999984, 9.104732190648000767 ) ) ;
#50661=LINE ( 'NONE', #2761, #23445 ) ;
#50665=CARTESIAN_POINT ( 'NONE',  ( 11.03905685320999908, -3.855072944465999907, -9.179476187420998912 ) ) ;
#50676=AXIS2_PLACEMENT_3D ( 'NONE', #44605, #34793, #66589 ) ;
#50677=CARTESIAN_POINT ( 'NONE',  ( 8.570147025264834184, -5.044616720184398773, 6.241050644686979787 ) ) ;
#50687=DIRECTION ( 'NONE',  ( 0.000000000000000000, 1.000000000000000000, 0.000000000000000000 ) ) ;
#50691=B_SPLINE_CURVE_WITH_KNOTS ( 'NONE', 3,
 ( #671, #5901, #11156, #23022, #1356 ),
 .UNSPECIFIED., .F., .F.,
 ( 4, 1, 4 ),
 ( 0.000000000000000000, 0.5000000000000000000, 1.000000000000000000 ),
 .UNSPECIFIED. ) ;
#50703=CARTESIAN_POINT ( 'NONE',  ( 10.81962466143134804, -4.116062333401275808, 9.235854717643961820 ) ) ;
#50704=CARTESIAN_POINT ( 'NONE',  ( 8.213543146793000460, -3.608524635952000459, 5.913372239166000632 ) ) ;
#50708=VERTEX_POINT ( 'NONE', #39510 ) ;
#50720=CARTESIAN_POINT ( 'NONE',  ( 7.437254440376999121, -2.216884807317999861, 8.370075800106999253 ) ) ;
#50721=VERTEX_POINT ( 'NONE', #1325 ) ;
#50730=CARTESIAN_POINT ( 'NONE',  ( 10.66405417102151887, -5.056489201926463117, 5.060659056817709889 ) ) ;
#50734=CARTESIAN_POINT ( 'NONE',  ( 10.34939194037999854, -2.653148377029999949, -7.312413909354000374 ) ) ;
#50739=AXIS2_PLACEMENT_3D ( 'NONE', #23568, #49801, #12744 ) ;
#50742=CARTESIAN_POINT ( 'NONE',  ( 10.35685100253999913, -2.832432432432000269, -6.822293592207000934 ) ) ;
#50743=ORIENTED_EDGE ( 'NONE', *, *, #55406, .F. ) ;
#50751=CARTESIAN_POINT ( 'NONE',  ( 10.70441271436000008, -3.444516450945999786, 6.009051312948000323 ) ) ;
#50752=EDGE_CURVE ( 'NONE', #36042, #68830, #55852, .T. ) ;
#50754=CARTESIAN_POINT ( 'NONE',  ( 10.71983009893999927, -3.571743996388999864, -5.696159701115999674 ) ) ;
#50756=ADVANCED_FACE ( 'NONE', ( #50604 ), #51077, .T. ) ;
#50757=EDGE_CURVE ( 'NONE', #56244, #7917, #20926, .T. ) ;
#50758=CARTESIAN_POINT ( 'NONE',  ( 10.69180966889106088, -2.945054940980131875, -5.060957807827213273 ) ) ;
#50759=ORIENTED_EDGE ( 'NONE', *, *, #24784, .T. ) ;
#50767=CARTESIAN_POINT ( 'NONE',  ( 9.646285452541999206, -2.591464128784999765, 6.760053199270999791 ) ) ;
#50772=ORIENTED_EDGE ( 'NONE', *, *, #35203, .F. ) ;
#50778=VECTOR ( 'NONE', #59984, 1000.000000000000227 ) ;
#50779=B_SPLINE_SURFACE_WITH_KNOTS ( 'NONE', 3, 3, ( 
 ( #5225, #56992, #46511, #68156, #10465, #37048, #9778, #20621, #15031, #67813, #58028, #58363, #41602, #4527, #30433, #4874, #31807, #41258, #3837, #62910, #36355, #25863, #20967, #47196, #14353, #68498, #42304, #53124, #41945, #19937, #25176, #62573, #63254, #47888, #21306 ),
 ( #37730, #48914, #60093, #38416, #59741, #11842, #6246, #28277, #17442, #5905, #16738, #38067, #32155, #33180, #59392, #54498, #1359, #64283, #6945, #58709, #43327, #27588, #10813, #64632, #6598, #49598, #53806, #16400, #22676, #32493, #1705, #53471, #27246, #59056, #27939 ),
 ( #11492, #32837, #11158, #49250, #5564, #54149, #42635, #37386, #1022, #22332, #43672, #38769, #12199, #64969, #17083, #26906, #44021, #42976, #65324, #33527, #54846, #63944, #16056, #48220, #326, #21641, #48569, #673, #21985, #2058, #40480, #61807, #18827, #39112, #34907 ),
 ( #13924, #51320, #13245, #67046, #35251, #28633, #60436, #44374, #3076, #24061, #34570, #23376, #56565, #8672, #40153, #12543, #56222, #55189, #44715, #66359, #55885, #45396, #8332, #28986, #29675, #61128, #65672, #33874, #45737, #60778, #7990, #7293, #50978, #30019, #61467 ) ),
 .UNSPECIFIED., .F., .F., .F.,
 ( 4, 4 ),
 ( 4, 1, 1, 1, 1, 1, 1, 1, 1, 1, 1, 1, 1, 1, 1, 1, 1, 1, 1, 1, 1, 1, 1, 1, 1, 1, 1, 1, 1, 1, 1, 1, 4 ),
 ( -0.1039086239011999951, 1.103908623900999864 ),
 ( 0.2233333333344000027, 0.2480800653604999795, 0.2728267973865999840, 0.2975735294126999886, 0.3223202614387999931, 0.3470669934649999733, 0.3718137254910999778, 0.3965604575171999824, 0.4213071895433000424, 0.4460539215694000470, 0.4708006535954999960, 0.4955473856216000006, 0.5202941176476999496, 0.5450408496738000652, 0.5697875816999000698, 0.5945343137260000743, 0.6192810457521999989, 0.6440277777783000035, 0.6687745098044000081, 0.6935212418305000126, 0.7182679738566000172, 0.7430147058827000217, 0.7677614379088000263, 0.7925081699349000308, 0.8172549019609999243, 0.8420016339870999289, 0.8667483660132000445, 0.8914950980394000801, 0.9162418300655000847, 0.9409885620915999782, 0.9657352941176999828, 0.9904820261437999873, 1.015228758169999912 ),
 .UNSPECIFIED. ) ;
#50783=FACE_OUTER_BOUND ( 'NONE', #57604, .T. ) ;
#50785=CARTESIAN_POINT ( 'NONE',  ( 9.685492310842999331, -4.505165106450999879, -8.732017808253001334 ) ) ;
#50795=CARTESIAN_POINT ( 'NONE',  ( 9.934999999999998721, -4.640430492595999823, -9.117542781427999898 ) ) ;
#50797=CARTESIAN_POINT ( 'NONE',  ( 9.352255147285999826, -2.817754448466000206, 6.388456890282999900 ) ) ;
#50801=LINE ( 'NONE', #41335, #1969 ) ;
#50804=ORIENTED_EDGE ( 'NONE', *, *, #23853, .F. ) ;
#50809=FACE_OUTER_BOUND ( 'NONE', #30969, .T. ) ;
#50811=CARTESIAN_POINT ( 'NONE',  ( 9.084135711596999840, -5.371875912611999482, -7.370590366721999409 ) ) ;
#50817=LINE ( 'NONE', #8507, #49938 ) ;
#50830=CYLINDRICAL_SURFACE ( 'NONE', #64974, 0.5000000000000002220 ) ;
#50839=ORIENTED_EDGE ( 'NONE', *, *, #44982, .F. ) ;
#50847=CARTESIAN_POINT ( 'NONE',  ( 9.354587383407045209, -3.357689054377400062, 9.116474598616981950 ) ) ;
#50855=EDGE_CURVE ( 'NONE', #42399, #20484, #38733, .T. ) ;
#50856=CARTESIAN_POINT ( 'NONE',  ( 10.80815535238000002, -2.937528991339000140, 8.948455587554001056 ) ) ;
#50858=FACE_OUTER_BOUND ( 'NONE', #26493, .T. ) ;
#50862=CARTESIAN_POINT ( 'NONE',  ( 7.000000000000000000, -0.2897247358851999799, 3.000000000000000000 ) ) ;
#50864=CARTESIAN_POINT ( 'NONE',  ( 7.413221459149189840, -4.978041439725138240, 6.521863944591406614 ) ) ;
#50869=CARTESIAN_POINT ( 'NONE',  ( 11.07071167063000061, -5.425576677726000163, 5.078384236784999395 ) ) ;
#50874=CARTESIAN_POINT ( 'NONE',  ( 10.71991265383000069, -2.957947977237000092, -5.111881366068000254 ) ) ;
#50877=CARTESIAN_POINT ( 'NONE',  ( 9.865041550948088656, -2.650034642413194419, -7.500002425457253707 ) ) ;
#50885=VECTOR ( 'NONE', #23461, 1000.000000000000114 ) ;
#50896=B_SPLINE_CURVE_WITH_KNOTS ( 'NONE', 3,
 ( #30102, #51405, #67130, #18568, #24497, #39196, #39894, #51065, #45819, #61214, #19240, #44797, #13331, #39544, #60518, #12628, #66100, #60866, #34997, #12982, #23804, #45136, #34304, #33956, #8073, #29416, #40568, #13668, #3501, #3167, #50034, #2818, #61895, #35339, #14010, #45481, #8760, #55627, #35680, #3838, #19595, #42305, #63607, #46512, #56993, #37049, #10130, #46854, #25864, #68157, #25177, #15723, #41946, #63255, #15381, #9779, #68499, #4188, #36710, #20622, #9095, #58030, #4875, #41603, #47545, #51745, #62911, #67814, #40915, #62237, #19938, #41260, #31462, #62574, #9429, #58364, #4528, #25525, #15032, #26217, #47197, #52780, #31808, #68849, #53125, #52432, #20968, #10466, #5226, #36356, #57328, #46166, #30434, #14694, #14354, #57671, #67473, #20277, #31129, #36012, #30772, #52084, #48915, #59742, #64970, #33528, #60094, #26563, #11843, #12200, #47889, #33181, #59057, #69194, #37387, #6599, #42636, #54847, #21307, #27941, #54499, #22677, #37731, #32494, #27589, #26907, #16401, #63945, #1360, #16057, #49251, #1023, #64633, #674, #17443, #58710, #10814, #11493, #22334, #32156, #53472, #42977, #44022, #65325, #21986, #59394, #43329, #38770, #5566, #16740, #43673, #38068, #32838, #6247, #64284, #11159, #48221, #327, #5906, #21642, #53807, #54150, #27247, #48570, #17084, #38417, #60779, #34571, #39806, #23717, #61470, #50979, #2393, #24062, #45052, #66360, #55887, #23377, #44716, #29676, #33875, #45738, #7991, #28634, #13246, #18136, #49946, #56223, #67048, #12893, #29324, #7294, #65673, #19157, #40154, #7639, #50636, #28987, #55192, #3077, #2737, #45397, #61129, #66707, #34221, #18828, #13589, #17795, #34909, #50295, #12544, #8333, #24410, #2059, #40481, #18481, #39114, #61808, #13926, #35252, #6946, #39458, #28278, #49599, #55541, #1706, #23025, #44375, #60437, #66013, #9692, #19850, #26127, #9341, #30686, #20532, #3753, #30350, #25093, #31039, #63520, #30020, #25434, #57585, #35928, #51994, #8673, #20878, #10038, #36618, #41858, #46077, #46423, #9009, #68070, #4098, #24752, #52347, #51658, #42215, #31377, #67385, #57942, #3417, #15634, #51322, #52689, #63164, #19507, #20187, #35596, #40824, #46767, #56568, #62150, #4785, #14268, #62826, #56910, #67725, #41515, #47454, #41179, #62486, #14944, #4441, #14610, #57240, #36270, #68410, #25780, #47111, #68759, #15293, #37642, #16659, #58974, #63858, #33097, #32752, #54065, #1279, #22593, #38330, #11076, #64887, #10382, #32411, #27503, #17001, #53726, #59660, #42550, #5825, #58623, #31720, #53042, #37301, #32071, #6162, #10724, #21899, #48140, #53386, #5137, #27162, #590, #11756, #48829, #43936, #938, #65240, #43237, #22250, #6514, #43588, #48483, #243, #27859, #26474, #15972, #64543, #54414, #49167, #37984, #47807, #69113, #59310, #36965, #11411, #58279, #21221, #5487, #26822, #21557, #42893, #64200, #16315, #39726, #33794, #38683, #28551, #28907, #44637, #49861, #2653, #23296, #44973, #29244, #55109, #7214, #7553, #44292, #12460, #60004, #50554, #33444, #55805 ),
 .UNSPECIFIED., .F., .F.,
 ( 4, 2, 2, 2, 2, 2, 1, 1, 1, 2, 2, 2, 2, 2, 2, 1, 2, 2, 2, 2, 1, 2, 2, 2, 2, 1, 1, 2, 2, 1, 2, 2, 2, 2, 2, 2, 2, 2, 2, 2, 2, 2, 2, 2, 2, 2, 2, 2, 1, 2, 2, 2, 2, 1, 1, 1, 2, 2, 2, 2, 2, 2, 2, 2, 1, 2, 2, 2, 2, 2, 2, 1, 2, 1, 2, 2, 1, 2, 2, 2, 2, 2, 1, 1, 2, 2, 2, 2, 2, 2, 2, 2, 1, 2, 2, 2, 2, 2, 2, 2, 2, 2, 2, 1, 2, 2, 2, 2, 1, 1, 1, 2, 2, 2, 2, 2, 2, 2, 2, 1, 1, 2, 2, 2, 2, 2, 2, 2, 1, 1, 2, 2, 2, 2, 1, 1, 1, 2, 2, 2, 2, 2, 2, 2, 2, 2, 2, 2, 2, 2, 1, 2, 2, 2, 2, 1, 2, 2, 2, 2, 1, 1, 1, 2, 2, 2, 2, 2, 2, 2, 2, 1, 2, 2, 2, 2, 2, 2, 2, 1, 1, 2, 2, 2, 2, 1, 1, 1, 2, 2, 2, 2, 2, 2, 2, 2, 1, 2, 2, 2, 2, 2, 1, 2, 2, 2, 2, 1, 2, 2, 4 ),
 ( 0.000000000000000000, 0.01562500000001094264, 0.03125000000002188527, 0.06250000000004377054, 0.07031250000004928002, 0.07421875000005202783, 0.07617187500005341561, 0.07714843750005409562, 0.07763671875005451195, 0.07788085937505478951, 0.07812500000005508094, 0.08203125000006007694, 0.08398437500006267209, 0.08447265625006321332, 0.08496093750006374068, 0.08593750000006465661, 0.09375000000007154000, 0.09765625000007492618, 0.09814453125007535639, 0.09863281250007577272, 0.09960937500007630008, 0.1015625000000773409, 0.1093750000000812406, 0.1113281250000822259, 0.1118164062500824757, 0.1123046875000827116, 0.1132812500000833084, 0.1171875000000856676, 0.1210937500000880268, 0.1230468750000891509, 0.1240234375000897199, 0.1250000000000902611, 0.1562500000001111611, 0.1718750000001215972, 0.1875000000001320333, 0.1953125000001372236, 0.1962890625001378897, 0.1972656250001385281, 0.1992187500001398603, 0.2031250000001424694, 0.2070312500001451061, 0.2089843750001464384, 0.2099609375001471323, 0.2109375000001477984, 0.2187500000001537104, 0.2226562500001565970, 0.2231445312501569300, 0.2236328125001572908, 0.2246093750001579570, 0.2265625000001592892, 0.2343750000001645628, 0.2421875000001698364, 0.2460937500001725009, 0.2480468750001738609, 0.2490234375001745271, 0.2495117187501748601, 0.2497558593751748324, 0.2500000000001748046, 0.2656250000001770806, 0.2812500000001793565, 0.3125000000001840195, 0.3203125000001850742, 0.3242187500001856293, 0.3261718750001860179, 0.3271484375001862399, 0.3276367187501863509, 0.3281250000001865175, 0.3320312500001871281, 0.3339843750001875167, 0.3344726562501874056, 0.3349609375001872946, 0.3359375000001870726, 0.3437500000001854628, 0.3476562500001845746, 0.3481445312501844636, 0.3486328125001843525, 0.3496093750001842415, 0.3515625000001838529, 0.3593750000001824096, 0.3671875000001809108, 0.3710937500001801892, 0.3730468750001795231, 0.3740234375001792455, 0.3745117187501793010, 0.3747558593751790235, 0.3750000000001787459, 0.4062500000001486589, 0.4218750000001336153, 0.4375000000001185718, 0.4453125000001111333, 0.4462890625001101896, 0.4467773437501098011, 0.4472656250001093570, 0.4492187500001074696, 0.4531250000001035283, 0.4570312500000995315, 0.4589843750000976441, 0.4599609375000966449, 0.4609375000000956457, 0.4687500000000878742, 0.4726562500000838773, 0.4731445312500832112, 0.4736328125000825451, 0.4746093750000812128, 0.4765625000000783817, 0.4843750000000671130, 0.4921875000000557887, 0.4960937500000501821, 0.4980468750000473510, 0.4990234375000460743, 0.4995117187500454081, 0.4997558593750451861, 0.5000000000000449640, 0.5156250000000307532, 0.5312500000000164313, 0.5624999999999878986, 0.5703124999999807931, 0.5712890624999799050, 0.5715332031249795719, 0.5717773437499793499, 0.5722656249999789058, 0.5742187499999770184, 0.5781249999999733546, 0.5859374999999660272, 0.5937499999999586997, 0.5976562499999550360, 0.5981445312499544809, 0.5983886718749541478, 0.5986328124999537037, 0.5996093749999521494, 0.6015624999999492628, 0.6093749999999371614, 0.6171874999999250599, 0.6210937499999190647, 0.6230468749999160671, 0.6240234374999148459, 0.6245117187499145128, 0.6247558593749144018, 0.6249999999999141798, 0.6562499999998935296, 0.6718749999998830935, 0.6874999999998727684, 0.6953124999998676614, 0.6962890624998668843, 0.6972656249998661071, 0.6992187499998651079, 0.7031249999998631095, 0.7070312499998612221, 0.7089843749998602229, 0.7099609374998596678, 0.7109374999998592237, 0.7187499999998558931, 0.7226562499998542277, 0.7231445312498538946, 0.7236328124998535616, 0.7246093749998531175, 0.7265624999998522293, 0.7343749999998488986, 0.7421874999998456790, 0.7460937499998440137, 0.7480468749998432365, 0.7490234374998427924, 0.7495117187498425704, 0.7497558593748424594, 0.7499999999998424594, 0.7656249999998324673, 0.7812499999998223643, 0.8124999999998024913, 0.8203124999997976063, 0.8212890624997970512, 0.8217773437497968292, 0.8222656249997966071, 0.8242187499997956079, 0.8281249999997936095, 0.8359374999997895017, 0.8437499999997853939, 0.8476562499997833955, 0.8481445312497839506, 0.8483886718747842837, 0.8486328124997845057, 0.8496093749997857270, 0.8515624999997882805, 0.8593749999997979394, 0.8671874999998075983, 0.8710937499998125944, 0.8730468749998150368, 0.8740234374998161471, 0.8745117187498168132, 0.8747558593748171463, 0.8749999999998173683, 0.9062499999998596678, 0.9218749999998806510, 0.9374999999999017453, 0.9453124999999122924, 0.9462890624999136246, 0.9467773437499142908, 0.9472656249999149569, 0.9492187499999179545, 0.9531249999999238387, 0.9570312499999298339, 0.9589843749999327205, 0.9599609374999341638, 0.9609374999999357181, 0.9687499999999472644, 0.9726562499999531486, 0.9731445312499539257, 0.9736328124999547029, 0.9746093749999563682, 0.9765624999999596989, 0.9843749999999731326, 1.000000000000000000 ),
 .UNSPECIFIED. ) ;
#50902=CARTESIAN_POINT ( 'NONE',  ( 9.555699158955999195, -2.440755924888999839, 6.680881588809999272 ) ) ;
#50905=CARTESIAN_POINT ( 'NONE',  ( 8.496691940379001551, -5.198566224659999513, 8.332559954171999905 ) ) ;
#50914=CARTESIAN_POINT ( 'NONE',  ( 10.71256247620999957, -5.951803124515000043, 7.233045248871000865 ) ) ;
#50916=EDGE_CURVE ( 'NONE', #2080, #65525, #13549, .T. ) ;
#50939=CARTESIAN_POINT ( 'NONE',  ( 10.05204995789999955, -2.669899884077999719, -8.791535702747999892 ) ) ;
#50942=CARTESIAN_POINT ( 'NONE',  ( 9.016026733244713043, -5.181567068652970676, 8.154973437734131636 ) ) ;
#50947=FACE_OUTER_BOUND ( 'NONE', #63772, .T. ) ;
#50949=DIRECTION ( 'NONE',  ( 1.000000000000000000, 0.000000000000000000, 0.000000000000000000 ) ) ;
#50958=CARTESIAN_POINT ( 'NONE',  ( 7.384456853207000293, -3.346260729029000291, 6.002247316312999459 ) ) ;
#50960=LINE ( 'NONE', #25764, #25568 ) ;
#50962=ORIENTED_EDGE ( 'NONE', *, *, #52334, .F. ) ;
#50974=CARTESIAN_POINT ( 'NONE',  ( 11.05935368890999904, -2.480241580537000168, 6.610077204591000566 ) ) ;
#50978=CARTESIAN_POINT ( 'NONE',  ( 10.19794194037999979, -4.262172867567000090, -8.834326937932999613 ) ) ;
#50979=CARTESIAN_POINT ( 'NONE',  ( 7.908383208917886265, -2.485710556326794496, 8.356913658884913332 ) ) ;
#50980=CARTESIAN_POINT ( 'NONE',  ( 10.40727044253999978, -3.797905333157999941, 5.889909992361999969 ) ) ;
#50981=AXIS2_PLACEMENT_3D ( 'NONE', #5479, #22241, #37294 ) ;
#50985=CARTESIAN_POINT ( 'NONE',  ( 10.31663362093999936, -4.574952992312999456, -4.565089889767000031 ) ) ;
#50987=EDGE_LOOP ( 'NONE', ( #54004, #55603, #5843, #7134 ) ) ;
#51001=CARTESIAN_POINT ( 'NONE',  ( 8.662855646795000197, -2.741638482234999952, 6.457327039244000311 ) ) ;
#51003=ORIENTED_EDGE ( 'NONE', *, *, #56145, .T. ) ;
#51006=CARTESIAN_POINT ( 'NONE',  ( 10.81188185321000006, -4.614147550108000928, -5.930138617968999881 ) ) ;
#51017=SHAPE_REPRESENTATION_RELATIONSHIP ( 'NONE' , 'NONE' ,  #30050, #42688 ) ;
#51045=CARTESIAN_POINT ( 'NONE',  ( 8.946004440379999423, -5.458705123429999695, 7.456451825584000659 ) ) ;
#51046=DIRECTION ( 'NONE',  ( 0.8480635683784329970, -0.3746919961710145075, 0.3746919961710145075 ) ) ;
#51058=CARTESIAN_POINT ( 'NONE',  ( 8.216851002544000693, -2.832432432432000269, 6.822293592207000934 ) ) ;
#51060=CARTESIAN_POINT ( 'NONE',  ( 8.502043146794999728, -3.869396851328000153, 5.695656592546999519 ) ) ;
#51065=CARTESIAN_POINT ( 'NONE',  ( 7.410149690637857667, -2.473805498145990711, 8.336998697800455105 ) ) ;
#51071=CARTESIAN_POINT ( 'NONE',  ( 10.86578724599310775, -5.674343923958758751, -8.061244989951715567 ) ) ;
#51075=CARTESIAN_POINT ( 'NONE',  ( 10.42499241036559532, -5.349775919985432004, 7.500001834605715345 ) ) ;
#51076=CARTESIAN_POINT ( 'NONE',  ( 10.31152944037999930, -2.716820959546999870, -7.950167805575999225 ) ) ;
#51077=CONICAL_SURFACE ( 'NONE', #34316, 10.65000781019999998, 0.7853981633972997312 ) ;
#51087=CARTESIAN_POINT ( 'NONE',  ( 8.962844625895410644, -5.333198074240036668, 7.284253336463978989 ) ) ;
#51094=CARTESIAN_POINT ( 'NONE',  ( 10.01532628870999986, -4.946995631616999844, 8.559221361189001342 ) ) ;
#51101=CARTESIAN_POINT ( 'NONE',  ( 11.07128162083999889, -5.551565104116000349, -5.077697045197999692 ) ) ;
#51105=CARTESIAN_POINT ( 'NONE',  ( 10.90000000000000036, -4.000000000000000000, 7.500000000000000000 ) ) ;
#51108=CARTESIAN_POINT ( 'NONE',  ( 10.59303089732000025, -2.436232726560000117, 7.793465286118999913 ) ) ;
#51125=CARTESIAN_POINT ( 'NONE',  ( 9.262725409949998934, -4.818302824158000597, -8.808202952968999355 ) ) ;
#51137=CARTESIAN_POINT ( 'NONE',  ( 10.34521071928999980, -2.724119865955000108, 6.497322598008000050 ) ) ;
#51139=CARTESIAN_POINT ( 'NONE',  ( 9.051550650638001017, -2.899999999999999911, 6.227445478845999638 ) ) ;
#51143=DIRECTION ( 'NONE',  ( 1.000000000000000000, 0.000000000000000000, 0.000000000000000000 ) ) ;
#51144=CARTESIAN_POINT ( 'NONE',  ( 9.332537864288001472, -2.899999999999999911, 6.571291218949999902 ) ) ;
#51145=VERTEX_POINT ( 'NONE', #67015 ) ;
#51147=ADVANCED_FACE ( 'NONE', ( #50947 ), #12787, .T. ) ;
#51149=CARTESIAN_POINT ( 'NONE',  ( 10.46536477495381590, -4.887125000223165650, -4.987012270671904446 ) ) ;
#51156=CARTESIAN_POINT ( 'NONE',  ( 9.790745838555999114, -4.301175052434000001, -8.935144319903001175 ) ) ;
#51157=CARTESIAN_POINT ( 'NONE',  ( 10.11094409420000062, -5.100000000000000533, -6.571291218949999902 ) ) ;
#51171=VERTEX_POINT ( 'NONE', #49135 ) ;
#51180=VERTEX_POINT ( 'NONE', #65206 ) ;
#51199=CARTESIAN_POINT ( 'NONE',  ( 11.04647262364999882, -5.245405433888000069, -5.117543298298000032 ) ) ;
#51204=ORIENTED_EDGE ( 'NONE', *, *, #13546, .F. ) ;
#51209=DIRECTION ( 'NONE',  ( -1.000000000000000000, 0.000000000000000000, 2.893429392099000104E-14 ) ) ;
#51215=ORIENTED_EDGE ( 'NONE', *, *, #55265, .T. ) ;
#51216=DIRECTION ( 'NONE',  ( -1.000000000000000000, 0.000000000000000000, 0.000000000000000000 ) ) ;
#51218=CARTESIAN_POINT ( 'NONE',  ( 9.881157842586999251, -5.290169207169999943, -8.858081286661999343 ) ) ;
#51222=CARTESIAN_POINT ( 'NONE',  ( 11.04678944127999962, -5.235596213805000509, -5.039805523473999571 ) ) ;
#51230=VERTEX_POINT ( 'NONE', #57817 ) ;
#51242=CARTESIAN_POINT ( 'NONE',  ( 9.573148997458000409, -5.167567567567999731, -6.822293592207000934 ) ) ;
#51246=CARTESIAN_POINT ( 'NONE',  ( 9.423521818475000700, -4.993993578306000103, 8.578110568283999982 ) ) ;
#51247=VERTEX_POINT ( 'NONE', #48361 ) ;
#51248=CARTESIAN_POINT ( 'NONE',  ( 9.424850088744616272, -5.349972419855331118, 7.500009359253513530 ) ) ;
#51249=CARTESIAN_POINT ( 'NONE',  ( 8.560879440379000727, -4.228293421747000735, 8.941387937291999322 ) ) ;
#51253=CARTESIAN_POINT ( 'NONE',  ( 10.99570321855803456, -5.445259508076158106, -7.243346639202360215 ) ) ;
#51258=VERTEX_POINT ( 'NONE', #64082 ) ;
#51266=CARTESIAN_POINT ( 'NONE',  ( 10.95823604978370547, -2.826496578562578854, -6.686434942404212656 ) ) ;
#51270=ADVANCED_FACE ( 'NONE', ( #37875 ), #52573, .T. ) ;
#51273=ORIENTED_EDGE ( 'NONE', *, *, #32739, .T. ) ;
#51280=CARTESIAN_POINT ( 'NONE',  ( 10.75911128370000114, -4.477561100530000004, -5.708582007447000173 ) ) ;
#51283=EDGE_LOOP ( 'NONE', ( #33017, #46080, #48117 ) ) ;
#51292=B_SPLINE_CURVE_WITH_KNOTS ( 'NONE', 3,
 ( #29177, #40007, #35445, #2586 ),
 .UNSPECIFIED., .F., .F.,
 ( 4, 4 ),
 ( 0.000000000000000000, 1.000000000000000000 ),
 .UNSPECIFIED. ) ;
#51299=CARTESIAN_POINT ( 'NONE',  ( 7.833769353207999941, -2.583664704444999849, 6.684748541034000624 ) ) ;
#51317=CARTESIAN_POINT ( 'NONE',  ( 11.09999999999999964, -5.299999999999999822, -5.157071272631999825 ) ) ;
#51318=EDGE_LOOP ( 'NONE', ( #57231, #51949, #54331, #9603 ) ) ;
#51320=CARTESIAN_POINT ( 'NONE',  ( 11.35905860703999970, -2.719090443614000208, -7.157642341559000698 ) ) ;
#51322=CARTESIAN_POINT ( 'NONE',  ( 8.233317044961992792, -5.585056236752896197, 8.216725689016870504 ) ) ;
#51326=FACE_OUTER_BOUND ( 'NONE', #8538, .T. ) ;
#51331=VERTEX_POINT ( 'NONE', #56375 ) ;
#51332=CARTESIAN_POINT ( 'NONE',  ( 9.235799540957000175, -4.950980172046000050, -5.959730545597000884 ) ) ;
#51333=DIRECTION ( 'NONE',  ( 0.000000000000000000, 1.000000000000000000, 0.000000000000000000 ) ) ;
#51341=B_SPLINE_CURVE_WITH_KNOTS ( 'NONE', 3,
 ( #52425, #36350, #4522, #42299 ),
 .UNSPECIFIED., .F., .F.,
 ( 4, 4 ),
 ( 0.000000000000000000, 1.000000000000000000 ),
 .UNSPECIFIED. ) ;
#51342=CARTESIAN_POINT ( 'NONE',  ( 8.470293146793999028, -4.255646685191999623, 9.114089645792999406 ) ) ;
#51348=CARTESIAN_POINT ( 'NONE',  ( 10.90246814679000131, -4.554787328265999413, -6.081873034041000103 ) ) ;
#51358=CARTESIAN_POINT ( 'NONE',  ( 10.33235660140000078, -4.841932061664000031, 4.868350078553000060 ) ) ;
#51384=CARTESIAN_POINT ( 'NONE',  ( 10.62947109217999930, -5.100000000000000533, 6.152188490330000370 ) ) ;
#51385=CARTESIAN_POINT ( 'NONE',  ( 8.881816940380000247, -4.977917894183000236, 6.416767031887000705 ) ) ;
#51388=CIRCLE ( 'NONE', #67003, 1.000000000000000000 ) ;
#51391=B_SPLINE_CURVE_WITH_KNOTS ( 'NONE', 3,
 ( #22694, #44037, #54863, #49615 ),
 .UNSPECIFIED., .F., .F.,
 ( 4, 4 ),
 ( 0.000000000000000000, 1.000000000000000000 ),
 .UNSPECIFIED. ) ;
#51397=CARTESIAN_POINT ( 'NONE',  ( 7.000000000000000000, -7.356391799243646723, 3.356391799243647167 ) ) ;
#51401=CARTESIAN_POINT ( 'NONE',  ( 8.207504440379000954, -5.944572422272999646, 7.106845737860000511 ) ) ;
#51402=ORIENTED_EDGE ( 'NONE', *, *, #50855, .F. ) ;
#51405=CARTESIAN_POINT ( 'NONE',  ( 7.332307259148439726, -3.827065593140268174, 9.239363644322621028 ) ) ;
#51406=CARTESIAN_POINT ( 'NONE',  ( 10.49640421544676983, -5.348966112464561995, 7.853238477522131333 ) ) ;
#51412=CARTESIAN_POINT ( 'NONE',  ( 10.27427173614549716, -4.712533253186579785, 4.944156917096328208 ) ) ;
#51433=CARTESIAN_POINT ( 'NONE',  ( 9.959635380193999410, -5.406637819064000539, 7.700301345050000634 ) ) ;
#51438=VERTEX_POINT ( 'NONE', #36247 ) ;
#51439=AXIS2_PLACEMENT_3D ( 'NONE', #30761, #26205, #68487 ) ;
#51440=CARTESIAN_POINT ( 'NONE',  ( 10.96256856629999987, -5.431962315094999383, -4.905456409002999507 ) ) ;
#51443=CARTESIAN_POINT ( 'NONE',  ( 11.09999999999999964, -4.000000000000000000, 7.500000000000000000 ) ) ;
#51448=CARTESIAN_POINT ( 'NONE',  ( 10.24478558459999888, -5.265199116477000452, 8.959495174640998982 ) ) ;
#51461=DIRECTION ( 'NONE',  ( 0.000000000000000000, -0.2461538461537955691, -0.9692307692307821076 ) ) ;
#51462=AXIS2_PLACEMENT_3D ( 'NONE', #58177, #69006, #15865 ) ;
#51474=CARTESIAN_POINT ( 'NONE',  ( 10.77962878203999963, -2.397503436487000261, 7.755423856053000442 ) ) ;
#51476=CARTESIAN_POINT ( 'NONE',  ( 10.91080643070914213, -2.803404389956826392, -6.850777194059048725 ) ) ;
#51477=CARTESIAN_POINT ( 'NONE',  ( 9.587239738464759853, -5.286462772564067158, -7.027016876574450954 ) ) ;
#51486=CARTESIAN_POINT ( 'NONE',  ( 8.288959924527002698, -3.489898988435000238, -6.767656065023998302 ) ) ;
#51488=CIRCLE ( 'NONE', #21343, 0.8000000000000000444 ) ;
#51490=CARTESIAN_POINT ( 'NONE',  ( 9.570737326637999587, -4.261100936929000049, -5.979198511086000423 ) ) ;
#51492=CARTESIAN_POINT ( 'NONE',  ( 9.725191424783300675, -2.649754699899359522, 7.500009801425228773 ) ) ;
#51493=CARTESIAN_POINT ( 'NONE',  ( 8.679055905797000037, -2.899999999999999911, 6.571291218949999902 ) ) ;
#51500=CARTESIAN_POINT ( 'NONE',  ( 9.281707361444031079, -3.320047962278884768, -8.679668831483224878 ) ) ;
#51508=DIRECTION ( 'NONE',  ( 0.000000000000000000, 0.8648648648648720183, 0.5020047465136825426 ) ) ;
#51524=CARTESIAN_POINT ( 'NONE',  ( 10.90000000000000036, -8.091320520030999219, -7.077643127633000297 ) ) ;
#51525=EDGE_CURVE ( 'NONE', #48366, #23094, #37617, .T. ) ;
#51529=DIRECTION ( 'NONE',  ( 0.8843050095428980351, 0.1786785984225995050, -0.4313682980505990638 ) ) ;
#51541=CARTESIAN_POINT ( 'NONE',  ( 7.350695902300781626, -3.999976678040469746, 6.116819565496747657 ) ) ;
#51547=CARTESIAN_POINT ( 'NONE',  ( 8.507487536397000838, -5.082459883441999615, -6.579846171250996356 ) ) ;
#51550=CARTESIAN_POINT ( 'NONE',  ( 10.49684650188000035, -3.093163888438999809, -5.046887178931999784 ) ) ;
#51551=CARTESIAN_POINT ( 'NONE',  ( 9.326385834542001874, -4.867164667115999599, -6.095483598963999938 ) ) ;
#51554=CARTESIAN_POINT ( 'NONE',  ( 11.04426809015000011, -5.244714960646999380, 5.175279275819000269 ) ) ;
#51556=CARTESIAN_POINT ( 'NONE',  ( 7.780759508074995168, -4.599947829706001912, 6.384407252255998699 ) ) ;
#51579=CARTESIAN_POINT ( 'NONE',  ( 10.14750362918999826, -2.602959084636999876, 6.738575912023000214 ) ) ;
#51582=CARTESIAN_POINT ( 'NONE',  ( 8.625066940379999991, -3.117370956513999758, 8.662188901935000018 ) ) ;
#51583=AXIS2_PLACEMENT_3D ( 'NONE', #64676, #52826, #43719 ) ;
#51590=CARTESIAN_POINT ( 'NONE',  ( 8.167796732633897605, -2.954779252209375873, 6.459714628853201468 ) ) ;
#51592=CARTESIAN_POINT ( 'NONE',  ( 11.08492081570999943, -3.668392767032000013, 5.558160538745999801 ) ) ;
#51595=CARTESIAN_POINT ( 'NONE',  ( 10.68375832677999959, -4.547311397465000127, -8.749131152219000285 ) ) ;
#51601=CARTESIAN_POINT ( 'NONE',  ( 10.43314899746000002, -5.167567567567999731, 6.822293592207000934 ) ) ;
#51609=CARTESIAN_POINT ( 'NONE',  ( 8.079287380335998137, -4.920039154826996608, 6.237958006931995314 ) ) ;
#51616=CARTESIAN_POINT ( 'NONE',  ( 10.60198654464000079, -2.164987663130000239, -7.764523632348000248 ) ) ;
#51638=CARTESIAN_POINT ( 'NONE',  ( 7.743183059623000020, -2.735207418315000361, 6.771977475428999860 ) ) ;
#51643=B_SPLINE_CURVE_WITH_KNOTS ( 'NONE', 3,
 ( #17195, #57020, #45847, #35703 ),
 .UNSPECIFIED., .F., .F.,
 ( 4, 4 ),
 ( 0.000000000000000000, 1.000000000000000000 ),
 .UNSPECIFIED. ) ;
#51652=CARTESIAN_POINT ( 'NONE',  ( 10.63462194421999918, -5.668721490782999695, 6.527259573254000635 ) ) ;
#51658=CARTESIAN_POINT ( 'NONE',  ( 8.219916112706140865, -5.679804218022393769, 7.950509028919302779 ) ) ;
#51664=VERTEX_POINT ( 'NONE', #6840 ) ;
#51667=CARTESIAN_POINT ( 'NONE',  ( 9.888906509039999904, -2.890602650755999647, -6.682694598879999504 ) ) ;
#51668=PLANE ( 'NONE',  #63894 ) ;
#51677=CARTESIAN_POINT ( 'NONE',  ( 8.417495559623999313, -2.029110377978999846, 7.726994002375999315 ) ) ;
#51682=CARTESIAN_POINT ( 'NONE',  ( 10.37239314679000124, -3.992345679293999972, -5.977234595428000397 ) ) ;
#51691=ADVANCED_FACE ( 'NONE', ( #56466 ), #4341, .T. ) ;
#51703=CARTESIAN_POINT ( 'NONE',  ( 10.18795867446420722, -4.829522773136136315, -8.579479308275068661 ) ) ;
#51704=B_SPLINE_CURVE_WITH_KNOTS ( 'NONE', 3,
 ( #28426, #55333, #33323, #39252, #49049 ),
 .UNSPECIFIED., .F., .F.,
 ( 4, 1, 4 ),
 ( 0.000000000000000000, 0.5000000000000000000, 1.000000000000000000 ),
 .UNSPECIFIED. ) ;
#51705=ORIENTED_EDGE ( 'NONE', *, *, #65698, .T. ) ;
#51738=CYLINDRICAL_SURFACE ( 'NONE', #19873, 0.4999999999999998335 ) ;
#51739=CARTESIAN_POINT ( 'NONE',  ( 8.116918146793999256, -5.773185758034999893, 7.141496747382000798 ) ) ;
#51745=CARTESIAN_POINT ( 'NONE',  ( 7.576913711449058120, -4.062718167131674996, 5.761938145506621645 ) ) ;
#51751=CARTESIAN_POINT ( 'NONE',  ( 10.32671362595031006, -4.830823584655211889, 4.959879567452830429 ) ) ;
#51763=VERTEX_POINT ( 'NONE', #40721 ) ;
#51772=CARTESIAN_POINT ( 'NONE',  ( 9.980430903642000473, -4.047223565251000466, 9.090364706348999846 ) ) ;
#51774=CARTESIAN_POINT ( 'NONE',  ( 10.20917469696999902, -3.334764780022000163, -5.769478358936999562 ) ) ;
#51782=CARTESIAN_POINT ( 'NONE',  ( 10.31746213571000048, -5.100000000000000533, 6.571291218949999902 ) ) ;
#51787=DIRECTION ( 'NONE',  ( 1.000000000000000000, 0.000000000000000000, 0.000000000000000000 ) ) ;
#51801=CARTESIAN_POINT ( 'NONE',  ( 7.307500000000000107, -0.2999999999999999889, 3.149999999999999911 ) ) ;
#51812=CARTESIAN_POINT ( 'NONE',  ( 11.09999999999999964, -4.000000000000000000, 7.500000000000000000 ) ) ;
#51815=CARTESIAN_POINT ( 'NONE',  ( 7.000000000000000000, 0.000000000000000000, 0.000000000000000000 ) ) ;
#51825=CARTESIAN_POINT ( 'NONE',  ( 10.95279684016000132, -2.845132595845000001, 5.182798816160999245 ) ) ;
#51832=CARTESIAN_POINT ( 'NONE',  ( 11.08729972629000038, -2.258669075224000178, -7.034582301298999418 ) ) ;
#51833=CARTESIAN_POINT ( 'NONE',  ( 8.965984360231558981, -5.205022649008422597, 8.206117015345352428 ) ) ;
#51842=CARTESIAN_POINT ( 'NONE',  ( 8.497376085219370268, -4.829144488946368163, 8.579037299257766591 ) ) ;
#51859=EDGE_CURVE ( 'NONE', #66543, #17007, #58543, .T. ) ;
#51875=CARTESIAN_POINT ( 'NONE',  ( 9.870877370727999534, -2.904359058094999835, -8.563874348197000330 ) ) ;
#51880=CARTESIAN_POINT ( 'NONE',  ( 8.296584958550784705, -4.202842144468573515, 6.085974855212024082 ) ) ;
#51892=CARTESIAN_POINT ( 'NONE',  ( 9.839739029020998728, -5.130141620686999637, -6.219151643305999677 ) ) ;
#51895=CARTESIAN_POINT ( 'NONE',  ( 11.13353229228999908, -5.335146187777999316, 5.116023372597999774 ) ) ;
#51905=ADVANCED_FACE ( 'NONE', ( #67973 ), #58486, .T. ) ;
#51908=DIRECTION ( 'NONE',  ( 0.000000000000000000, -1.000000000000000000, 0.000000000000000000 ) ) ;
#51919=ORIENTED_EDGE ( 'NONE', *, *, #27187, .F. ) ;
#51920=CARTESIAN_POINT ( 'NONE',  ( 10.42595817177000050, -5.042180160032999403, 8.702227297563000619 ) ) ;
#51922=CARTESIAN_POINT ( 'NONE',  ( 7.550000000000000711, -4.000000000000000000, 8.849999999999999645 ) ) ;
#51923=CARTESIAN_POINT ( 'NONE',  ( 8.946004440379999423, -5.458705123429999695, 7.456451825584000659 ) ) ;
#51930=CARTESIAN_POINT ( 'NONE',  ( 11.09999999999999964, -5.350000000000000533, 7.500000000000000000 ) ) ;
#51933=CARTESIAN_POINT ( 'NONE',  ( 10.02990552045999983, -2.506467134554999809, 6.215414506835998942 ) ) ;
#51937=CARTESIAN_POINT ( 'NONE',  ( 9.858853446676000942, -2.668079545448999834, -7.206971019603000350 ) ) ;
#51938=CARTESIAN_POINT ( 'NONE',  ( 10.86123236735334530, -5.100000000000000533, -6.348362623949493688 ) ) ;
#51948=CARTESIAN_POINT ( 'NONE',  ( 8.434756776051003158, -5.098765216145000778, 6.624660916390000764 ) ) ;
#51949=ORIENTED_EDGE ( 'NONE', *, *, #19086, .F. ) ;
#51954=CARTESIAN_POINT ( 'NONE',  ( 10.28773706650000008, -5.077599250153999932, -5.991350640809000261 ) ) ;
#51955=EDGE_CURVE ( 'NONE', #51763, #64065, #50801, .T. ) ;
#51958=VERTEX_POINT ( 'NONE', #45893 ) ;
#51971=B_SPLINE_CURVE_WITH_KNOTS ( 'NONE', 3,
 ( #38170, #31915, #43779, #21746 ),
 .UNSPECIFIED., .F., .F.,
 ( 4, 4 ),
 ( 0.000000000000000000, 1.000000000000000000 ),
 .UNSPECIFIED. ) ;
#51974=ORIENTED_EDGE ( 'NONE', *, *, #55444, .T. ) ;
#51975=CARTESIAN_POINT ( 'NONE',  ( 9.117519353207999444, -4.954907757874000396, 8.825780921426000347 ) ) ;
#51983=EDGE_CURVE ( 'NONE', #50721, #44355, #16808, .T. ) ;
#51987=DIRECTION ( 'NONE',  ( -3.936133611084978447E-08, 0.7071067676227968946, -0.7071067947502968076 ) ) ;
#51991=ADVANCED_FACE ( 'NONE', ( #14768, #36085 ), #45561, .T. ) ;
#51994=CARTESIAN_POINT ( 'NONE',  ( 8.128451618207334306, -5.085822230759275087, 6.140894674361986993 ) ) ;
#51995=AXIS2_PLACEMENT_3D ( 'NONE', #12233, #48947, #54180 ) ;
#51997=ORIENTED_EDGE ( 'NONE', *, *, #15801, .T. ) ;
#51998=CARTESIAN_POINT ( 'NONE',  ( 9.299999999999998934, -4.537600397704999899, 9.154563893594000135 ) ) ;
#52017=VERTEX_POINT ( 'NONE', #61973 ) ;
#52021=CARTESIAN_POINT ( 'NONE',  ( 9.991527686541001430, -4.805948463426999773, -8.932428271061001013 ) ) ;
#52022=LINE ( 'NONE', #4123, #43325 ) ;
#52055=CARTESIAN_POINT ( 'NONE',  ( 9.218906055667105193, -2.654017316073122856, 7.603682184084918028 ) ) ;
#52065=B_SPLINE_CURVE_WITH_KNOTS ( 'NONE', 3,
 ( #26384, #27071, #38236, #16907 ),
 .UNSPECIFIED., .F., .F.,
 ( 4, 4 ),
 ( 0.000000000000000000, 1.000000000000000000 ),
 .UNSPECIFIED. ) ;
#52071=DIRECTION ( 'NONE',  ( 1.000000000000000000, 0.000000000000000000, 0.000000000000000000 ) ) ;
#52076=DIRECTION ( 'NONE',  ( 0.000000000000000000, 0.8648648648648720183, 0.5020047465136825426 ) ) ;
#52077=CARTESIAN_POINT ( 'NONE',  ( 9.234504440379000201, -5.964711531933999389, 7.776478361891000723 ) ) ;
#52084=CARTESIAN_POINT ( 'NONE',  ( 7.645530094557493328, -5.359336832227764802, 6.415087437494591427 ) ) ;
#52097=CARTESIAN_POINT ( 'NONE',  ( 9.975298369746534277, -5.350379160513648813, 7.499985214262776978 ) ) ;
#52102=CARTESIAN_POINT ( 'NONE',  ( 8.709622771139999386, -5.146410603519000482, -6.783155613812000162 ) ) ;
#52112=CARTESIAN_POINT ( 'NONE',  ( 9.646285452541999206, -2.591464128784999765, 6.760053199270999791 ) ) ;
#52119=CARTESIAN_POINT ( 'NONE',  ( 11.12486982654999856, -6.581651479209999600, -5.643180424050000532 ) ) ;
#52125=CARTESIAN_POINT ( 'NONE',  ( 9.465112865370999273, -2.290047720994000002, 6.601709978349000529 ) ) ;
#52126=VERTEX_POINT ( 'NONE', #47615 ) ;
#52129=CARTESIAN_POINT ( 'NONE',  ( 9.246653663635285625, -2.697134473482441841, 7.146693063513369637 ) ) ;
#52133=CARTESIAN_POINT ( 'NONE',  ( 10.57314899745999881, -5.167567567567999731, -6.822293592207000934 ) ) ;
#52134=CARTESIAN_POINT ( 'NONE',  ( 9.538434317036999843, -5.620900626097999897, 7.423100105894999245 ) ) ;
#52139=LINE ( 'NONE', #24892, #25933 ) ;
#52141=CARTESIAN_POINT ( 'NONE',  ( 10.11094409420000062, -5.100000000000000533, -6.571291218949999902 ) ) ;
#52163=ORIENTED_EDGE ( 'NONE', *, *, #41655, .F. ) ;
#52170=CARTESIAN_POINT ( 'NONE',  ( 10.49914019022526901, -4.925950642208848151, -4.998102050154486165 ) ) ;
#52178=CARTESIAN_POINT ( 'NONE',  ( 10.72129555961999792, -4.673507771948999689, -5.778404201896999659 ) ) ;
#52182=CARTESIAN_POINT ( 'NONE',  ( 8.287602349183067929, -2.892084057926692431, 6.689538224764139507 ) ) ;
#52184=EDGE_CURVE ( 'NONE', #5164, #1057, #63488, .T. ) ;
#52199=VERTEX_POINT ( 'NONE', #58502 ) ;
#52205=ORIENTED_EDGE ( 'NONE', *, *, #55168, .T. ) ;
#52215=CARTESIAN_POINT ( 'NONE',  ( 8.039443364739078390, -4.176885327615397436, 8.849067469250744722 ) ) ;
#52220=CARTESIAN_POINT ( 'NONE',  ( 10.65650106607000147, -5.448187878199999723, -7.015213573792999036 ) ) ;
#52221=ADVANCED_FACE ( 'NONE', ( #26354 ), #36845, .T. ) ;
#52223=VERTEX_POINT ( 'NONE', #26702 ) ;
#52233=CARTESIAN_POINT ( 'NONE',  ( 7.782975328289005290, -3.196931270636999667, 6.293200827887002191 ) ) ;
#52234=ORIENTED_EDGE ( 'NONE', *, *, #29481, .T. ) ;
#52236=CARTESIAN_POINT ( 'NONE',  ( 8.149001627428001271, -3.121156835630000348, 6.130053226229998486 ) ) ;
#52247=CARTESIAN_POINT ( 'NONE',  ( 8.244326721667006197, -4.955553483043997787, 6.175174249266997428 ) ) ;
#52261=CARTESIAN_POINT ( 'NONE',  ( 9.214598350284001427, -2.899999999999999911, -6.571291218949999902 ) ) ;
#52265=DIRECTION ( 'NONE',  ( -0.7071067811865713315, 0.6115518083850753905, -0.3549709645321856843 ) ) ;
#52269=CARTESIAN_POINT ( 'NONE',  ( 9.332935524889000689, -5.100347267927999972, 8.693464469215999912 ) ) ;
#52273=CARTESIAN_POINT ( 'NONE',  ( 8.122956853208000538, -3.566638198986999964, 5.743608852252999775 ) ) ;
#52275=ORIENTED_EDGE ( 'NONE', *, *, #39639, .T. ) ;
#52281=CARTESIAN_POINT ( 'NONE',  ( 8.155831921393041029, -3.033675026350174608, 6.347534157511051767 ) ) ;
#52283=FACE_OUTER_BOUND ( 'NONE', #37907, .T. ) ;
#52287=CARTESIAN_POINT ( 'NONE',  ( 10.97075054419999951, -2.648517896406999750, -6.788869136079999755 ) ) ;
#52311=B_SPLINE_CURVE_WITH_KNOTS ( 'NONE', 3,
 ( #50238, #56860, #67330, #2342 ),
 .UNSPECIFIED., .F., .F.,
 ( 4, 4 ),
 ( 0.000000000000000000, 1.000000000000000000 ),
 .UNSPECIFIED. ) ;
#52329=CARTESIAN_POINT ( 'NONE',  ( 9.250897313459001126, -4.135077143711000325, 9.175520401071999288 ) ) ;
#52333=AXIS2_PLACEMENT_3D ( 'NONE', #9381, #19889, #57625 ) ;
#52334=EDGE_CURVE ( 'NONE', #34244, #28326, #65685, .T. ) ;
#52347=CARTESIAN_POINT ( 'NONE',  ( 8.219858292491261764, -5.680146748682262547, 7.949319526458594964 ) ) ;
#52356=ORIENTED_EDGE ( 'NONE', *, *, #2692, .F. ) ;
#52357=CARTESIAN_POINT ( 'NONE',  ( 9.580894592352999339, -5.371875912611999482, -7.370590366721999409 ) ) ;
#52358=DIRECTION ( 'NONE',  ( 0.4384236320214023319, 0.000000000000000000, 0.8987684456439056779 ) ) ;
#52367=CARTESIAN_POINT ( 'NONE',  ( 9.149956853208999874, -4.175914961544999748, 5.699510287082000026 ) ) ;
#52390=EDGE_CURVE ( 'NONE', #63466, #16664, #118, .T. ) ;
#52393=EDGE_CURVE ( 'NONE', #51763, #64582, #6045, .T. ) ;
#52406=CARTESIAN_POINT ( 'NONE',  ( 9.180279526884143948, -2.858231322599188662, 8.226333960650446642 ) ) ;
#52420=DIRECTION ( 'NONE',  ( 0.000000000000000000, 0.000000000000000000, -1.000000000000000000 ) ) ;
#52425=CARTESIAN_POINT ( 'NONE',  ( 11.09999999999999964, -5.538898460221000519, 7.685179721164000277 ) ) ;
#52426=CARTESIAN_POINT ( 'NONE',  ( 7.641206853206999661, -4.524489047957000132, 9.047757046927999980 ) ) ;
#52432=CARTESIAN_POINT ( 'NONE',  ( 7.612036250381388314, -4.782439721774751185, 5.946226314582684580 ) ) ;
#52436=LINE ( 'NONE', #4532, #37758 ) ;
#52442=ORIENTED_EDGE ( 'NONE', *, *, #49706, .F. ) ;
#52446=CARTESIAN_POINT ( 'NONE',  ( 10.97884673417783041, -5.207210053465712640, 6.723535013421952478 ) ) ;
#52450=ORIENTED_EDGE ( 'NONE', *, *, #9730, .F. ) ;
#52455=CARTESIAN_POINT ( 'NONE',  ( 10.74708275169999894, -5.262360166711999909, 4.827842598592000378 ) ) ;
#52460=CARTESIAN_POINT ( 'NONE',  ( 10.07771285905000092, -4.622037501707999319, 5.671359981946999973 ) ) ;
#52473=CARTESIAN_POINT ( 'NONE',  ( 11.09648096125000016, -3.099777420064000033, 6.097103007060000301 ) ) ;
#52482=CARTESIAN_POINT ( 'NONE',  ( 9.104016254283999743, -5.045864843302999780, 8.527867871227000407 ) ) ;
#52485=B_SPLINE_SURFACE_WITH_KNOTS ( 'NONE', 3, 3, ( 
 ( #3203, #24873, #9465, #21255 ),
 ( #63892, #30806, #46201, #51440 ),
 ( #10761, #51101, #40952, #62274 ),
 ( #32104, #18943, #46549, #67852 ),
 ( #19976, #53421, #41297, #45857 ),
 ( #62606, #40271, #61588, #35034 ),
 ( #13704, #14729, #56348, #3536 ),
 ( #8454, #8794, #14392, #67166 ),
 ( #52119, #42584, #36044, #19279 ) ),
 .UNSPECIFIED., .F., .F., .F.,
 ( 4, 1, 1, 1, 1, 1, 4 ),
 ( 4, 4 ),
 ( -0.01830387170766999833, 0.000000000000000000, 0.2500000000000000000, 0.5000000000000000000, 0.7500000000000000000, 1.000000000000000000, 1.018541916426999983 ),
 ( -0.2206046696922999983, 1.220604669692000099 ),
 .UNSPECIFIED. ) ;
#52488=DIRECTION ( 'NONE',  ( 0.000000000000000000, 0.000000000000000000, -1.000000000000000000 ) ) ;
#52490=CARTESIAN_POINT ( 'NONE',  ( 9.531901401888999814, -3.025808284870999731, -9.100010361367001366 ) ) ;
#52503=CARTESIAN_POINT ( 'NONE',  ( 10.68904248846000016, -2.568964727443000307, 7.728094434513999467 ) ) ;
#52509=EDGE_LOOP ( 'NONE', ( #27178, #51215, #13805, #1136 ) ) ;
#52512=CARTESIAN_POINT ( 'NONE',  ( 9.731599613776074520, -3.320020895154290663, -8.679702885126729939 ) ) ;
#52518=B_SPLINE_CURVE_WITH_KNOTS ( 'NONE', 3,
 ( #61461, #35245, #8666, #66353 ),
 .UNSPECIFIED., .F., .F.,
 ( 4, 4 ),
 ( 0.000000000000000000, 1.000000000000000000 ),
 .UNSPECIFIED. ) ;
#52520=CARTESIAN_POINT ( 'NONE',  ( 9.531901401888999814, -3.025808284870999731, -9.100010361367001366 ) ) ;
#52521=LINE ( 'NONE', #15123, #58365 ) ;
#52526=CARTESIAN_POINT ( 'NONE',  ( 9.216851002545999094, -2.832432432432000269, 6.822293592207000934 ) ) ;
#52527=CARTESIAN_POINT ( 'NONE',  ( 11.00000000000000000, -2.799999999999999822, -5.864181267619000160 ) ) ;
#52554=EDGE_CURVE ( 'NONE', #63466, #36772, #39234, .T. ) ;
#52562=AXIS2_PLACEMENT_3D ( 'NONE', #6985, #23062, #11191 ) ;
#52565=CARTESIAN_POINT ( 'NONE',  ( 10.49937632700000023, -2.985311165300999825, -6.358653174814000053 ) ) ;
#52573=CYLINDRICAL_SURFACE ( 'NONE', #5347, 0.5000000000000002220 ) ;
#52578=CARTESIAN_POINT ( 'NONE',  ( 7.555544676565999040, -2.930005555947998275, 6.552699291324001862 ) ) ;
#52582=CARTESIAN_POINT ( 'NONE',  ( 7.540373275913000661, -2.929987504175003199, 6.557984262489997995 ) ) ;
#52585=CARTESIAN_POINT ( 'NONE',  ( 9.595487457706001422, -3.928425191288000384, 5.531324308465000783 ) ) ;
#52589=CARTESIAN_POINT ( 'NONE',  ( 8.057875016312998184, -4.641725571029997610, 6.225038937488997171 ) ) ;
#52600=CARTESIAN_POINT ( 'NONE',  ( 8.646755198799242592, -2.839843517792559613, -6.809530303469401247 ) ) ;
#52610=ORIENTED_EDGE ( 'NONE', *, *, #58253, .T. ) ;
#52611=CARTESIAN_POINT ( 'NONE',  ( 10.74600376124999990, -5.242711034443999552, 8.978690688221998784 ) ) ;
#52614=CARTESIAN_POINT ( 'NONE',  ( 7.866206853207000194, -4.580607464247000493, 9.213361409141999303 ) ) ;
#52624=CARTESIAN_POINT ( 'NONE',  ( 10.12549839661999940, -5.788806995403000144, 7.335561828691000485 ) ) ;
#52628=CARTESIAN_POINT ( 'NONE',  ( 9.688891943909794691, -2.651205815582408754, 7.263338752445791080 ) ) ;
#52638=CARTESIAN_POINT ( 'NONE',  ( 11.07345355053000091, -3.998673159585000025, 8.920828114954002075 ) ) ;
#52643=ORIENTED_EDGE ( 'NONE', *, *, #47435, .F. ) ;
#52651=CARTESIAN_POINT ( 'NONE',  ( 9.442390274284505836, -4.489521974667288973, -9.208960678577202685 ) ) ;
#52653=ORIENTED_EDGE ( 'NONE', *, *, #63158, .F. ) ;
#52658=CARTESIAN_POINT ( 'NONE',  ( 8.822980646795000936, -2.678334737187000325, 8.735278777293000729 ) ) ;
#52668=DIRECTION ( 'NONE',  ( -1.000000000000000000, 0.000000000000000000, -2.523982353566999962E-12 ) ) ;
#52671=CARTESIAN_POINT ( 'NONE',  ( 7.390495559621999888, -2.216884807317999861, 8.370075800106999253 ) ) ;
#52689=CARTESIAN_POINT ( 'NONE',  ( 8.234515473452628243, -5.574618550199808453, 8.239559727061074312 ) ) ;
#52690=CARTESIAN_POINT ( 'NONE',  ( 11.03775575519999919, -8.050335494570999728, 6.914609630061999468 ) ) ;
#52699=EDGE_CURVE ( 'NONE', #15904, #17545, #61764, .T. ) ;
#52700=EDGE_CURVE ( 'NONE', #23313, #53841, #12954, .T. ) ;
#52701=CARTESIAN_POINT ( 'NONE',  ( 9.492891187585001944, -4.474581801608000120, -6.279517683005999551 ) ) ;
#52711=VECTOR ( 'NONE', #46275, 1000.000000000000000 ) ;
#52712=CARTESIAN_POINT ( 'NONE',  ( 8.160745559622998968, -5.944572422272999646, 7.106845737860000511 ) ) ;
#52717=CARTESIAN_POINT ( 'NONE',  ( 5.700000000000000178, -1.300000000000000044, -10.66294468575716969 ) ) ;
#52720=B_SPLINE_CURVE_WITH_KNOTS ( 'NONE', 3,
 ( #7846, #13782, #17995, #29181, #55394 ),
 .UNSPECIFIED., .F., .F.,
 ( 4, 1, 4 ),
 ( 0.000000000000000000, 0.5000000000000000000, 1.000000000000000000 ),
 .UNSPECIFIED. ) ;
#52722=DIRECTION ( 'NONE',  ( 0.000000000000000000, 1.000000000000000000, 0.000000000000000000 ) ) ;
#52724=VERTEX_POINT ( 'NONE', #35983 ) ;
#52733=CARTESIAN_POINT ( 'NONE',  ( 10.52663358771999924, -4.933730002636999679, -6.506004698255999585 ) ) ;
#52738=EDGE_LOOP ( 'NONE', ( #41470, #44647, #61421, #62806, #55492 ) ) ;
#52739=CARTESIAN_POINT ( 'NONE',  ( 10.90157398350000051, -5.294378252237999405, -4.903209430186000084 ) ) ;
#52740=ORIENTED_EDGE ( 'NONE', *, *, #47519, .T. ) ;
#52752=CARTESIAN_POINT ( 'NONE',  ( 9.148111568353531453, -3.223588768401370874, 8.615646755131677992 ) ) ;
#52762=EDGE_LOOP ( 'NONE', ( #23330, #67309, #16613, #68024 ) ) ;
#52770=ORIENTED_EDGE ( 'NONE', *, *, #51983, .T. ) ;
#52775=CARTESIAN_POINT ( 'NONE',  ( 8.668206853210000062, -3.979464503892999439, 9.134080454305001595 ) ) ;
#52780=CARTESIAN_POINT ( 'NONE',  ( 7.608564460558524090, -4.712693663111584996, 5.912577119032927264 ) ) ;
#52791=EDGE_CURVE ( 'NONE', #39266, #58368, #65968, .T. ) ;
#52805=VERTEX_POINT ( 'NONE', #1332 ) ;
#52811=CARTESIAN_POINT ( 'NONE',  ( 10.00122642709000154, -2.274091010763000131, 7.851325450887000734 ) ) ;
#52813=LINE ( 'NONE', #41632, #17377 ) ;
#52825=CARTESIAN_POINT ( 'NONE',  ( 9.254609482145166766, -2.734579386017075286, 7.018993749219657019 ) ) ;
#52826=DIRECTION ( 'NONE',  ( -1.000000000000000000, 0.000000000000000000, 0.000000000000000000 ) ) ;
#52827=ORIENTED_EDGE ( 'NONE', *, *, #38801, .F. ) ;
#52831=CARTESIAN_POINT ( 'NONE',  ( 9.724613486786999772, -2.928302463146000179, 8.718481221599999387 ) ) ;
#52849=VERTEX_POINT ( 'NONE', #16712 ) ;
#52868=CARTESIAN_POINT ( 'NONE',  ( 10.90000000000000036, -2.832432432432000269, -6.822293592207000934 ) ) ;
#52874=EDGE_CURVE ( 'NONE', #28855, #29023, #17058, .T. ) ;
#52884=ORIENTED_EDGE ( 'NONE', *, *, #46056, .T. ) ;
#52890=CARTESIAN_POINT ( 'NONE',  ( 7.000000000000000000, -7.356634010774431687, -3.356634010774432575 ) ) ;
#52904=B_SPLINE_SURFACE_WITH_KNOTS ( 'NONE', 3, 3, ( 
 ( #33507, #45032, #2718, #12521, #60756, #17418, #39784, #50616, #28254, #43996, #1684, #33852, #28611, #13226, #12871, #1334, #7620, #2375, #24042, #55166, #6922, #12177, #49227, #7271, #39091, #28966, #22651, #7969, #34199, #50271, #29305, #45377, #60416, #13567, #23698 ),
 ( #49925, #23354, #18117, #2036, #18808, #40135, #66337, #66684, #23001, #34887, #65303, #44696, #18461, #38744, #65991, #61106, #56203, #39435, #44350, #34553, #8311, #54823, #60073, #55863, #65649, #61449, #49574, #17773, #35906, #41496, #62128, #24732, #36598, #52329, #19831 ),
 ( #62807, #67704, #30667, #8988, #3735, #50958, #63147, #4424, #9669, #14926, #19137, #67362, #51299, #3395, #46059, #19485, #25762, #8651, #40459, #46749, #61786, #45718, #15274, #36249, #40806, #35233, #68054, #47092, #57924, #24387, #68392, #20168, #51975, #20512, #14248 ),
 ( #13905, #57569, #56545, #67027, #29657, #31020, #35575, #29999, #41838, #3056, #56891, #30330, #51638, #25069, #4077, #46403, #41162, #62468, #14588, #57221, #25415, #9323, #53366, #47433, #16297, #48119, #27486, #10705, #20859, #920, #223, #21884, #32050, #21200, #21540 ) ),
 .UNSPECIFIED., .F., .F., .F.,
 ( 4, 4 ),
 ( 4, 1, 1, 1, 1, 1, 1, 1, 1, 1, 1, 1, 1, 1, 1, 1, 1, 1, 1, 1, 1, 1, 1, 1, 1, 1, 1, 1, 1, 1, 1, 1, 4 ),
 ( -0.1039086239011999951, 1.103908623900999864 ),
 ( -0.02000000000000000042, 0.01250000000000000069, 0.04499999999999999833, 0.07749999999999999944, 0.1100000000000000006, 0.1424999999999999878, 0.1749999999999999889, 0.2074999999999999900, 0.2399999999999999911, 0.2725000000000000200, 0.3049999999999999933, 0.3375000000000000222, 0.3699999999999999956, 0.4025000000000000244, 0.4349999999999999978, 0.4675000000000000266, 0.5000000000000000000, 0.5324999999999999734, 0.5649999999999999467, 0.5975000000000000311, 0.6300000000000000044, 0.6624999999999999778, 0.6949999999999999512, 0.7275000000000000355, 0.7600000000000000089, 0.7924999999999999822, 0.8249999999999999556, 0.8575000000000000400, 0.8900000000000000133, 0.9224999999999999867, 0.9549999999999999600, 0.9875000000000000444, 1.020000000000000018 ),
 .UNSPECIFIED. ) ;
#52905=CARTESIAN_POINT ( 'NONE',  ( 8.447783767286816570, -5.285582108569009563, 7.027722483016056287 ) ) ;
#52906=CARTESIAN_POINT ( 'NONE',  ( 10.44608131895000191, -8.241816726637999579, -6.830402593584000925 ) ) ;
#52916=CARTESIAN_POINT ( 'NONE',  ( 10.40879003340999986, -3.093879171920000282, -6.480773124728999690 ) ) ;
#52921=DIRECTION ( 'NONE',  ( 1.000000000000000000, 0.000000000000000000, 0.000000000000000000 ) ) ;
#52927=CARTESIAN_POINT ( 'NONE',  ( 10.26106145044999884, -3.441494892447000353, 4.532186341712000299 ) ) ;
#52928=CARTESIAN_POINT ( 'NONE',  ( 7.790168786842999182, -2.923571394339999685, 6.474157094959999803 ) ) ;
#52932=CARTESIAN_POINT ( 'NONE',  ( 7.861945368778997079, -2.855203060631998024, 6.787771340568003353 ) ) ;
#52933=CARTESIAN_POINT ( 'NONE',  ( 9.800903104272999045, -2.772050158355999994, -8.125211791007998841 ) ) ;
#52935=CARTESIAN_POINT ( 'NONE',  ( 9.905786073958001481, -2.698967003257000119, 8.979227319929000473 ) ) ;
#52936=CARTESIAN_POINT ( 'NONE',  ( 10.86209373942999967, -5.065348428249999202, 5.178139088298999937 ) ) ;
#52949=DIRECTION ( 'NONE',  ( -1.000000000000000000, 0.000000000000000000, 0.000000000000000000 ) ) ;
#52967=CARTESIAN_POINT ( 'NONE',  ( 8.508081853209001011, -2.202816532622999812, 7.706987678916999762 ) ) ;
#52969=ORIENTED_EDGE ( 'NONE', *, *, #42796, .T. ) ;
#52975=CARTESIAN_POINT ( 'NONE',  ( 9.724613486786999772, -2.928302463146000179, 8.718481221599999387 ) ) ;
#52981=CYLINDRICAL_SURFACE ( 'NONE', #67154, 10.75000000000000000 ) ;
#52982=ORIENTED_EDGE ( 'NONE', *, *, #61176, .F. ) ;
#52985=EDGE_CURVE ( 'NONE', #46630, #9447, #13223, .T. ) ;
#53003=CARTESIAN_POINT ( 'NONE',  ( 9.258050732556000639, -4.895927245463000510, -6.008721945297999412 ) ) ;
#53009=CARTESIAN_POINT ( 'NONE',  ( 7.127706853208000126, -4.698358408974000255, 8.789434435623999065 ) ) ;
#53011=CARTESIAN_POINT ( 'NONE',  ( 10.27164068752446902, -2.873222873891751572, 6.752018918739129738 ) ) ;
#53012=AXIS2_PLACEMENT_3D ( 'NONE', #28347, #11909, #22740 ) ;
#53021=CARTESIAN_POINT ( 'NONE',  ( 9.304730646793998972, -5.284133759825000887, 6.489273023403000273 ) ) ;
#53025=ORIENTED_EDGE ( 'NONE', *, *, #16665, .F. ) ;
#53035=CARTESIAN_POINT ( 'NONE',  ( 7.121419741036552509, -3.646617224772007670, 8.816373456089998228 ) ) ;
#53038=CARTESIAN_POINT ( 'NONE',  ( 7.844724262280000637, -4.719412258162999585, 6.357657668295000342 ) ) ;
#53042=CARTESIAN_POINT ( 'NONE',  ( 8.414467752718078231, -2.422965004064780103, 8.233303954855905715 ) ) ;
#53045=DIRECTION ( 'NONE',  ( -0.7660444387781886189, 2.249698893085964329E-11, -0.6427876148596907147 ) ) ;
#53050=CARTESIAN_POINT ( 'NONE',  ( 7.800894438721999613, -3.218815632501999868, 6.398977300879999497 ) ) ;
#53051=CARTESIAN_POINT ( 'NONE',  ( 9.932908211424001266, -3.485164486501000081, -6.221839249167999242 ) ) ;
#53052=CARTESIAN_POINT ( 'NONE',  ( 9.733249152250484926, -4.120954265945523609, -8.873128867233456063 ) ) ;
#53055=CARTESIAN_POINT ( 'NONE',  ( 8.835539685685773748, -3.765107182069276526, 9.264007590920439128 ) ) ;
#53064=B_SPLINE_SURFACE_WITH_KNOTS ( 'NONE', 3, 3, ( 
 ( #30354, #3082, #57588, #35931 ),
 ( #9696, #40487, #8338, #50985 ),
 ( #24415, #31042, #35600, #25096 ),
 ( #3421, #62829, #2742, #34915 ),
 ( #3757, #36273, #13930, #24068 ),
 ( #24756, #19853, #41182, #19162 ),
 ( #41518, #67729, #45403, #46082 ),
 ( #56914, #66712, #19511, #40829 ),
 ( #56229, #62154, #14613, #30689 ),
 ( #57244, #61813, #14272, #67389 ),
 ( #18833, #13594, #9013, #9345 ) ),
 .UNSPECIFIED., .F., .F., .F.,
 ( 4, 1, 1, 1, 1, 1, 1, 1, 4 ),
 ( 4, 4 ),
 ( -0.01375657147579999878, 0.000000000000000000, 0.06250000000000000000, 0.1250000000000000000, 0.1875000000000000000, 0.2500000000000000000, 0.3125000000000000000, 0.3750000000000000000, 0.4325988669058000169 ),
 ( -0.1687363430499000116, 1.168634397496999933 ),
 .UNSPECIFIED. ) ;
#53068=CARTESIAN_POINT ( 'NONE',  ( 11.09999999999999964, -4.000000000000000000, -7.500000000000000000 ) ) ;
#53095=EDGE_CURVE ( 'NONE', #59582, #14991, #13209, .T. ) ;
#53098=CARTESIAN_POINT ( 'NONE',  ( 9.213774118050919171, -2.663711227152621763, 7.691546656787776826 ) ) ;
#53107=VECTOR ( 'NONE', #24178, 1000.000000000000114 ) ;
#53113=FACE_OUTER_BOUND ( 'NONE', #30065, .T. ) ;
#53118=CARTESIAN_POINT ( 'NONE',  ( 10.31457635473999979, -5.362146312020000138, 6.677778992223999843 ) ) ;
#53119=CARTESIAN_POINT ( 'NONE',  ( 7.614808059621999803, -3.326257819185999942, 8.794522506294001118 ) ) ;
#53120=VERTEX_POINT ( 'NONE', #10016 ) ;
#53123=CARTESIAN_POINT ( 'NONE',  ( 10.05882936267868466, -4.704418606475396558, 8.703716202581736283 ) ) ;
#53124=CARTESIAN_POINT ( 'NONE',  ( 10.11549555961999936, -2.489199523559999960, -6.434642413229999747 ) ) ;
#53125=CARTESIAN_POINT ( 'NONE',  ( 7.611706454504995278, -4.775798000191374904, 5.942893401888585281 ) ) ;
#53144=CARTESIAN_POINT ( 'NONE',  ( 5.499999999550999163, -0.5000000004493000416, -9.662944680110001627 ) ) ;
#53147=EDGE_CURVE ( 'NONE', #24689, #65709, #16552, .T. ) ;
#53152=CARTESIAN_POINT ( 'NONE',  ( 9.910640133503999749, -2.107273866476999657, 7.885282692430999774 ) ) ;
#53171=DIRECTION ( 'NONE',  ( 0.000000000000000000, -0.1333333333333049375, 0.9910712498212376209 ) ) ;
#53172=CARTESIAN_POINT ( 'NONE',  ( 10.97865453029000093, -5.273142482194999481, 7.958032781726000593 ) ) ;
#53179=B_SPLINE_CURVE_WITH_KNOTS ( 'NONE', 3,
 ( #51601, #24011, #3699, #25037 ),
 .UNSPECIFIED., .F., .F.,
 ( 4, 4 ),
 ( 0.000000000000000000, 0.1254754252289749794 ),
 .UNSPECIFIED. ) ;
#53180=CARTESIAN_POINT ( 'NONE',  ( 0.000000000000000000, -5.100000000000000533, -7.500000000000000000 ) ) ;
#53183=DIRECTION ( 'NONE',  ( 0.000000000000000000, -1.000000000000000000, 0.000000000000000000 ) ) ;
#53209=CARTESIAN_POINT ( 'NONE',  ( 9.267891187585000523, -4.645169647889000331, -5.840816811670999975 ) ) ;
#53210=CARTESIAN_POINT ( 'NONE',  ( 10.19122055961999962, -3.990707710465999813, -5.651373900265999950 ) ) ;
#53242=DIRECTION ( 'NONE',  ( 0.4384236320213994453, -0.6355252626312994924, 0.6355252626312996034 ) ) ;
#53250=CIRCLE ( 'NONE', #30954, 0.4999999999999995559 ) ;
#53254=CARTESIAN_POINT ( 'NONE',  ( 10.18512684885999953, -5.526147823900999789, -7.556025229989000280 ) ) ;
#53257=EDGE_LOOP ( 'NONE', ( #36566, #12845, #56500, #33440 ) ) ;
#53262=CARTESIAN_POINT ( 'NONE',  ( 8.616332382228000242, -2.832433105983000132, -6.822293595522999965 ) ) ;
#53264=EDGE_CURVE ( 'NONE', #11189, #57248, #14763, .T. ) ;
#53266=LINE ( 'NONE', #48020, #28860 ) ;
#53275=CARTESIAN_POINT ( 'NONE',  ( 7.602716214150000873, -2.929796814311000919, 6.536389039862005035 ) ) ;
#53279=CARTESIAN_POINT ( 'NONE',  ( 10.83668192271000130, -4.288535286065000562, 9.448729895547000268 ) ) ;
#53282=EDGE_CURVE ( 'NONE', #2520, #37807, #57546, .T. ) ;
#53293=DIRECTION ( 'NONE',  ( -1.644739578229999948E-10, -1.644740771478999934E-10, 1.000000000000000000 ) ) ;
#53299=DIRECTION ( 'NONE',  ( 0.9999999999977496890, 1.824801334886089481E-06, -1.081901619956053515E-06 ) ) ;
#53303=EDGE_LOOP ( 'NONE', ( #18850, #20538 ) ) ;
#53305=CARTESIAN_POINT ( 'NONE',  ( 10.33537187819000103, -5.153689638257000105, 8.830861236101000600 ) ) ;
#53308=CARTESIAN_POINT ( 'NONE',  ( 10.02052890782000105, -2.899999999999999911, 6.152188490330000370 ) ) ;
#53309=CARTESIAN_POINT ( 'NONE',  ( 7.545269353206999874, -2.302293129340000188, 6.875167727519000849 ) ) ;
#53314=B_SPLINE_CURVE_WITH_KNOTS ( 'NONE', 3,
 ( #28528, #59637, #49840, #1951, #48461, #569, #54389, #11733, #23272 ),
 .UNSPECIFIED., .F., .F.,
 ( 4, 1, 2, 2, 4 ),
 ( 0.000000000000000000, 0.2500000000000015543, 0.3750000000000009992, 0.5000000000000004441, 1.000000000000000000 ),
 .UNSPECIFIED. ) ;
#53318=CARTESIAN_POINT ( 'NONE',  ( 10.90000000536000080, -2.899999999941999640, -5.157071284930999866 ) ) ;
#53319=CARTESIAN_POINT ( 'NONE',  ( 7.100000000000000533, -5.349999999999999645, -7.500000000000000000 ) ) ;
#53321=CARTESIAN_POINT ( 'NONE',  ( 10.59344961228999971, -5.297755890367000120, 8.474197994416998725 ) ) ;
#53327=CARTESIAN_POINT ( 'NONE',  ( 11.14450444037999866, -5.035425715994000129, -8.381528062715000615 ) ) ;
#53354=CARTESIAN_POINT ( 'NONE',  ( 8.951355646795001064, -2.821866379289000193, 6.127148604720000336 ) ) ;
#53358=CARTESIAN_POINT ( 'NONE',  ( 7.100000000000000533, -5.349999999999999645, 7.500000000000000000 ) ) ;
#53365=CARTESIAN_POINT ( 'NONE',  ( 9.240543146793999796, -4.158911960977000000, 5.873536005760000123 ) ) ;
#53366=CARTESIAN_POINT ( 'NONE',  ( 8.385058059625000837, -4.977917894183000236, 6.416767031887000705 ) ) ;
#53379=CARTESIAN_POINT ( 'NONE',  ( 10.90437023801000116, -5.099522774867000230, 5.132565236215000049 ) ) ;
#53381=CARTESIAN_POINT ( 'NONE',  ( 7.954938716748859662, -4.949324164348111843, 6.428079711092701487 ) ) ;
#53384=CARTESIAN_POINT ( 'NONE',  ( 7.835819183419109102, -4.957498340680790427, 6.488970330265980024 ) ) ;
#53386=CARTESIAN_POINT ( 'NONE',  ( 8.418727353860353091, -2.386268681369533962, 8.150113380672019403 ) ) ;
#53391=B_SPLINE_CURVE_WITH_KNOTS ( 'NONE', 3,
 ( #41634, #46885, #35709, #30134, #9814 ),
 .UNSPECIFIED., .F., .F.,
 ( 4, 1, 4 ),
 ( 0.000000000000000000, 0.5000000000000000000, 1.000000000000000000 ),
 .UNSPECIFIED. ) ;
#53409=CARTESIAN_POINT ( 'NONE',  ( 11.09999999999999964, -5.350000000000000533, 7.500000000000000000 ) ) ;
#53412=CARTESIAN_POINT ( 'NONE',  ( 10.27427156480999848, -4.600000212792999754, 4.944156960788000710 ) ) ;
#53421=CARTESIAN_POINT ( 'NONE',  ( 11.07242469412000041, -6.093414471448999947, -5.195953259728000262 ) ) ;
#53454=CARTESIAN_POINT ( 'NONE',  ( 10.98768538770000092, -2.700669876604000041, 4.945210823433001224 ) ) ;
#53456=CARTESIAN_POINT ( 'NONE',  ( 9.266851002542999538, -2.832432432432000269, 6.822293592207000934 ) ) ;
#53466=CARTESIAN_POINT ( 'NONE',  ( 9.980430903642000473, -4.047223565251000466, 9.090364706348999846 ) ) ;
#53467=CARTESIAN_POINT ( 'NONE',  ( 7.037120559622001004, -4.623636604834999275, 8.651469651195000665 ) ) ;
#53471=CARTESIAN_POINT ( 'NONE',  ( 10.05463185321000097, -3.531218470783999752, -9.119231780812000920 ) ) ;
#53472=CARTESIAN_POINT ( 'NONE',  ( 7.790883244326107793, -4.713827597390799262, 9.089417837454107030 ) ) ;
#53473=CARTESIAN_POINT ( 'NONE',  ( 10.00137895011999944, -3.855365288061999962, 5.709482985498999241 ) ) ;
#53475=VERTEX_POINT ( 'NONE', #42369 ) ;
#53479=ORIENTED_EDGE ( 'NONE', *, *, #16800, .T. ) ;
#53488=DIRECTION ( 'NONE',  ( 0.000000000000000000, 1.000000000000000000, 0.000000000000000000 ) ) ;
#53490=EDGE_LOOP ( 'NONE', ( #20171, #14087, #64138, #57103, #49101, #20801, #66998, #47408, #31723, #66310 ) ) ;
#53498=CARTESIAN_POINT ( 'NONE',  ( 11.05935368890999904, -2.480241580537000168, 6.610077204591000566 ) ) ;
#53508=DIRECTION ( 'NONE',  ( 0.7660444431190069903, 0.000000000000000000, 0.6427876096865049460 ) ) ;
#53521=CARTESIAN_POINT ( 'NONE',  ( 10.99934110471000004, -5.081022574063999819, 8.239050178861999640 ) ) ;
#53551=DIRECTION ( 'NONE',  ( -1.000000000000000000, 0.000000000000000000, 0.000000000000000000 ) ) ;
#53557=CARTESIAN_POINT ( 'NONE',  ( 10.69829435321000055, -2.534030585780999711, -6.667788699001999220 ) ) ;
#53558=PLANE ( 'NONE',  #12050 ) ;
#53559=CARTESIAN_POINT ( 'NONE',  ( 9.520528907821001141, -2.899999999999999911, 6.152188490330000370 ) ) ;
#53568=VERTEX_POINT ( 'NONE', #59811 ) ;
#53572=EDGE_CURVE ( 'NONE', #53921, #32830, #34160, .T. ) ;
#53575=CARTESIAN_POINT ( 'NONE',  ( 9.356463691918067482, -5.100000000000000533, 6.665341197419115460 ) ) ;
#53601=CARTESIAN_POINT ( 'NONE',  ( 10.60198654464000079, -2.164987663130000239, -7.764523632348000248 ) ) ;
#53602=ORIENTED_EDGE ( 'NONE', *, *, #23607, .F. ) ;
#53605=CARTESIAN_POINT ( 'NONE',  ( 10.90000000000000036, -5.100000000000000533, -6.436740704805999691 ) ) ;
#53609=CARTESIAN_POINT ( 'NONE',  ( -15.86200481174999943, -5.599999999999999645, -6.571291218949999902 ) ) ;
#53614=CARTESIAN_POINT ( 'NONE',  ( 8.166819129144998968, -2.890362633264002667, 6.359808956951005676 ) ) ;
#53617=CARTESIAN_POINT ( 'NONE',  ( 10.89874164595999950, -2.834836218627000193, 9.088455567997000273 ) ) ;
#53620=CARTESIAN_POINT ( 'NONE',  ( 9.781666627457001439, -5.464740618746000145, 8.817321229216000589 ) ) ;
#53635=CARTESIAN_POINT ( 'NONE',  ( 9.447682302133550536, -5.285671839984060760, 7.027659275301481046 ) ) ;
#53646=CARTESIAN_POINT ( 'NONE',  ( 9.910640133503999749, -2.107273866476999657, 7.885282692430999774 ) ) ;
#53650=CARTESIAN_POINT ( 'NONE',  ( 8.791230646795000325, -5.095088356574999366, 6.286978111459999852 ) ) ;
#53657=B_SPLINE_CURVE_WITH_KNOTS ( 'NONE', 3,
 ( #50384, #8767, #2483, #7731, #46518, #24845, #50730, #66452, #30109, #9102, #19945, #55632, #51751, #51412, #14016 ),
 .UNSPECIFIED., .F., .F.,
 ( 4, 2, 2, 1, 2, 2, 2, 4 ),
 ( 0.000000000000000000, 0.1250000000000078271, 0.1875000000000136280, 0.2187500000000169031, 0.2343750000000154321, 0.2500000000000139333, 0.5000000000000107692, 1.000000000000000000 ),
 .UNSPECIFIED. ) ;
#53663=CARTESIAN_POINT ( 'NONE',  ( 9.290195424034999760, -2.377814350880000038, 7.540992175424999999 ) ) ;
#53670=VERTEX_POINT ( 'NONE', #39530 ) ;
#53676=DIRECTION ( 'NONE',  ( 0.000000000000000000, -1.000000000000000000, 0.000000000000000000 ) ) ;
#53679=ORIENTED_EDGE ( 'NONE', *, *, #58412, .T. ) ;
#53680=CARTESIAN_POINT ( 'NONE',  ( 9.308000177250203677, -4.364660356823166332, 9.210564710512558761 ) ) ;
#53694=CARTESIAN_POINT ( 'NONE',  ( 10.19256470245000123, -2.560274838243000062, 7.664550593243999899 ) ) ;
#53696=CARTESIAN_POINT ( 'NONE',  ( 7.346668146792000087, -2.374041291348000016, 8.293390875797999939 ) ) ;
#53708=CARTESIAN_POINT ( 'NONE',  ( 8.893206853209999707, -3.977267280662000193, 9.308921106447000327 ) ) ;
#53710=AXIS2_PLACEMENT_3D ( 'NONE', #19667, #30502, #18978 ) ;
#53722=CARTESIAN_POINT ( 'NONE',  ( 11.00000000058999916, -1.300000000000000044, -10.56294468516420082 ) ) ;
#53726=CARTESIAN_POINT ( 'NONE',  ( 8.392827495614858080, -2.685109840479763754, 8.639376818827626536 ) ) ;
#53736=ORIENTED_EDGE ( 'NONE', *, *, #62265, .T. ) ;
#53737=CARTESIAN_POINT ( 'NONE',  ( 10.99458782869000117, -8.059061327796998242, 7.168112971386999988 ) ) ;
#53738=( NAMED_UNIT ( * ) PLANE_ANGLE_UNIT ( ) SI_UNIT ( $, .RADIAN. ) );
#53743=ORIENTED_EDGE ( 'NONE', *, *, #59217, .T. ) ;
#53745=EDGE_CURVE ( 'NONE', #683, #18643, #63356, .T. ) ;
#53746=VERTEX_POINT ( 'NONE', #36691 ) ;
#53749=CARTESIAN_POINT ( 'NONE',  ( 5.500000000000000000, 0.8000000000000000444, 3.149999999999999911 ) ) ;
#53759=ORIENTED_EDGE ( 'NONE', *, *, #29507, .F. ) ;
#53771=VECTOR ( 'NONE', #1744, 1000.000000000000000 ) ;
#53772=ORIENTED_EDGE ( 'NONE', *, *, #44922, .T. ) ;
#53784=EDGE_CURVE ( 'NONE', #55729, #33287, #13368, .T. ) ;
#53795=CARTESIAN_POINT ( 'NONE',  ( 9.766851002543001314, -2.832432432432000269, 6.822293592207000934 ) ) ;
#53801=CARTESIAN_POINT ( 'NONE',  ( 10.73930809942999964, -2.762991917822000154, 6.801028165221000066 ) ) ;
#53802=CARTESIAN_POINT ( 'NONE',  ( 7.871558059623000148, -4.780993534312999671, 6.267212032957000467 ) ) ;
#53806=CARTESIAN_POINT ( 'NONE',  ( 10.24394435321000074, -3.220344030624999743, -6.005416930865999703 ) ) ;
#53807=CARTESIAN_POINT ( 'NONE',  ( 7.892384426797941721, -2.680859579914350199, 8.636688153635477150 ) ) ;
#53822=EDGE_LOOP ( 'NONE', ( #9783, #62184, #17073, #61233 ) ) ;
#53826=CARTESIAN_POINT ( 'NONE',  ( 8.111566940377999302, -3.326257819185999942, 8.794522506294001118 ) ) ;
#53835=CARTESIAN_POINT ( 'NONE',  ( 9.465112865370999273, -2.290047720994000002, 6.601709978349000529 ) ) ;
#53841=VERTEX_POINT ( 'NONE', #19836 ) ;
#53856=CARTESIAN_POINT ( 'NONE',  ( 9.299999999999998934, -4.537600397704999899, 9.154563893594000135 ) ) ;
#53857=CARTESIAN_POINT ( 'NONE',  ( 10.37874387220000116, -4.882732524430000609, 6.350796477317000921 ) ) ;
#53885=CARTESIAN_POINT ( 'NONE',  ( 9.648264191885376206, -4.679965170704055488, -8.679680463610704777 ) ) ;
#53887=CARTESIAN_POINT ( 'NONE',  ( 7.307500000000000107, -0.2999999999999999889, 3.149999999999999911 ) ) ;
#53891=CARTESIAN_POINT ( 'NONE',  ( 10.96333185321000059, -5.283547384770999500, -8.592770849731000027 ) ) ;
#53900=CARTESIAN_POINT ( 'NONE',  ( 11.09999999999999964, -5.299999998610999796, 5.148506132424000015 ) ) ;
#53903=CONICAL_SURFACE ( 'NONE', #63928, 0.8999999993723004632, 0.7853981633972997312 ) ;
#53919=VERTEX_POINT ( 'NONE', #64187 ) ;
#53921=VERTEX_POINT ( 'NONE', #27490 ) ;
#53927=CARTESIAN_POINT ( 'NONE',  ( 9.681180837610000367, -2.612237299844000216, 7.804680206899999639 ) ) ;
#53938=CARTESIAN_POINT ( 'NONE',  ( 9.961463664312999455, -2.787129471086000176, -8.677705025472000955 ) ) ;
#53943=CARTESIAN_POINT ( 'NONE',  ( 8.611367277397988573, -2.905107992438832110, 6.370216274085540142 ) ) ;
#53944=LINE ( 'NONE', #42773, #5375 ) ;
#53945=AXIS2_PLACEMENT_3D ( 'NONE', #41456, #10322, #19440 ) ;
#53953=CARTESIAN_POINT ( 'NONE',  ( 9.305875415870998424, -4.945293979885000191, 9.077881967919999795 ) ) ;
#53958=CARTESIAN_POINT ( 'NONE',  ( 10.34020413671000149, -4.202027362542999356, 9.459588031742001135 ) ) ;
#53959=CARTESIAN_POINT ( 'NONE',  ( 9.905947954862410754, -2.481286724714716563, 8.418981899270745473 ) ) ;
#53970=CARTESIAN_POINT ( 'NONE',  ( 9.424850088744616272, -5.349972419855331118, 7.500009359253513530 ) ) ;
#53986=CARTESIAN_POINT ( 'NONE',  ( 10.96876739532000045, -2.333349849211999949, 6.524062020538999640 ) ) ;
#53992=ORIENTED_EDGE ( 'NONE', *, *, #52334, .T. ) ;
#53998=CARTESIAN_POINT ( 'NONE',  ( 9.972852379787999766, -5.044471434015000533, 6.258101649750000384 ) ) ;
#54003=CARTESIAN_POINT ( 'NONE',  ( 10.42511694037999881, -3.371058793856000158, -6.294333763729999198 ) ) ;
#54004=ORIENTED_EDGE ( 'NONE', *, *, #33105, .F. ) ;
#54020=CARTESIAN_POINT ( 'NONE',  ( 10.27814441345999974, -5.521593622715999850, 8.751220666652999469 ) ) ;
#54022=AXIS2_PLACEMENT_3D ( 'NONE', #18617, #24547, #28772 ) ;
#54023=CARTESIAN_POINT ( 'NONE',  ( 7.717918984469999799, -2.852331559125000027, 6.784354950350999225 ) ) ;
#54027=VECTOR ( 'NONE', #47375, 1000.000000000000114 ) ;
#54031=CARTESIAN_POINT ( 'NONE',  ( 7.282480646792000023, -3.448181789123000218, 9.222458996124998976 ) ) ;
#54036=DIRECTION ( 'NONE',  ( 1.000000000000000000, 0.000000000000000000, 0.000000000000000000 ) ) ;
#54046=CARTESIAN_POINT ( 'NONE',  ( 9.047980646795000581, -2.806079842068999852, 8.615883328687999665 ) ) ;
#54048=B_SPLINE_CURVE_WITH_KNOTS ( 'NONE', 3,
 ( #3513, #24851, #40927, #62249 ),
 .UNSPECIFIED., .F., .F.,
 ( 4, 4 ),
 ( 0.000000000000000000, 1.000000000000000000 ),
 .UNSPECIFIED. ) ;
#54058=CARTESIAN_POINT ( 'NONE',  ( 7.000000000000000000, 0.5292307692307999245, 2.083846153846000249 ) ) ;
#54060=CARTESIAN_POINT ( 'NONE',  ( 7.183954769576917698, -2.819171138525097930, 8.180672465553621819 ) ) ;
#54065=CARTESIAN_POINT ( 'NONE',  ( 8.374455264001134935, -2.988149489109947599, 8.916437303143837312 ) ) ;
#54077=CARTESIAN_POINT ( 'NONE',  ( 10.39973737267491138, -5.293988795193000030, -8.716508489687221584 ) ) ;
#54111=DIRECTION ( 'NONE',  ( -0.7071067811865474617, -0.7071067811865474617, -1.029446549002069181E-08 ) ) ;
#54115=CARTESIAN_POINT ( 'NONE',  ( 10.08079553768663672, -5.100000000000000533, -6.662590550639031939 ) ) ;
#54133=ORIENTED_EDGE ( 'NONE', *, *, #62642, .F. ) ;
#54139=ORIENTED_EDGE ( 'NONE', *, *, #16779, .F. ) ;
#54143=CARTESIAN_POINT ( 'NONE',  ( 11.29621718459000057, -3.561654022787999807, 6.266039799355000106 ) ) ;
#54149=CARTESIAN_POINT ( 'NONE',  ( 11.12964314679000033, -3.869080819553999628, -9.017146989745999264 ) ) ;
#54150=CARTESIAN_POINT ( 'NONE',  ( 7.896885084209208649, -2.621122013384412419, 8.559930520408130405 ) ) ;
#54151=CARTESIAN_POINT ( 'NONE',  ( 10.40226385995999969, -2.765692573780999641, 9.035345396600000356 ) ) ;
#54166=CARTESIAN_POINT ( 'NONE',  ( 7.598066940377999678, -3.554853390786000045, 8.889491623367000273 ) ) ;
#54172=EDGE_CURVE ( 'NONE', #51180, #17467, #60028, .T. ) ;
#54176=CARTESIAN_POINT ( 'NONE',  ( 10.80169466977000070, -3.998196228428999355, 9.431543037543999475 ) ) ;
#54180=DIRECTION ( 'NONE',  ( 1.000000000000000000, 0.000000000000000000, 0.000000000000000000 ) ) ;
#54183=EDGE_LOOP ( 'NONE', ( #505, #65580, #50313, #30079 ) ) ;
#54204=CARTESIAN_POINT ( 'NONE',  ( 11.00000000058999916, -1.300000000000000044, -9.662944685757000940 ) ) ;
#54220=FACE_OUTER_BOUND ( 'NONE', #52509, .T. ) ;
#54229=CARTESIAN_POINT ( 'NONE',  ( 10.62947109217999930, -5.100000000000000533, 6.152188490330000370 ) ) ;
#54230=DIRECTION ( 'NONE',  ( 1.000000000000000000, 0.000000000000000000, 0.000000000000000000 ) ) ;
#54235=CARTESIAN_POINT ( 'NONE',  ( 10.54684435321000002, -3.691674321452999674, -9.157280075569998345 ) ) ;
#54237=DIRECTION ( 'NONE',  ( 1.000000000000000000, 0.000000000000000000, 0.000000000000000000 ) ) ;
#54257=CARTESIAN_POINT ( 'NONE',  ( 9.753033816428001046, -4.922930220739999641, -8.639537379291999386 ) ) ;
#54269=CARTESIAN_POINT ( 'NONE',  ( 10.63214998050358773, -2.955201170656483800, 5.051157783803637891 ) ) ;
#54272=CARTESIAN_POINT ( 'NONE',  ( 9.532671748231999587, -4.663050389319001177, 8.669823109968998409 ) ) ;
#54282=CARTESIAN_POINT ( 'NONE',  ( 10.24845588172999911, -4.234132110154000372, -5.660862927546999934 ) ) ;
#54287=CARTESIAN_POINT ( 'NONE',  ( 8.767879976495999372, -3.394455611366999914, -6.293427637271999942 ) ) ;
#54290=EDGE_CURVE ( 'NONE', #42842, #27465, #65836, .T. ) ;
#54296=CARTESIAN_POINT ( 'NONE',  ( 7.925467018026002286, -3.503349646405999884, 6.315515750141001305 ) ) ;
#54297=ORIENTED_EDGE ( 'NONE', *, *, #24051, .T. ) ;
#54301=CARTESIAN_POINT ( 'NONE',  ( 7.925467018026002286, -3.503349646405999884, 6.315515750141001305 ) ) ;
#54304=CARTESIAN_POINT ( 'NONE',  ( 9.075489683949001574, -4.020837068201999820, 8.948702918089999514 ) ) ;
#54316=CARTESIAN_POINT ( 'NONE',  ( 9.933148997456999751, -5.167567567567999731, 6.822293592207000934 ) ) ;
#54331=ORIENTED_EDGE ( 'NONE', *, *, #23517, .T. ) ;
#54336=DIRECTION ( 'NONE',  ( -1.000000000000000000, 0.000000000000000000, 0.000000000000000000 ) ) ;
#54342=CARTESIAN_POINT ( 'NONE',  ( 10.06844525594999951, -4.148609764890999863, 8.941457795715999524 ) ) ;
#54347=CARTESIAN_POINT ( 'NONE',  ( 10.16007944038000055, -4.812966563646999596, -8.526591612524001107 ) ) ;
#54353=EDGE_CURVE ( 'NONE', #5840, #49573, #15687, .T. ) ;
#54379=EDGE_CURVE ( 'NONE', #11630, #25798, #27245, .T. ) ;
#54380=CARTESIAN_POINT ( 'NONE',  ( 9.091120559621998609, -3.762710033898000184, 8.787827024292999667 ) ) ;
#54389=CARTESIAN_POINT ( 'NONE',  ( 11.10000000000000320, -5.584402864533258182, 7.269764875316957919 ) ) ;
#54392=CARTESIAN_POINT ( 'NONE',  ( 8.545870559624999530, -3.856773448568000084, 5.521258396339000285 ) ) ;
#54397=CARTESIAN_POINT ( 'NONE',  ( 9.447288403127886980, -2.899999999999999911, 6.305985889523069154 ) ) ;
#54414=CARTESIAN_POINT ( 'NONE',  ( 8.513685092916551511, -2.802204424339387767, 6.226699829290962995 ) ) ;
#54420=ORIENTED_EDGE ( 'NONE', *, *, #32993, .T. ) ;
#54425=CARTESIAN_POINT ( 'NONE',  ( 10.43232984631212013, -4.711432589314514807, -9.126745072100195699 ) ) ;
#54433=CARTESIAN_POINT ( 'NONE',  ( 10.98768503802999952, -8.067884818888000353, -6.818830313157000056 ) ) ;
#54455=CARTESIAN_POINT ( 'NONE',  ( 10.62924380535000068, -3.609488729914999805, -5.855142811286000004 ) ) ;
#54467=VECTOR ( 'NONE', #57940, 1000.000000000000114 ) ;
#54481=ORIENTED_EDGE ( 'NONE', *, *, #15162, .T. ) ;
#54487=CARTESIAN_POINT ( 'NONE',  ( 10.81499708368651369, -2.650004840405617124, -7.499999822193714749 ) ) ;
#54492=CARTESIAN_POINT ( 'NONE',  ( 10.09181272066999924, -2.440908155048000516, 7.817368209339999652 ) ) ;
#54498=CARTESIAN_POINT ( 'NONE',  ( 10.66043185321000131, -2.315667072036000196, -7.431702410656999547 ) ) ;
#54499=CARTESIAN_POINT ( 'NONE',  ( 7.749273516063919232, -5.411483081375795479, 8.518382685781334729 ) ) ;
#54500=CARTESIAN_POINT ( 'NONE',  ( 11.14698053895999941, -5.129799765052999838, 5.886044098803999702 ) ) ;
#54501=CARTESIAN_POINT ( 'NONE',  ( 10.14577693501968803, -2.689538146648244421, 7.995535515817278949 ) ) ;
#54504=B_SPLINE_CURVE_WITH_KNOTS ( 'NONE', 3,
 ( #18709, #18026, #13128, #60320, #7516, #23598, #44941, #49478, #55770, #7872, #40040, #61353, #29208, #8213 ),
 .UNSPECIFIED., .F., .F.,
 ( 4, 2, 2, 2, 2, 2, 4 ),
 ( 0.000000000000000000, 0.1249999999999997224, 0.2499999999999994449, 0.4999999999999991118, 0.7499999999999987788, 0.8749999999999993339, 1.000000000000000000 ),
 .UNSPECIFIED. ) ;
#54517=AXIS2_PLACEMENT_3D ( 'NONE', #47815, #24850, #10390 ) ;
#54525=CARTESIAN_POINT ( 'NONE',  ( 10.00190805961999807, -2.729654112791000120, -8.843024969850999284 ) ) ;
#54528=EDGE_CURVE ( 'NONE', #8090, #31317, #34893, .T. ) ;
#54538=ORIENTED_EDGE ( 'NONE', *, *, #43349, .T. ) ;
#54551=FACE_OUTER_BOUND ( 'NONE', #27570, .T. ) ;
#54553=CARTESIAN_POINT ( 'NONE',  ( 10.44080359545000114, -5.435731278187999393, 7.303630150377999009 ) ) ;
#54558=DIRECTION ( 'NONE',  ( -0.7071067811865474617, -0.7071067811865474617, -7.650295924916503855E-09 ) ) ;
#54584=DIRECTION ( 'NONE',  ( 0.000000000000000000, 1.000000000000000000, 0.000000000000000000 ) ) ;
#54587=CARTESIAN_POINT ( 'NONE',  ( 9.972537864286000087, -2.899999999999999911, -6.571291218949999902 ) ) ;
#54593=CARTESIAN_POINT ( 'NONE',  ( 11.03905685320999908, -3.855072944465999907, -9.179476187420998912 ) ) ;
#54594=FACE_OUTER_BOUND ( 'NONE', #45527, .T. ) ;
#54596=DIRECTION ( 'NONE',  ( 1.000000000000000000, 0.000000000000000000, 0.000000000000000000 ) ) ;
#54607=CARTESIAN_POINT ( 'NONE',  ( 10.90000000000000036, -1.433333333332999837, 10.65401593558000037 ) ) ;
#54611=CARTESIAN_POINT ( 'NONE',  ( 11.19120431613999855, -3.005395205805000192, -6.023553580263000029 ) ) ;
#54612=CARTESIAN_POINT ( 'NONE',  ( 10.08492069073747466, -4.544768192061120260, -8.875938726815583379 ) ) ;
#54616=CARTESIAN_POINT ( 'NONE',  ( 10.71937333909091450, -2.934588105059417362, -5.069903530434454630 ) ) ;
#54623=CYLINDRICAL_SURFACE ( 'NONE', #60874, 1.350000000000000089 ) ;
#54631=CARTESIAN_POINT ( 'NONE',  ( 10.67008478491585066, -2.650321919618085609, 7.583525828155321058 ) ) ;
#54639=CARTESIAN_POINT ( 'NONE',  ( 10.35427551197999918, -4.879111827962000270, -8.944027914303999793 ) ) ;
#54641=CARTESIAN_POINT ( 'NONE',  ( 10.17500046684972936, -2.650307855384914202, 7.500001770945068813 ) ) ;
#54654=CARTESIAN_POINT ( 'NONE',  ( 9.566960887370999700, -5.215923019114000247, 6.177729435798999802 ) ) ;
#54657=CARTESIAN_POINT ( 'NONE',  ( 11.05639424537999993, -5.030223832177999732, 6.028291574375000295 ) ) ;
#54669=CARTESIAN_POINT ( 'NONE',  ( 7.770167153117901293, -2.851532783649957548, 6.786996034065015948 ) ) ;
#54672=ORIENTED_EDGE ( 'NONE', *, *, #55712, .T. ) ;
#54676=CARTESIAN_POINT ( 'NONE',  ( 9.928197172112565028, -5.125396288433639036, 6.749639981095324259 ) ) ;
#54686=CARTESIAN_POINT ( 'NONE',  ( 9.294724726289000927, -4.148132978932999926, 9.337467253566000380 ) ) ;
#54694=CARTESIAN_POINT ( 'NONE',  ( 10.97865453029000093, -5.273142482194999481, 7.958032781726000593 ) ) ;
#54695=EDGE_CURVE ( 'NONE', #51171, #3171, #65713, .T. ) ;
#54701=CARTESIAN_POINT ( 'NONE',  ( 10.76587944038000089, -3.166536971515000243, -8.574494061818999313 ) ) ;
#54708=B_SPLINE_CURVE_WITH_KNOTS ( 'NONE', 3,
 ( #47216, #26235, #58727, #5580, #15741, #52102, #14712, #67837 ),
 .UNSPECIFIED., .F., .F.,
 ( 4, 1, 1, 1, 1, 4 ),
 ( 0.000000000000000000, 0.2000000000000000111, 0.4000000000000000222, 0.5999999999999999778, 0.8000000000000000444, 1.000000000000000000 ),
 .UNSPECIFIED. ) ;
#54712=CARTESIAN_POINT ( 'NONE',  ( 8.229423500915721945, -4.864029983609895247, 6.209053182952776417 ) ) ;
#54719=CARTESIAN_POINT ( 'NONE',  ( 9.905786073958001481, -2.698967003257000119, 8.979227319929000473 ) ) ;
#54723=ORIENTED_EDGE ( 'NONE', *, *, #56776, .T. ) ;
#54728=CARTESIAN_POINT ( 'NONE',  ( 9.648858509738902356, -2.900412407185302577, -6.176298919794867004 ) ) ;
#54730=CARTESIAN_POINT ( 'NONE',  ( 8.834370559623998531, -4.141908960411000429, 6.047561724438000219 ) ) ;
#54734=CARTESIAN_POINT ( 'NONE',  ( 11.12483846379999974, -5.434435013714999485, 5.164704272902999271 ) ) ;
#54742=ORIENTED_EDGE ( 'NONE', *, *, #11258, .F. ) ;
#54747=CARTESIAN_POINT ( 'NONE',  ( 10.16000000000000014, -4.496968146123999865, -8.755198255949000696 ) ) ;
#54753=DIRECTION ( 'NONE',  ( 0.000000000000000000, -0.1333333333333049098, 0.9910712498212373989 ) ) ;
#54756=ORIENTED_EDGE ( 'NONE', *, *, #49962, .T. ) ;
#54772=DIRECTION ( 'NONE',  ( 0.000000000000000000, 0.000000000000000000, -1.000000000000000000 ) ) ;
#54774=CARTESIAN_POINT ( 'NONE',  ( 9.470944094206000585, -5.100000000000000533, 6.571291218949999902 ) ) ;
#54776=ORIENTED_EDGE ( 'NONE', *, *, #23404, .T. ) ;
#54801=CARTESIAN_POINT ( 'NONE',  ( 10.14584566409999944, -5.370505908760000224, -6.826219946961000318 ) ) ;
#54811=CARTESIAN_POINT ( 'NONE',  ( 8.896432056425105372, -5.285622111567716885, 7.027794277398525580 ) ) ;
#54816=CARTESIAN_POINT ( 'NONE',  ( 8.616332382228000242, -2.832433105983000132, -6.822293595522999965 ) ) ;
#54823=CARTESIAN_POINT ( 'NONE',  ( 8.502043146794999728, -3.869396851328000153, 5.695656592546999519 ) ) ;
#54824=CARTESIAN_POINT ( 'NONE',  ( 10.01574583856000089, -4.333399685216000385, -9.088699530815999239 ) ) ;
#54841=CARTESIAN_POINT ( 'NONE',  ( 9.632185590920999019, -5.638162562978999759, 6.476633609657000079 ) ) ;
#54846=CARTESIAN_POINT ( 'NONE',  ( 10.56170564679000101, -5.057490041178001050, -8.595713413570999606 ) ) ;
#54847=CARTESIAN_POINT ( 'NONE',  ( 7.745598420978331511, -5.458216742540686894, 8.448484368435345004 ) ) ;
#54848=CARTESIAN_POINT ( 'NONE',  ( 9.753140057121997941, -4.104977100659999323, 9.293279163877999238 ) ) ;
#54863=CARTESIAN_POINT ( 'NONE',  ( 8.869959105252339882, -2.899999999999999911, 6.481052078534832006 ) ) ;
#54866=VERTEX_POINT ( 'NONE', #11140 ) ;
#54867=CARTESIAN_POINT ( 'NONE',  ( 7.533879440377999614, -4.623636604834999275, 8.651469651195000665 ) ) ;
#54872=CARTESIAN_POINT ( 'NONE',  ( 10.68343305961999867, -3.810133104029999718, -5.661126601970999594 ) ) ;
#54875=CARTESIAN_POINT ( 'NONE',  ( 8.017297003156455659, -5.179978819780794552, 8.180934229233972843 ) ) ;
#54885=DIRECTION ( 'NONE',  ( -1.264998825433999916E-10, -1.265000103913999927E-10, 1.000000000000000000 ) ) ;
#54931=FACE_OUTER_BOUND ( 'NONE', #49092, .T. ) ;
#54941=CARTESIAN_POINT ( 'NONE',  ( 10.37239314679000124, -3.992345679293999972, -5.977234595428000397 ) ) ;
#54945=EDGE_LOOP ( 'NONE', ( #17287, #6465, #66084, #3299 ) ) ;
#54946=CARTESIAN_POINT ( 'NONE',  ( 11.09999999999999964, -5.299771130038000599, 5.136740763824000133 ) ) ;
#54959=CARTESIAN_POINT ( 'NONE',  ( 9.949439740260999088, -2.508493821066999807, -7.171861383782999866 ) ) ;
#54965=VERTEX_POINT ( 'NONE', #17421 ) ;
#54972=CARTESIAN_POINT ( 'NONE',  ( 9.555699158955999195, -2.440755924888999839, 6.680881588809999272 ) ) ;
#54974=EDGE_CURVE ( 'NONE', #15766, #54866, #18177, .T. ) ;
#54977=B_SPLINE_CURVE_WITH_KNOTS ( 'NONE', 3,
 ( #59879, #22819, #11985, #30829 ),
 .UNSPECIFIED., .F., .F.,
 ( 4, 4 ),
 ( 0.000000000000000000, 0.1254144463278223376 ),
 .UNSPECIFIED. ) ;
#54987=CARTESIAN_POINT ( 'NONE',  ( 10.95551720753999980, -4.744041807741999683, -9.198129812222999746 ) ) ;
#54989=CYLINDRICAL_SURFACE ( 'NONE', #20340, 1.350000000000000089 ) ;
#55001=CARTESIAN_POINT ( 'NONE',  ( 10.96080136920999948, -2.054580854576999904, 7.810082699133999995 ) ) ;
#55005=CARTESIAN_POINT ( 'NONE',  ( 9.104016254283999743, -5.045864843302999780, 8.527867871227000407 ) ) ;
#55014=CARTESIAN_POINT ( 'NONE',  ( 9.933148997456999751, -5.167567567567999731, 6.822293592207000934 ) ) ;
#55032=CARTESIAN_POINT ( 'NONE',  ( 5.600000000706000236, 0.8000000000000000444, -3.149999999999999911 ) ) ;
#55036=CARTESIAN_POINT ( 'NONE',  ( 8.224933059623998233, -5.629389383493999865, 8.631822608164000599 ) ) ;
#55038=CARTESIAN_POINT ( 'NONE',  ( 11.09999999999999964, -2.289217163982593561, -7.673604523768878138 ) ) ;
#55041=CARTESIAN_POINT ( 'NONE',  ( 11.08333333333538562, -2.470076941867837217, 7.228155005602529215 ) ) ;
#55046=ORIENTED_EDGE ( 'NONE', *, *, #55168, .F. ) ;
#55058=CARTESIAN_POINT ( 'NONE',  ( 9.351200703499365829, -3.426673320826296276, 9.142253940106426668 ) ) ;
#55066=CARTESIAN_POINT ( 'NONE',  ( 9.442841440870999747, -2.691258483914000355, 6.269525829285999663 ) ) ;
#55069=ORIENTED_EDGE ( 'NONE', *, *, #44390, .T. ) ;
#55074=CARTESIAN_POINT ( 'NONE',  ( 9.261668853699999815, -2.944250413017999612, 6.507387951280999339 ) ) ;
#55075=LINE ( 'NONE', #19041, #68512 ) ;
#55076=CARTESIAN_POINT ( 'NONE',  ( 7.807370559623000084, -3.650411072918999800, 6.083135626079000602 ) ) ;
#55079=CARTESIAN_POINT ( 'NONE',  ( 11.01665855156000084, -6.699723434166000580, 5.516656797456000128 ) ) ;
#55102=CARTESIAN_POINT ( 'NONE',  ( 7.808998088039303731, -3.043595652559401898, 6.499272882928453399 ) ) ;
#55109=CARTESIAN_POINT ( 'NONE',  ( 8.576768274605196751, -4.042014915351536786, 5.760874511329109104 ) ) ;
#55114=CARTESIAN_POINT ( 'NONE',  ( 10.29378083128999855, -3.483628580733000302, 6.176326635498999629 ) ) ;
#55117=CARTESIAN_POINT ( 'NONE',  ( 9.406851002546000373, -2.832432432432000269, -6.822293592207000934 ) ) ;
#55121=CARTESIAN_POINT ( 'NONE',  ( 9.011117069441999305, -8.696115174831000161, 6.406018931393000493 ) ) ;
#55141=ORIENTED_EDGE ( 'NONE', *, *, #55505, .F. ) ;
#55147=CARTESIAN_POINT ( 'NONE',  ( 9.753033816428001046, -4.922930220739999641, -8.639537379291999386 ) ) ;
#55150=LINE ( 'NONE', #59702, #44545 ) ;
#55165=ORIENTED_EDGE ( 'NONE', *, *, #53784, .T. ) ;
#55166=CARTESIAN_POINT ( 'NONE',  ( 8.464254440379999522, -2.029110377978999846, 7.726994002375999315 ) ) ;
#55167=CARTESIAN_POINT ( 'NONE',  ( 9.842321917838999568, -3.423478821957000040, -6.068694811299999436 ) ) ;
#55168=EDGE_CURVE ( 'NONE', #59694, #67173, #50960, .T. ) ;
#55183=CARTESIAN_POINT ( 'NONE',  ( 10.46754921866999943, -2.318350880468999620, 6.549783596838000044 ) ) ;
#55186=ORIENTED_EDGE ( 'NONE', *, *, #39002, .T. ) ;
#55188=B_SPLINE_CURVE_WITH_KNOTS ( 'NONE', 3,
 ( #22180, #43520, #64819, #33027 ),
 .UNSPECIFIED., .F., .F.,
 ( 4, 4 ),
 ( 0.000000000000000000, 1.000000000000000000 ),
 .UNSPECIFIED. ) ;
#55189=CARTESIAN_POINT ( 'NONE',  ( 10.76587944038000089, -3.166536971515000243, -8.574494061818999313 ) ) ;
#55192=CARTESIAN_POINT ( 'NONE',  ( 7.966778298513556678, -2.303323755512395543, 7.117734776878376302 ) ) ;
#55193=CARTESIAN_POINT ( 'NONE',  ( 9.786673210037999837, -2.381198102024000285, 7.612749732462000374 ) ) ;
#55212=DIRECTION ( 'NONE',  ( 0.000000000000000000, -0.8648648648648717963, -0.5020047465136829867 ) ) ;
#55218=DIRECTION ( 'NONE',  ( -1.000000000000000000, 0.000000000000000000, 0.000000000000000000 ) ) ;
#55260=CARTESIAN_POINT ( 'NONE',  ( 8.111566940377999302, -3.326257819185999942, 8.794522506294001118 ) ) ;
#55265=EDGE_CURVE ( 'NONE', #69025, #60711, #12217, .T. ) ;
#55270=B_SPLINE_CURVE_WITH_KNOTS ( 'NONE', 3,
 ( #35003, #2823, #3845, #45488, #40240, #14362, #29421, #66803, #35345, #67136, #67821, #60872, #51071, #29074, #46172, #61558, #23809, #19247 ),
 .UNSPECIFIED., .F., .F.,
 ( 4, 2, 2, 2, 2, 2, 2, 2, 4 ),
 ( 0.000000000000000000, 0.1250000000000000000, 0.2500000000000000000, 0.3750000000000000000, 0.5000000000000000000, 0.6250000000000000000, 0.7500000000000000000, 0.8750000000000000000, 1.000000000000000000 ),
 .UNSPECIFIED. ) ;
#55290=CARTESIAN_POINT ( 'NONE',  ( 5.500000000595999694, -0.4999999994045000173, 3.150000007847999939 ) ) ;
#55294=EDGE_LOOP ( 'NONE', ( #23043, #16397, #64697, #52356, #7522, #40964 ) ) ;
#55295=CARTESIAN_POINT ( 'NONE',  ( 10.98768503802999952, -8.067884818888000353, -6.818830313157000056 ) ) ;
#55303=FACE_OUTER_BOUND ( 'NONE', #33230, .T. ) ;
#55307=CARTESIAN_POINT ( 'NONE',  ( 10.94349328348999961, -3.081618981425999770, -8.919377696680001577 ) ) ;
#55310=ORIENTED_EDGE ( 'NONE', *, *, #27056, .F. ) ;
#55313=CARTESIAN_POINT ( 'NONE',  ( 10.25832651750999958, -4.639457704266000349, 4.530776779397999832 ) ) ;
#55319=CARTESIAN_POINT ( 'NONE',  ( 10.72520823780999955, -5.521647200017000934, 6.612992938078999572 ) ) ;
#55324=ORIENTED_EDGE ( 'NONE', *, *, #59174, .F. ) ;
#55333=CARTESIAN_POINT ( 'NONE',  ( 6.992190918810999634, -9.194554705909000702, -5.189167530940999917 ) ) ;
#55336=CARTESIAN_POINT ( 'NONE',  ( 9.749327024990000368, -5.634417356902000407, -7.003562403358999156 ) ) ;
#55342=CARTESIAN_POINT ( 'NONE',  ( 11.00478015909000007, -2.938058373007000235, 5.194088448331000585 ) ) ;
#55347=CARTESIAN_POINT ( 'NONE',  ( 11.02786767503999954, -5.596230239120999705, 7.209501483790000442 ) ) ;
#55350=CARTESIAN_POINT ( 'NONE',  ( 9.600494040286998043, -5.206548117663999165, 8.585114612872999373 ) ) ;
#55354=ORIENTED_EDGE ( 'NONE', *, *, #63982, .F. ) ;
#55365=CARTESIAN_POINT ( 'NONE',  ( 9.392147628284998717, -2.890602650755999647, -6.682694598879999504 ) ) ;
#55368=DIRECTION ( 'NONE',  ( -0.8660254037844974384, 0.000000000000000000, 0.4999999999998981925 ) ) ;
#55380=CARTESIAN_POINT ( 'NONE',  ( 8.674245559624999657, -5.983034890242000081, 7.440798487724999966 ) ) ;
#55386=CARTESIAN_POINT ( 'NONE',  ( 9.327567085901730337, -5.070068301512486997, -6.253587086782717464 ) ) ;
#55389=DIRECTION ( 'NONE',  ( 1.000000000000000000, 0.000000000000000000, 0.000000000000000000 ) ) ;
#55394=CARTESIAN_POINT ( 'NONE',  ( 11.03775575519999919, -8.050335494570999728, 6.914609630061999468 ) ) ;
#55406=EDGE_CURVE ( 'NONE', #21093, #21223, #13098, .T. ) ;
#55407=CARTESIAN_POINT ( 'NONE',  ( 9.409668643352913975, -2.474094513855759736, 8.334984523595771577 ) ) ;
#55409=CARTESIAN_POINT ( 'NONE',  ( 8.228673373757093401, -4.831901240730346103, 6.190044060663523418 ) ) ;
#55421=CARTESIAN_POINT ( 'NONE',  ( 10.72510394928771227, -2.650147065043205519, 7.500007457243348163 ) ) ;
#55426=CARTESIAN_POINT ( 'NONE',  ( 8.732394353210001015, -2.806079842068999852, 8.615883328687999665 ) ) ;
#55429=CARTESIAN_POINT ( 'NONE',  ( 11.12483852207999924, -6.576352438315999471, 5.637707935939000770 ) ) ;
#55438=CARTESIAN_POINT ( 'NONE',  ( 8.738433059624998833, -5.414909314743000301, 8.890670256079998168 ) ) ;
#55442=CARTESIAN_POINT ( 'NONE',  ( 8.354417780085995560, -5.125509315120996057, 6.367236178909004174 ) ) ;
#55444=EDGE_CURVE ( 'NONE', #43366, #50721, #15620, .T. ) ;
#55449=CARTESIAN_POINT ( 'NONE',  ( 7.805362843630345715, -2.998771363040654947, 6.543984068746279803 ) ) ;
#55456=DIRECTION ( 'NONE',  ( 1.000000000000000000, 0.000000000000000000, 0.000000000000000000 ) ) ;
#55459=EDGE_LOOP ( 'NONE', ( #20757, #55186, #20167, #54139 ) ) ;
#55481=CARTESIAN_POINT ( 'NONE',  ( 10.56577346846700038, -5.100000000000000533, 6.304440313576233024 ) ) ;
#55485=DIRECTION ( 'NONE',  ( -1.000000000000000000, 0.000000000000000000, 0.000000000000000000 ) ) ;
#55492=ORIENTED_EDGE ( 'NONE', *, *, #67383, .T. ) ;
#55496=CARTESIAN_POINT ( 'NONE',  ( 9.949439740260999088, -2.508493821066999807, -7.171861383782999866 ) ) ;
#55498=CARTESIAN_POINT ( 'NONE',  ( 11.10000000009000054, -2.699999999911000259, 6.571291220400000022 ) ) ;
#55499=DIRECTION ( 'NONE',  ( 1.000000000000000000, 0.000000000000000000, 0.000000000000000000 ) ) ;
#55500=ORIENTED_EDGE ( 'NONE', *, *, #65918, .F. ) ;
#55504=CARTESIAN_POINT ( 'NONE',  ( 10.78170625604285782, -3.320082702567464850, -8.679590637733081593 ) ) ;
#55505=EDGE_CURVE ( 'NONE', #67663, #683, #17295, .T. ) ;
#55515=AXIS2_PLACEMENT_3D ( 'NONE', #49564, #7954, #29292 ) ;
#55523=VECTOR ( 'NONE', #38932, 1000.000000000000000 ) ;
#55536=CARTESIAN_POINT ( 'NONE',  ( 10.16829915263999951, -4.567213659083999566, 5.832528837986999726 ) ) ;
#55541=CARTESIAN_POINT ( 'NONE',  ( 8.092827459944675894, -4.405392649884461775, 5.808720040846370836 ) ) ;
#55542=CARTESIAN_POINT ( 'NONE',  ( 11.15982711745999900, -5.578228817597000955, 8.067792329320999656 ) ) ;
#55551=CARTESIAN_POINT ( 'NONE',  ( 9.573145925901000552, -2.133039813254999917, -7.346564890486999566 ) ) ;
#55562=CARTESIAN_POINT ( 'NONE',  ( 9.047980646795000581, -2.806079842068999852, 8.615883328687999665 ) ) ;
#55571=CARTESIAN_POINT ( 'NONE',  ( 8.090129597172618148, -4.176673380088065990, 8.851094058678157239 ) ) ;
#55603=ORIENTED_EDGE ( 'NONE', *, *, #62120, .F. ) ;
#55608=CARTESIAN_POINT ( 'NONE',  ( 8.432504440379000599, -5.430412429559000387, 7.210798766422999329 ) ) ;
#55619=VECTOR ( 'NONE', #996, 1000.000000000000114 ) ;
#55627=CARTESIAN_POINT ( 'NONE',  ( 7.451720376979478644, -2.261709126496390443, 7.443204203363470661 ) ) ;
#55632=CARTESIAN_POINT ( 'NONE',  ( 10.48389394032039235, -4.970831725323499484, 5.006796266880559010 ) ) ;
#55635=EDGE_CURVE ( 'NONE', #14642, #44229, #68918, .T. ) ;
#55638=CARTESIAN_POINT ( 'NONE',  ( 11.25809194037999994, -3.275508415657999883, -8.650784343212000849 ) ) ;
#55648=CARTESIAN_POINT ( 'NONE',  ( 8.973567461188688199, -5.349887746458779070, 7.470579050607700111 ) ) ;
#55659=CARTESIAN_POINT ( 'NONE',  ( 10.81379776946905125, -2.908665697285443219, -5.100634573475641531 ) ) ;
#55665=CARTESIAN_POINT ( 'NONE',  ( 10.75580099727000061, -5.294318740464999173, 4.786926179488999900 ) ) ;
#55670=CARTESIAN_POINT ( 'NONE',  ( 9.701976361057999654, -3.399137684422000039, 6.026753338319999820 ) ) ;
#55677=CARTESIAN_POINT ( 'NONE',  ( 10.64659662355864711, -2.685854016001090638, 7.981709294338716454 ) ) ;
#55682=CARTESIAN_POINT ( 'NONE',  ( 8.361784236169967244, -5.107027742527944447, 6.686924772338650236 ) ) ;
#55688=CARTESIAN_POINT ( 'NONE',  ( 9.700159544970999193, -4.268950419651999617, -8.781589108989999559 ) ) ;
#55694=CARTESIAN_POINT ( 'NONE',  ( 10.70985928442000024, -2.874451299444999552, 5.003015709877000283 ) ) ;
#55697=ORIENTED_EDGE ( 'NONE', *, *, #45011, .T. ) ;
#55699=CARTESIAN_POINT ( 'NONE',  ( 10.65550933554000146, -4.237674644795000667, 9.105223721671999115 ) ) ;
#55702=CARTESIAN_POINT ( 'NONE',  ( 10.34521071928999980, -2.724119865955000108, 6.497322598008000050 ) ) ;
#55712=EDGE_CURVE ( 'NONE', #67791, #53475, #20639, .T. ) ;
#55716=CARTESIAN_POINT ( 'NONE',  ( 9.441315108303999892, -3.111669560323000017, -8.958991988670002016 ) ) ;
#55718=VERTEX_POINT ( 'NONE', #21043 ) ;
#55719=CARTESIAN_POINT ( 'NONE',  ( 9.911033975247157457, -5.348894881546552682, 7.263563640299063096 ) ) ;
#55729=VERTEX_POINT ( 'NONE', #14431 ) ;
#55742=ORIENTED_EDGE ( 'NONE', *, *, #58396, .T. ) ;
#55754=CARTESIAN_POINT ( 'NONE',  ( 9.428389268916888000, -2.310473079787241257, 7.963614157108587222 ) ) ;
#55761=CARTESIAN_POINT ( 'NONE',  ( 11.06924082387999952, -5.425685649895999774, 8.012912555523998392 ) ) ;
#55766=EDGE_LOOP ( 'NONE', ( #1794, #22169, #62336, #46857 ) ) ;
#55770=CARTESIAN_POINT ( 'NONE',  ( 9.242435128169496750, -5.510362259932574780, 8.414241021983331237 ) ) ;
#55771=CARTESIAN_POINT ( 'NONE',  ( 8.128308059623998716, -3.117370956513999758, 8.662188901935000018 ) ) ;
#55779=CARTESIAN_POINT ( 'NONE',  ( 10.90000000296000060, -5.100000000009000445, 5.160242730682999657 ) ) ;
#55783=CARTESIAN_POINT ( 'NONE',  ( 11.09999999999999964, -3.512324525112999751, -8.971282648301999174 ) ) ;
#55789=B_SPLINE_SURFACE_WITH_KNOTS ( 'NONE', 3, 3, ( 
 ( #45288, #61357, #60325, #59975 ),
 ( #55429, #7520, #55079, #2623 ),
 ( #12781, #17326, #12085, #39345 ),
 ( #44946, #13478, #34797, #23604 ),
 ( #56108, #33416, #6834, #66594 ),
 ( #7185, #12433, #18713, #38652 ),
 ( #66250, #28522, #40046, #8219 ),
 ( #54734, #2966, #29567, #49833 ),
 ( #34461, #50869, #45632, #28875 ) ),
 .UNSPECIFIED., .F., .F., .F.,
 ( 4, 1, 1, 1, 1, 1, 4 ),
 ( 4, 4 ),
 ( -0.01830387170767999727, 0.000000000000000000, 0.2500000000000000000, 0.5000000000000000000, 0.7500000000000000000, 1.000000000000000000, 1.018541916426999983 ),
 ( -0.2206046696922999983, 1.220604669692000099 ),
 .UNSPECIFIED. ) ;
#55796=CARTESIAN_POINT ( 'NONE',  ( 7.801415703136094670, -2.973868799469420843, 6.571950203487468833 ) ) ;
#55797=CARTESIAN_POINT ( 'NONE',  ( 11.07484075165016613, -2.725159248349832364, -6.497852970900667380 ) ) ;
#55799=DIRECTION ( 'NONE',  ( 1.000000000000000000, 0.000000000000000000, 0.000000000000000000 ) ) ;
#55802=EDGE_CURVE ( 'NONE', #21511, #18362, #25593, .T. ) ;
#55805=CARTESIAN_POINT ( 'NONE',  ( 8.610875063856999745, -4.757997781751000410, 5.934102420827000124 ) ) ;
#55806=CARTESIAN_POINT ( 'NONE',  ( 9.076707875513999824, -5.109724393580905577, -6.693505495912332570 ) ) ;
#55813=CARTESIAN_POINT ( 'NONE',  ( 8.341918146793998901, -5.601799093797000140, 7.176147756900999930 ) ) ;
#55817=CARTESIAN_POINT ( 'NONE',  ( 8.856463691919834957, -5.100000000000000533, 6.665341197420979746 ) ) ;
#55818=LINE ( 'NONE', #50225, #44895 ) ;
#55824=CYLINDRICAL_SURFACE ( 'NONE', #50617, 0.5000000000000004441 ) ;
#55826=CARTESIAN_POINT ( 'NONE',  ( 9.702711596877973577, -5.100000000000000533, 6.305985889537642386 ) ) ;
#55828=CARTESIAN_POINT ( 'NONE',  ( 10.71685100253999856, -2.832432432432000269, 6.822293592207000934 ) ) ;
#55829=DIRECTION ( 'NONE',  ( 1.000000000000000000, 2.664535258987999937E-14, 3.552713678651000428E-14 ) ) ;
#55832=CARTESIAN_POINT ( 'NONE',  ( 5.500000000000000000, 0.000000000000000000, 0.000000000000000000 ) ) ;
#55835=ORIENTED_EDGE ( 'NONE', *, *, #8362, .F. ) ;
#55841=CARTESIAN_POINT ( 'NONE',  ( 10.32701825126999928, -5.663784181836000187, -6.682035927671000408 ) ) ;
#55850=B_SPLINE_CURVE_WITH_KNOTS ( 'NONE', 3,
 ( #22363, #16764, #60123, #54875, #28662, #65702, #34251, #17825, #55571, #23052, #12574, #12924, #39140, #44402 ),
 .UNSPECIFIED., .F., .F.,
 ( 4, 2, 2, 2, 2, 2, 4 ),
 ( 0.1255288163819863745, 0.2191764973934874350, 0.3128241784049884955, 0.4064718594164895560, 0.5001195404279905610, 0.6874149024509927930, 0.8747102644739948030 ),
 .UNSPECIFIED. ) ;
#55852=LINE ( 'NONE', #6910, #68926 ) ;
#55863=CARTESIAN_POINT ( 'NONE',  ( 8.630418146794999856, -5.808258301303999893, 7.446016267012000256 ) ) ;
#55865=CARTESIAN_POINT ( 'NONE',  ( 11.09999058424243046, -2.671414376110614164, 6.690776694877762942 ) ) ;
#55879=CARTESIAN_POINT ( 'NONE',  ( 11.03855816545999957, -2.974093234901999949, 8.716125417860000724 ) ) ;
#55881=ORIENTED_EDGE ( 'NONE', *, *, #52699, .F. ) ;
#55885=CARTESIAN_POINT ( 'NONE',  ( 10.65229194037999960, -4.944342461481999962, -8.478476072358999360 ) ) ;
#55886=AXIS2_PLACEMENT_3D ( 'NONE', #12973, #50368, #67121 ) ;
#55887=CARTESIAN_POINT ( 'NONE',  ( 7.916668338613877864, -2.408209902419789827, 8.201634448280884726 ) ) ;
#55888=CARTESIAN_POINT ( 'NONE',  ( 9.013429960698999821, -4.933961117404000341, 8.417889755737999025 ) ) ;
#55908=CARTESIAN_POINT ( 'NONE',  ( 9.475897313459000770, -4.122021308488999836, 9.013573548576999883 ) ) ;
#55913=CARTESIAN_POINT ( 'NONE',  ( 11.09992055961999924, -2.373397911211000189, -6.776606350776999577 ) ) ;
#55924=LINE ( 'NONE', #39845, #61512 ) ;
#55928=VECTOR ( 'NONE', #3631, 1000.000000000000000 ) ;
#55932=EDGE_CURVE ( 'NONE', #57184, #61413, #4770, .T. ) ;
#55944=ORIENTED_EDGE ( 'NONE', *, *, #38432, .F. ) ;
#55947=CARTESIAN_POINT ( 'NONE',  ( 10.81600392782857867, -4.193768045697381375, 9.228900182785400474 ) ) ;
#55948=FACE_OUTER_BOUND ( 'NONE', #1788, .T. ) ;
#55949=FACE_OUTER_BOUND ( 'NONE', #3672, .T. ) ;
#55956=CARTESIAN_POINT ( 'NONE',  ( 7.000000000000000000, -6.495643345158865323, 2.999999999999999556 ) ) ;
#55961=CARTESIAN_POINT ( 'NONE',  ( 8.785191940379998954, -5.414909314743000301, 8.890670256079998168 ) ) ;
#55962=ORIENTED_EDGE ( 'NONE', *, *, #50434, .F. ) ;
#55966=ADVANCED_FACE ( 'NONE', ( #50372 ), #56648, .T. ) ;
#55973=DIRECTION ( 'NONE',  ( 0.000000000000000000, 1.000000000000000000, 0.000000000000000000 ) ) ;
#55977=CARTESIAN_POINT ( 'NONE',  ( 8.624774230494178795, -4.944546604704892268, 6.044843339268166638 ) ) ;
#55980=DIRECTION ( 'NONE',  ( -0.6684585169941805738, 0.6684585169941805738, 0.3260773253629903334 ) ) ;
#55997=CARTESIAN_POINT ( 'NONE',  ( 10.64872180584000105, -2.614778238704999591, 6.717279975758000177 ) ) ;
#56002=EDGE_LOOP ( 'NONE', ( #64467, #19036, #37236, #23191, #10659 ) ) ;
#56008=CARTESIAN_POINT ( 'NONE',  ( 10.81579453138999902, -5.374572909254000663, 6.698726302909000729 ) ) ;
#56020=VECTOR ( 'NONE', #21010, 1000.000000000000000 ) ;
#56023=CARTESIAN_POINT ( 'NONE',  ( 9.485316810687001166, -2.477793449086000077, -8.275032865112999403 ) ) ;
#56030=CARTESIAN_POINT ( 'NONE',  ( 10.97534709859367474, -5.193992591243323353, -6.717726803882955622 ) ) ;
#56033=AXIS2_PLACEMENT_3D ( 'NONE', #56435, #8537, #29887 ) ;
#56034=CARTESIAN_POINT ( 'NONE',  ( 10.31167756636999933, -2.874479384703000129, 8.900026329558999194 ) ) ;
#56037=CARTESIAN_POINT ( 'NONE',  ( 10.99934110471000004, -5.081022574063999819, 8.239050178861999640 ) ) ;
#56040=EDGE_CURVE ( 'NONE', #51763, #23757, #36643, .T. ) ;
#56048=CARTESIAN_POINT ( 'NONE',  ( 9.394730517101999467, -2.624921803719999946, -8.200122328058998988 ) ) ;
#56049=CARTESIAN_POINT ( 'NONE',  ( 10.20577346834789267, -5.100000000000000533, -6.304440313861129574 ) ) ;
#56054=CARTESIAN_POINT ( 'NONE',  ( 11.09999999999999964, -2.700688486617000006, 5.124965750789000296 ) ) ;
#56060=CARTESIAN_POINT ( 'NONE',  ( 9.115000000004000569, -5.349999999999999645, -7.500000000000000000 ) ) ;
#56064=CARTESIAN_POINT ( 'NONE',  ( 10.43314899746000002, -5.167567567567999731, 6.822293592207000934 ) ) ;
#56079=ORIENTED_EDGE ( 'NONE', *, *, #32739, .F. ) ;
#56087=CARTESIAN_POINT ( 'NONE',  ( 9.381635378478234699, -2.862680139623721587, 8.816521241667800268 ) ) ;
#56091=CARTESIAN_POINT ( 'NONE',  ( 10.86133765299000054, -5.065201555913000142, -5.176815510448999902 ) ) ;
#56094=CARTESIAN_POINT ( 'NONE',  ( 10.68403590588000007, -5.436611040123999317, 8.578433628717998971 ) ) ;
#56108=CARTESIAN_POINT ( 'NONE',  ( 11.12341523360999851, -6.055729757550999182, 5.272785169106999348 ) ) ;
#56109=CARTESIAN_POINT ( 'NONE',  ( 9.048318768181994542, -5.133256012319003858, -6.341058004364997558 ) ) ;
#56110=ORIENTED_EDGE ( 'NONE', *, *, #52699, .T. ) ;
#56116=CARTESIAN_POINT ( 'NONE',  ( 9.898728259668697405, -2.762655044027092721, -6.942780202613654694 ) ) ;
#56123=CARTESIAN_POINT ( 'NONE',  ( 7.810726116476000236, -5.086048788582002267, 6.527219528731996512 ) ) ;
#56130=B_SPLINE_CURVE_WITH_KNOTS ( 'NONE', 3,
 ( #19011, #45248, #50481, #40336, #44571, #55386, #49440, #29528, #7838, #18329, #39653, #12389 ),
 .UNSPECIFIED., .F., .F.,
 ( 4, 2, 2, 2, 2, 4 ),
 ( 0.000000000000000000, 0.2499999999999972800, 0.3749999999999953926, 0.4374999999999937828, 0.4999999999999922284, 1.000000000000000000 ),
 .UNSPECIFIED. ) ;
#56132=CARTESIAN_POINT ( 'NONE',  ( 7.807254669145095249, -3.019363530874672463, 6.522727296858301216 ) ) ;
#56135=CARTESIAN_POINT ( 'NONE',  ( 10.06577346837133291, -5.100000000000000533, 6.304440313804915874 ) ) ;
#56143=CARTESIAN_POINT ( 'NONE',  ( 9.813358178091998951, -5.349400659402999914, 6.657024270273000255 ) ) ;
#56145=EDGE_CURVE ( 'NONE', #40213, #31317, #57665, .T. ) ;
#56147=CARTESIAN_POINT ( 'NONE',  ( 9.523691940378000709, -4.852736108563000528, 8.683927195503999386 ) ) ;
#56149=EDGE_LOOP ( 'NONE', ( #56459, #52275, #57975, #5492 ) ) ;
#56151=CARTESIAN_POINT ( 'NONE',  ( 10.99999196979000082, -2.861044734458999627E-13, 5.200284647344000995E-13 ) ) ;
#56156=CARTESIAN_POINT ( 'NONE',  ( 9.285188841453999586, -5.269672295101000437, 8.747824102203999530 ) ) ;
#56158=DIRECTION ( 'NONE',  ( 0.000000000000000000, 1.000000000000000000, 0.000000000000000000 ) ) ;
#56162=CARTESIAN_POINT ( 'NONE',  ( 9.766851002543001314, -2.832432432432000269, 6.822293592207000934 ) ) ;
#56164=PRODUCT ( 'Positive Post', 'Positive Post', '', ( #42123 ) ) ;
#56165=LINE ( 'NONE', #29619, #65132 ) ;
#56170=CARTESIAN_POINT ( 'NONE',  ( 6.953073139469000630, -9.233001678504999532, 5.200628701625999994 ) ) ;
#56180=CARTESIAN_POINT ( 'NONE',  ( 10.00074484908000194, -2.373896846742000299, -7.962434077545999855 ) ) ;
#56183=CARTESIAN_POINT ( 'NONE',  ( 9.643637503375364517, -2.635046513920903166, -6.405124639914539841 ) ) ;
#56185=EDGE_CURVE ( 'NONE', #15766, #34080, #3774, .T. ) ;
#56187=ADVANCED_FACE ( 'NONE', ( #68843 ), #51738, .T. ) ;
#56190=FACE_OUTER_BOUND ( 'NONE', #14203, .T. ) ;
#56193=FACE_OUTER_BOUND ( 'NONE', #5090, .T. ) ;
#56203=CARTESIAN_POINT ( 'NONE',  ( 8.181105646794000208, -5.485781663882000281, 8.532068390166999805 ) ) ;
#56208=ORIENTED_EDGE ( 'NONE', *, *, #54695, .T. ) ;
#56218=CARTESIAN_POINT ( 'NONE',  ( 9.500008250440000523, -2.279684233303000074, 7.877691491255999878 ) ) ;
#56222=CARTESIAN_POINT ( 'NONE',  ( 10.80374194038000013, -2.766944173105999827, -8.073385940268000383 ) ) ;
#56223=CARTESIAN_POINT ( 'NONE',  ( 7.936743961419510995, -2.283396912964382075, 7.784033659319036680 ) ) ;
#56225=CARTESIAN_POINT ( 'NONE',  ( 10.37373728961999930, -2.215269876326000364, 7.703982265807999497 ) ) ;
#56228=ORIENTED_EDGE ( 'NONE', *, *, #29225, .F. ) ;
#56229=CARTESIAN_POINT ( 'NONE',  ( 10.85561138062999831, -5.068915657236000349, -5.151427698297999846 ) ) ;
#56238=ADVANCED_FACE ( 'NONE', ( #25170 ), #15026, .T. ) ;
#56244=VERTEX_POINT ( 'NONE', #46505 ) ;
#56246=CARTESIAN_POINT ( 'NONE',  ( 8.700644353210000403, -5.212258818969000451, 6.157189191035000064 ) ) ;
#56252=CARTESIAN_POINT ( 'NONE',  ( 10.88760685321000032, -5.634843745609000365, -7.088991614236999972 ) ) ;
#56264=CARTESIAN_POINT ( 'NONE',  ( 9.433148997456999751, -5.167567567567999731, 6.822293592207000934 ) ) ;
#56273=CARTESIAN_POINT ( 'NONE',  ( 10.29214449041784007, -3.170483834885368779, -8.579383242755033834 ) ) ;
#56274=EDGE_CURVE ( 'NONE', #606, #64705, #51341, .T. ) ;
#56289=AXIS2_PLACEMENT_3D ( 'NONE', #47719, #10644, #21144 ) ;
#56292=ADVANCED_FACE ( 'NONE', ( #26210 ), #50191, .T. ) ;
#56294=CARTESIAN_POINT ( 'NONE',  ( 9.459504440379001622, -5.445226602819000838, 7.703375344019999460 ) ) ;
#56307=CARTESIAN_POINT ( 'NONE',  ( 8.437855646795000553, -2.606998386752999775, 6.345764833140000505 ) ) ;
#56311=CARTESIAN_POINT ( 'NONE',  ( 10.98768472633000037, -6.720753151621999599, -5.471698430863999540 ) ) ;
#56322=CARTESIAN_POINT ( 'NONE',  ( 9.649875981547200610, -2.700874656649667749, 7.923553693498007533 ) ) ;
#56323=CARTESIAN_POINT ( 'NONE',  ( 10.50084194037999907, -4.616788958496999662, -6.288071994190999270 ) ) ;
#56341=CARTESIAN_POINT ( 'NONE',  ( 11.12914445903999905, -3.083861519183999977, 8.586004431109000024 ) ) ;
#56348=CARTESIAN_POINT ( 'NONE',  ( 11.01815802025999957, -6.613253574126999546, -5.429988750868999681 ) ) ;
#56354=CARTESIAN_POINT ( 'NONE',  ( 10.33537187819000103, -5.153689638257000105, 8.830861236101000600 ) ) ;
#56355=ORIENTED_EDGE ( 'NONE', *, *, #69128, .F. ) ;
#56365=VECTOR ( 'NONE', #53299, 1000.000000000000114 ) ;
#56366=B_SPLINE_SURFACE_WITH_KNOTS ( 'NONE', 3, 3, ( 
 ( #38418, #16741, #33182, #17444, #32495, #28280, #11160, #16402, #43674, #65674, #6600, #32157, #1361, #5908, #329, #48222, #44023, #38069, #48571, #54151, #6248, #27248, #675, #21643, #42978, #11844, #64285, #27942, #37388, #65326, #22335, #54500, #49600, #44376, #38771 ),
 ( #59395, #49252, #60095, #12201, #33529, #11495, #6947, #64971, #37732, #17086, #54848, #32839, #10815, #23026, #53473, #58711, #21987, #59743, #26908, #5567, #56225, #67049, #60438, #18829, #2738, #12545, #7640, #50296, #17796, #13590, #18137, #66708, #24064, #55542, #39460 ),
 ( #39115, #7295, #18482, #13247, #45398, #45739, #19158, #50638, #33876, #40155, #34222, #29678, #55193, #3078, #2394, #61130, #8334, #60780, #44717, #49947, #66014, #40482, #50980, #23718, #61471, #24411, #12894, #28635, #2060, #34910, #28988, #45054, #66361, #39807, #23378 ),
 ( #55888, #34572, #7992, #29325, #904, #55074, #43900, #48795, #22217, #44258, #43553, #32717, #64506, #44604, #11376, #27468, #64854, #65554, #1941, #23260, #53694, #33062, #27828, #33759, #60319, #18025, #12428, #49477, #28161, #1588, #16963, #65204, #49828, #6829, #11045 ) ),
 .UNSPECIFIED., .F., .F., .F.,
 ( 4, 4 ),
 ( 4, 1, 1, 1, 1, 1, 1, 1, 1, 1, 1, 1, 1, 1, 1, 1, 1, 1, 1, 1, 1, 1, 1, 1, 1, 1, 1, 1, 1, 1, 1, 1, 4 ),
 ( -0.1039086239011999951, 1.103908623900999864 ),
 ( -0.01933701211302999920, 0.01208563257065999909, 0.04350827725433999843, 0.07493092193802000645, 0.1063535666217000075, 0.1377762113054000204, 0.1691988559891000055, 0.2006215006727000150, 0.2320441453564000001, 0.2634667900400999851, 0.2948894347238000258, 0.3263120794074999553, 0.3577347240911999959, 0.3891573687748000054, 0.4205800134584999905, 0.4520026581421999756, 0.4834253028259000162, 0.5148479475096000568, 0.5462705921932000663, 0.5776932368768999959, 0.6091158815606000365, 0.6405385262443000771, 0.6719611709280000067, 0.7033838156117000473, 0.7348064602953000568, 0.7662291049789999864, 0.7976517496627000270, 0.8290743943464000676, 0.8604970390300999972, 0.8919196837138000378, 0.9233423283974000473, 0.9547649730810999769, 0.9861876177648000175 ),
 .UNSPECIFIED. ) ;
#56370=DIRECTION ( 'NONE',  ( 4.886316779972976613E-08, -0.7071067643484966192, -0.7071067980245964169 ) ) ;
#56375=CARTESIAN_POINT ( 'NONE',  ( 11.09999999999999964, -0.5000000000000000000, -5.124965750789000296 ) ) ;
#56383=CIRCLE ( 'NONE', #578, 1.100000000000000755 ) ;
#56384=CARTESIAN_POINT ( 'NONE',  ( 9.600494040286998043, -5.206548117663999165, 8.585114612872999373 ) ) ;
#56387=DIRECTION ( 'NONE',  ( 0.000000000000000000, 1.000000000000000000, 0.000000000000000000 ) ) ;
#56398=CARTESIAN_POINT ( 'NONE',  ( 9.749327024990000368, -5.634417356902000407, -7.003562403358999156 ) ) ;
#56403=CARTESIAN_POINT ( 'NONE',  ( 8.970944094206998898, -5.100000000000000533, 6.571291218949999902 ) ) ;
#56410=CARTESIAN_POINT ( 'NONE',  ( 9.344204180665373727, -2.685408982705638881, -7.853404758885505821 ) ) ;
#56418=DIRECTION ( 'NONE',  ( 1.000000000000000000, 0.000000000000000000, 0.000000000000000000 ) ) ;
#56434=EDGE_CURVE ( 'NONE', #6003, #46630, #56903, .T. ) ;
#56435=CARTESIAN_POINT ( 'NONE',  ( 8.350387243830999395, -4.599999999999999645, 6.632262360512000576 ) ) ;
#56436=EDGE_CURVE ( 'NONE', #35557, #45838, #19845, .T. ) ;
#56440=CYLINDRICAL_SURFACE ( 'NONE', #6178, 1.350000000000000089 ) ;
#56443=CARTESIAN_POINT ( 'NONE',  ( 10.34521071928999980, -2.724119865955000108, 6.497322598008000050 ) ) ;
#56445=CARTESIAN_POINT ( 'NONE',  ( 10.91944543538999923, -3.268376408192000149, -6.413937436229999456 ) ) ;
#56449=CARTESIAN_POINT ( 'NONE',  ( 10.76685100253999927, -2.832432432432000269, 6.822293592207000934 ) ) ;
#56457=CARTESIAN_POINT ( 'NONE',  ( 8.619872774977997310, -4.492752443836998566, -6.440200355240005337 ) ) ;
#56459=ORIENTED_EDGE ( 'NONE', *, *, #25281, .F. ) ;
#56464=CARTESIAN_POINT ( 'NONE',  ( 9.932908211424001266, -3.485164486501000081, -6.221839249167999242 ) ) ;
#56466=FACE_OUTER_BOUND ( 'NONE', #48516, .T. ) ;
#56474=VERTEX_POINT ( 'NONE', #47448 ) ;
#56487=ORIENTED_EDGE ( 'NONE', *, *, #27709, .F. ) ;
#56488=CARTESIAN_POINT ( 'NONE',  ( 10.40516264833000015, -5.216401621862000404, 6.765753642936999768 ) ) ;
#56490=CARTESIAN_POINT ( 'NONE',  ( 9.454580538893289088, -5.254250442392512710, 7.998733024362086219 ) ) ;
#56493=EDGE_CURVE ( 'NONE', #39811, #30230, #37223, .T. ) ;
#56494=ORIENTED_EDGE ( 'NONE', *, *, #11669, .F. ) ;
#56495=CARTESIAN_POINT ( 'NONE',  ( 10.52717528972000061, -8.216420183534999921, 6.728173953305000232 ) ) ;
#56496=CARTESIAN_POINT ( 'NONE',  ( 11.06622274902693093, -4.530851388958180515, -8.944471867880441351 ) ) ;
#56500=ORIENTED_EDGE ( 'NONE', *, *, #10025, .F. ) ;
#56501=CARTESIAN_POINT ( 'NONE',  ( 10.34020413671000149, -4.202027362542999356, 9.459588031742001135 ) ) ;
#56509=VECTOR ( 'NONE', #42726, 1000.000000000000000 ) ;
#56510=CARTESIAN_POINT ( 'NONE',  ( 10.93448722448066768, -2.832483728680937674, -6.743831965299308173 ) ) ;
#56518=ADVANCED_FACE ( 'NONE', ( #63853 ), #64882, .T. ) ;
#56523=EDGE_CURVE ( 'NONE', #48331, #31044, #2194, .T. ) ;
#56525=CARTESIAN_POINT ( 'NONE',  ( 11.11264194660999927, -2.146089039267000231, -7.517188649391000510 ) ) ;
#56545=CARTESIAN_POINT ( 'NONE',  ( 7.101308059622001068, -3.554853390786000045, 8.889491623367000273 ) ) ;
#56557=ORIENTED_EDGE ( 'NONE', *, *, #67967, .F. ) ;
#56562=CARTESIAN_POINT ( 'NONE',  ( 8.832537864289999874, -2.899999999999999911, 6.571291218949999902 ) ) ;
#56565=CARTESIAN_POINT ( 'NONE',  ( 10.95519194037999888, -3.860335380237000180, -6.147338954930000376 ) ) ;
#56566=APPLICATION_CONTEXT ( 'automotive_design' ) ;
#56568=CARTESIAN_POINT ( 'NONE',  ( 8.252728345141258970, -5.371128151206209900, 8.571272383222918734 ) ) ;
#56580=CARTESIAN_POINT ( 'NONE',  ( 9.666315108303999537, -3.197530835772000035, -8.817973615970998935 ) ) ;
#56581=DIRECTION ( 'NONE',  ( 1.000000000000000000, 5.572913924281000893E-12, -1.887560193303999882E-10 ) ) ;
#56587=B_SPLINE_CURVE_WITH_KNOTS ( 'NONE', 3,
 ( #58083, #15774, #32212, #37104 ),
 .UNSPECIFIED., .F., .F.,
 ( 4, 4 ),
 ( 0.8566590321960471099, 1.000000000000000000 ),
 .UNSPECIFIED. ) ;
#56590=CARTESIAN_POINT ( 'NONE',  ( 8.341918146793998901, -5.601799093797000140, 7.176147756900999930 ) ) ;
#56595=CARTESIAN_POINT ( 'NONE',  ( 10.59956814679000026, -4.438148200474000937, -8.958389257466000899 ) ) ;
#56611=AXIS2_PLACEMENT_3D ( 'NONE', #2169, #7399, #28045 ) ;
#56629=VECTOR ( 'NONE', #14466, 1000.000000000000000 ) ;
#56634=CARTESIAN_POINT ( 'NONE',  ( 10.88166120451243124, -2.855160512203144485, 8.850519483704566426 ) ) ;
#56636=CARTESIAN_POINT ( 'NONE',  ( 5.599999999588999522, 0.000000000000000000, 0.000000000000000000 ) ) ;
#56639=VERTEX_POINT ( 'NONE', #38678 ) ;
#56648=PLANE ( 'NONE',  #64514 ) ;
#56649=CARTESIAN_POINT ( 'NONE',  ( 7.988543146792999927, -3.566638198986999964, 5.743608852252999775 ) ) ;
#56650=ORIENTED_EDGE ( 'NONE', *, *, #18898, .T. ) ;
#56656=CARTESIAN_POINT ( 'NONE',  ( 7.793461047962999544, -3.207862402212000141, 6.406748704942000217 ) ) ;
#56664=EDGE_CURVE ( 'NONE', #46950, #16623, #67182, .T. ) ;
#56674=CARTESIAN_POINT ( 'NONE',  ( 11.01511860815784871, -5.215118608160429048, 6.608919745756069553 ) ) ;
#56676=EDGE_LOOP ( 'NONE', ( #19912, #4095, #19852, #12520, #51705 ) ) ;
#56687=CARTESIAN_POINT ( 'NONE',  ( 10.85068991645999859, -4.478102922274999287, 6.162028334171000488 ) ) ;
#56689=CIRCLE ( 'NONE', #26534, 1.449999999999999956 ) ;
#56690=CARTESIAN_POINT ( 'NONE',  ( 10.87695483801000051, -5.827068285690999438, -7.814745128155998977 ) ) ;
#56708=CARTESIAN_POINT ( 'NONE',  ( -15.86200481174999943, -5.599999999999999645, -6.571291218949999902 ) ) ;
#56717=EDGE_CURVE ( 'NONE', #34080, #53919, #66315, .T. ) ;
#56720=FACE_OUTER_BOUND ( 'NONE', #64890, .T. ) ;
#56729=VECTOR ( 'NONE', #14862, 1000.000000000000000 ) ;
#56731=B_SPLINE_CURVE_WITH_KNOTS ( 'NONE', 3,
 ( #38687, #3259, #29513, #32755 ),
 .UNSPECIFIED., .F., .F.,
 ( 4, 4 ),
 ( 0.000000000000000000, 0.3058164706682733325 ),
 .UNSPECIFIED. ) ;
#56732=CARTESIAN_POINT ( 'NONE',  ( 10.40727044253999978, -3.797905333157999941, 5.889909992361999969 ) ) ;
#56737=CARTESIAN_POINT ( 'NONE',  ( 11.09999999999999964, -4.000000000000000000, 7.500000000000000000 ) ) ;
#56739=ORIENTED_EDGE ( 'NONE', *, *, #13632, .F. ) ;
#56741=CARTESIAN_POINT ( 'NONE',  ( 10.66823071782296672, -5.044756569124447587, -5.053267171664180601 ) ) ;
#56745=CARTESIAN_POINT ( 'NONE',  ( 8.714021517297007691, -3.496029227938000972, -6.351413116489997179 ) ) ;
#56747=CARTESIAN_POINT ( 'NONE',  ( 9.573320215454998561, -2.624754973437999794, -6.486841649805000110 ) ) ;
#56760=CARTESIAN_POINT ( 'NONE',  ( 9.312955771054708620, -2.920709800291079627, -8.329395787248037308 ) ) ;
#56762=ORIENTED_EDGE ( 'NONE', *, *, #51955, .F. ) ;
#56768=CARTESIAN_POINT ( 'NONE',  ( 11.09999999999999964, -1.300000000000000044, 9.662944685757000940 ) ) ;
#56776=EDGE_CURVE ( 'NONE', #64065, #51247, #14200, .T. ) ;
#56786=ORIENTED_EDGE ( 'NONE', *, *, #48715, .F. ) ;
#56811=CARTESIAN_POINT ( 'NONE',  ( 9.749152735436000583, -5.239375073306999475, -6.095351682555999240 ) ) ;
#56815=CARTESIAN_POINT ( 'NONE',  ( 11.04829169656000154, -5.240875637261000364, 5.064311916315999973 ) ) ;
#56827=ORIENTED_EDGE ( 'NONE', *, *, #29167, .F. ) ;
#56838=CARTESIAN_POINT ( 'NONE',  ( 10.37026726325999881, -5.571557883540000589, 7.748386351620999868 ) ) ;
#56840=CYLINDRICAL_SURFACE ( 'NONE', #68584, 0.4999999999999998335 ) ;
#56841=CARTESIAN_POINT ( 'NONE',  ( 8.149355646792999508, -2.583664704444999849, 6.684748541034000624 ) ) ;
#56845=CARTESIAN_POINT ( 'NONE',  ( 11.01333310117525954, -5.463772421450651784, -7.751599404490038481 ) ) ;
#56848=CARTESIAN_POINT ( 'NONE',  ( 8.194123395920479780, -2.898248195268428251, 6.620168246131465928 ) ) ;
#56854=CARTESIAN_POINT ( 'NONE',  ( 10.90635170712999980, -3.089674976714000376, -6.534319251717000121 ) ) ;
#56860=CARTESIAN_POINT ( 'NONE',  ( 10.13706886426420084, -2.899999999999999911, 6.444141223280826836 ) ) ;
#56871=CARTESIAN_POINT ( 'NONE',  ( 10.04002603384999937, -2.348908096685999869, -7.136751747961000092 ) ) ;
#56872=DIRECTION ( 'NONE',  ( 1.000000000000000000, 0.000000000000000000, 0.000000000000000000 ) ) ;
#56878=CARTESIAN_POINT ( 'NONE',  ( 8.335879440378999305, -4.310353212080000773, 9.459493062793997709 ) ) ;
#56891=CARTESIAN_POINT ( 'NONE',  ( 7.614808059621999803, -3.326257819185999942, 8.794522506294001118 ) ) ;
#56900=DIRECTION ( 'NONE',  ( 1.000000000000000000, 0.000000000000000000, 0.000000000000000000 ) ) ;
#56901=CARTESIAN_POINT ( 'NONE',  ( 11.00000000000000000, -5.200000000000000178, 5.865766984179000332 ) ) ;
#56903=LINE ( 'NONE', #35922, #62293 ) ;
#56910=CARTESIAN_POINT ( 'NONE',  ( 8.256279407735984677, -5.320103330200151248, 8.633016269157472777 ) ) ;
#56914=CARTESIAN_POINT ( 'NONE',  ( 10.72098219424000121, -5.042358674275999597, -5.112202241721999663 ) ) ;
#56916=ORIENTED_EDGE ( 'NONE', *, *, #11258, .T. ) ;
#56918=ORIENTED_EDGE ( 'NONE', *, *, #12102, .T. ) ;
#56919=CARTESIAN_POINT ( 'NONE',  ( 9.793154437819998392, -5.792391408692000532, -6.955579396894000510 ) ) ;
#56922=B_SPLINE_CURVE_WITH_KNOTS ( 'NONE', 3,
 ( #35526, #18416, #45674, #50226 ),
 .UNSPECIFIED., .F., .F.,
 ( 4, 4 ),
 ( 0.000000000000000000, 1.000000000000000000 ),
 .UNSPECIFIED. ) ;
#56930=CARTESIAN_POINT ( 'NONE',  ( 9.278331853207999913, -5.791549888895000109, 7.752110689268000954 ) ) ;
#56937=CARTESIAN_POINT ( 'NONE',  ( 10.86460564679000029, -3.843601288168000174, -5.985268170611000471 ) ) ;
#56947=CARTESIAN_POINT ( 'NONE',  ( 10.88508678867000157, -5.158304027353000087, 5.065542421513000271 ) ) ;
#56955=CARTESIAN_POINT ( 'NONE',  ( 10.16712151127301667, -5.079456268609191305, -8.329490867415614730 ) ) ;
#56992=CARTESIAN_POINT ( 'NONE',  ( 11.08729972629000038, -2.258669075224000178, -7.034582301298999418 ) ) ;
#56993=CARTESIAN_POINT ( 'NONE',  ( 7.468789704280648145, -2.309885600679958628, 7.088095784442930203 ) ) ;
#57003=B_SPLINE_CURVE_WITH_KNOTS ( 'NONE', 3,
 ( #45234, #54676, #38594, #28465 ),
 .UNSPECIFIED., .F., .F.,
 ( 4, 4 ),
 ( 0.000000000000000000, 1.000000000000000000 ),
 .UNSPECIFIED. ) ;
#57007=CARTESIAN_POINT ( 'NONE',  ( 10.97601622864088178, -5.224113188238077576, 6.768286317869557145 ) ) ;
#57011=DIRECTION ( 'NONE',  ( 0.4384236320213996119, -0.6355252626312996034, -0.6355252626312996034 ) ) ;
#57013=ORIENTED_EDGE ( 'NONE', *, *, #26350, .T. ) ;
#57020=CARTESIAN_POINT ( 'NONE',  ( 7.204907196771999978, -0.2999999999999999889, -3.099954730132999714 ) ) ;
#57022=CARTESIAN_POINT ( 'NONE',  ( 9.757667269575000191, -4.489271889653999814, 5.986031004145000445 ) ) ;
#57024=CARTESIAN_POINT ( 'NONE',  ( 10.13061232742999884, -2.189322372303999842, -7.101642112140999608 ) ) ;
#57034=FACE_OUTER_BOUND ( 'NONE', #41786, .T. ) ;
#57049=CARTESIAN_POINT ( 'NONE',  ( 9.751909913808001207, -4.316974633926000671, -5.653758079558000027 ) ) ;
#57050=EDGE_CURVE ( 'NONE', #20897, #44819, #13828, .T. ) ;
#57071=CARTESIAN_POINT ( 'NONE',  ( 10.65520300221153782, -5.038713246137302981, -5.049010194981326194 ) ) ;
#57074=CARTESIAN_POINT ( 'NONE',  ( 8.385191233021004109, -3.508000636384001947, -6.669203184159004039 ) ) ;
#57078=CARTESIAN_POINT ( 'NONE',  ( 11.13107481686000177, -2.674997213776999949, -5.007806838190000498 ) ) ;
#57079=CARTESIAN_POINT ( 'NONE',  ( 10.79702055961999818, -5.792859009854000263, -7.049265738992000152 ) ) ;
#57088=CARTESIAN_POINT ( 'NONE',  ( 9.229626678759569103, -4.176630817665263784, -8.850101115164489940 ) ) ;
#57098=EDGE_CURVE ( 'NONE', #19018, #65197, #1868, .T. ) ;
#57101=LINE ( 'NONE', #20045, #56629 ) ;
#57103=ORIENTED_EDGE ( 'NONE', *, *, #4519, .F. ) ;
#57111=CARTESIAN_POINT ( 'NONE',  ( 5.699999999877000789, -1.433333330872999856, 10.65401593578999950 ) ) ;
#57114=CARTESIAN_POINT ( 'NONE',  ( 7.000000000000000000, -7.526486366024999874, -3.526486366024999874 ) ) ;
#57116=CARTESIAN_POINT ( 'NONE',  ( 8.101999744244276158, -3.171054102886327719, 8.579047487217421164 ) ) ;
#57128=EDGE_CURVE ( 'NONE', #1282, #5900, #48732, .T. ) ;
#57129=EDGE_CURVE ( 'NONE', #49363, #61047, #52065, .T. ) ;
#57130=CARTESIAN_POINT ( 'NONE',  ( 8.191498616105999275, -3.399962740672999750, 6.146646623957999545 ) ) ;
#57139=CARTESIAN_POINT ( 'NONE',  ( 11.09999999999999964, -6.593648102827000201, 5.598803487171999826 ) ) ;
#57140=CARTESIAN_POINT ( 'NONE',  ( 9.927742433789001453, -5.651611919872999934, -7.935921913274999184 ) ) ;
#57147=CARTESIAN_POINT ( 'NONE',  ( 8.079287380335998137, -4.920039154826996608, 6.237958006931995314 ) ) ;
#57157=CARTESIAN_POINT ( 'NONE',  ( 7.250690656965701031, -4.000034976101444428, 9.109408410636810061 ) ) ;
#57159=CARTESIAN_POINT ( 'NONE',  ( 9.637068864299580540, -2.899999999999999911, 6.444141223381762096 ) ) ;
#57162=DIRECTION ( 'NONE',  ( 0.000000000000000000, 0.000000000000000000, -1.000000000000000000 ) ) ;
#57165=VECTOR ( 'NONE', #6648, 1000.000000000000114 ) ;
#57167=CARTESIAN_POINT ( 'NONE',  ( 9.646285452541999206, -2.591464128784999765, 6.760053199270999791 ) ) ;
#57170=CARTESIAN_POINT ( 'NONE',  ( 9.459504440379001622, -5.445226602819000838, 7.703375344019999460 ) ) ;
#57173=ORIENTED_EDGE ( 'NONE', *, *, #45626, .F. ) ;
#57184=VERTEX_POINT ( 'NONE', #53970 ) ;
#57191=CARTESIAN_POINT ( 'NONE',  ( 7.871384613761001070, -5.129340912189999990, 6.740051747100999968 ) ) ;
#57203=CARTESIAN_POINT ( 'NONE',  ( 9.038695689765509300, -4.943520148687432503, 8.465362812019415983 ) ) ;
#57217=CARTESIAN_POINT ( 'NONE',  ( 9.136976429976712666, -5.100000000000000533, 6.167827406373843857 ) ) ;
#57221=CARTESIAN_POINT ( 'NONE',  ( 8.192495559623999668, -2.550228841911000188, 7.666975032000999946 ) ) ;
#57226=B_SPLINE_CURVE_WITH_KNOTS ( 'NONE', 3,
 ( #18424, #61067, #13185, #56162 ),
 .UNSPECIFIED., .F., .F.,
 ( 4, 4 ),
 ( 0.8746679733675616353, 1.000000000000000000 ),
 .UNSPECIFIED. ) ;
#57231=ORIENTED_EDGE ( 'NONE', *, *, #52985, .F. ) ;
#57238=CARTESIAN_POINT ( 'NONE',  ( 7.847822007142403855, -5.059730379935329481, 6.600780866611749786 ) ) ;
#57240=CARTESIAN_POINT ( 'NONE',  ( 8.286427776887917318, -4.793419134848132757, 9.047669286253999132 ) ) ;
#57244=CARTESIAN_POINT ( 'NONE',  ( 10.94668920802000045, -5.066629281208999913, -5.177964064427999169 ) ) ;
#57248=VERTEX_POINT ( 'NONE', #12717 ) ;
#57250=CARTESIAN_POINT ( 'NONE',  ( 5.699999999554000496, -0.3000000004460000036, 9.662944681662999358 ) ) ;
#57252=EDGE_CURVE ( 'NONE', #23757, #67334, #11937, .T. ) ;
#57259=MECHANICAL_DESIGN_GEOMETRIC_PRESENTATION_REPRESENTATION('',(#62845),#23788);
#57265=CARTESIAN_POINT ( 'NONE',  ( 10.18308064679000147, -2.953580299898999950, -8.606287508253000595 ) ) ;
#57274=ORIENTED_EDGE ( 'NONE', *, *, #21522, .T. ) ;
#57276=( NAMED_UNIT ( * ) SI_UNIT ( $, .STERADIAN. ) SOLID_ANGLE_UNIT ( ) );
#57286=VERTEX_POINT ( 'NONE', #23199 ) ;
#57294=EDGE_CURVE ( 'NONE', #33561, #66341, #68782, .T. ) ;
#57314=CARTESIAN_POINT ( 'NONE',  ( 10.21194365307746743, -5.865446360225381461, 7.794835729825335235 ) ) ;
#57318=CARTESIAN_POINT ( 'NONE',  ( 7.716851002542999716, -2.832432432432000269, 6.822293592207000934 ) ) ;
#57323=CARTESIAN_POINT ( 'NONE',  ( 7.758191940376999440, -5.797088532631000213, 8.340479314546998424 ) ) ;
#57324=ORIENTED_EDGE ( 'NONE', *, *, #54353, .T. ) ;
#57327=CARTESIAN_POINT ( 'NONE',  ( 10.57314899745999881, -5.167567567567999731, -6.822293592207000934 ) ) ;
#57328=CARTESIAN_POINT ( 'NONE',  ( 7.623314959413727721, -5.001887204095511130, 6.074294720979810158 ) ) ;
#57353=CARTESIAN_POINT ( 'NONE',  ( 10.07101719722999889, -4.042170815906999337, 8.920201479886998186 ) ) ;
#57368=CARTESIAN_POINT ( 'NONE',  ( 9.520803773887999810, -3.270557529354000348, 5.711489293131999823 ) ) ;
#57400=DIRECTION ( 'NONE',  ( 1.000000000000000000, 0.000000000000000000, 0.000000000000000000 ) ) ;
#57412=CARTESIAN_POINT ( 'NONE',  ( 8.914818027809994661, -3.440065392353999663, -6.172246220506001357 ) ) ;
#57417=CARTESIAN_POINT ( 'NONE',  ( 10.53198305961999992, -2.323723769066000422, -8.279488812962998878 ) ) ;
#57432=CARTESIAN_POINT ( 'NONE',  ( 8.496516550600020423, -5.350579948490476134, 7.852800305270212000 ) ) ;
#57441=VECTOR ( 'NONE', #24495, 1000.000000000000000 ) ;
#57443=ORIENTED_EDGE ( 'NONE', *, *, #48697, .F. ) ;
#57458=LINE ( 'NONE', #30227, #55928 ) ;
#57459=CARTESIAN_POINT ( 'NONE',  ( 10.17310292480999934, -4.709171320598000143, -8.664883863910000983 ) ) ;
#57471=CARTESIAN_POINT ( 'NONE',  ( 7.909525359152002721, -3.174976509417001491, 6.234240719816002141 ) ) ;
#57475=CARTESIAN_POINT ( 'NONE',  ( 11.09999999999999964, -5.555182244517999912, 5.124965749841000395 ) ) ;
#57479=CARTESIAN_POINT ( 'NONE',  ( 10.95304521165000011, -5.154933323944999479, 5.180455670148000458 ) ) ;
#57494=CARTESIAN_POINT ( 'NONE',  ( 8.866178911608058044, -2.879880053984696264, -6.717471171832306354 ) ) ;
#57495=VERTEX_POINT ( 'NONE', #52868 ) ;
#57496=CYLINDRICAL_SURFACE ( 'NONE', #19888, 0.5000000000000002220 ) ;
#57503=CARTESIAN_POINT ( 'NONE',  ( 11.14993998249000029, -2.627133311863999676, 6.696092388640000337 ) ) ;
#57505=CARTESIAN_POINT ( 'NONE',  ( 7.559808771084921553, -3.823091902406630549, 8.850087896820790334 ) ) ;
#57506=CARTESIAN_POINT ( 'NONE',  ( 9.021581853209999835, -2.193670085072000120, 7.400591740205000768 ) ) ;
#57515=B_SPLINE_CURVE_WITH_KNOTS ( 'NONE', 3,
 ( #21721, #59132, #21047, #47279, #32573, #21384, #53885, #5987, #15799, #27325, #31892, #52512, #26646, #22065, #57753, #61, #4612, #25946 ),
 .UNSPECIFIED., .F., .F.,
 ( 4, 2, 2, 2, 2, 2, 2, 2, 4 ),
 ( 0.1254138569076999055, 0.2190601518424659111, 0.3127064467772319167, 0.4063527417119979224, 0.4999990366467639280, 0.5936453315815299892, 0.6872916265162959393, 0.7809379214510618894, 0.8745842163858279505 ),
 .UNSPECIFIED. ) ;
#57516=LINE ( 'NONE', #51930, #6325 ) ;
#57518=CARTESIAN_POINT ( 'NONE',  ( 8.156860996257041307, -3.022118299483437021, 6.361385428469135128 ) ) ;
#57520=CARTESIAN_POINT ( 'NONE',  ( 9.657547180956999711, -5.333447643521000536, 6.049925825719999928 ) ) ;
#57521=EDGE_CURVE ( 'NONE', #46365, #6210, #21241, .T. ) ;
#57525=CARTESIAN_POINT ( 'NONE',  ( 10.85290698989999925, -3.170384785323999921, -8.782188229854000383 ) ) ;
#57527=ORIENTED_EDGE ( 'NONE', *, *, #30618, .T. ) ;
#57539=EDGE_LOOP ( 'NONE', ( #32490, #41620, #64211, #68255 ) ) ;
#57542=CARTESIAN_POINT ( 'NONE',  ( 5.700000000000000178, 0.000000000000000000, 0.000000000000000000 ) ) ;
#57546=B_SPLINE_CURVE_WITH_KNOTS ( 'NONE', 3,
 ( #39966, #61283, #13399, #50795 ),
 .UNSPECIFIED., .F., .F.,
 ( 4, 4 ),
 ( 0.000000000000000000, 1.000000000000000000 ),
 .UNSPECIFIED. ) ;
#57547=CARTESIAN_POINT ( 'NONE',  ( 5.700000000000000178, 0.000000000000000000, 0.000000000000000000 ) ) ;
#57569=CARTESIAN_POINT ( 'NONE',  ( 7.058516392956000196, -4.314043295739000250, 8.819145559946001356 ) ) ;
#57585=CARTESIAN_POINT ( 'NONE',  ( 8.128369806614207604, -5.084382722290230916, 6.139741310093872251 ) ) ;
#57588=CARTESIAN_POINT ( 'NONE',  ( 10.33538764829999934, -4.566957278416999166, -4.713742776521000266 ) ) ;
#57594=ORIENTED_EDGE ( 'NONE', *, *, #35059, .F. ) ;
#57595=CARTESIAN_POINT ( 'NONE',  ( 9.416972128128000108, -4.783349162191000481, -6.231236652334000148 ) ) ;
#57599=CARTESIAN_POINT ( 'NONE',  ( 8.624846738991013950, -5.035341376712734629, 6.089196183450023447 ) ) ;
#57604=EDGE_LOOP ( 'NONE', ( #43775, #15550, #42121, #56355, #45217, #18602, #45596, #2644, #3863, #29850, #4114, #13763 ) ) ;
#57607=CARTESIAN_POINT ( 'NONE',  ( 9.059370559623998176, -4.192917962110999319, 5.525484568403999930 ) ) ;
#57612=CARTESIAN_POINT ( 'NONE',  ( 10.75101814679000078, -2.478465696309000155, -7.438303690845000204 ) ) ;
#57622=DIRECTION ( 'NONE',  ( 1.000000000000000000, 0.000000000000000000, 0.000000000000000000 ) ) ;
#57624=SURFACE_SIDE_STYLE ('',( #40519 ) ) ;
#57625=DIRECTION ( 'NONE',  ( 0.000000000000000000, -0.9510199984508466153, 0.3091293621553143911 ) ) ;
#57633=CARTESIAN_POINT ( 'NONE',  ( 10.61341493184000129, -5.180137390751999860, -4.762641710075000034 ) ) ;
#57634=ORIENTED_EDGE ( 'NONE', *, *, #1261, .T. ) ;
#57640=LINE ( 'NONE', #23510, #660 ) ;
#57650=CARTESIAN_POINT ( 'NONE',  ( 10.97051713369074655, -2.309060732479470079, 7.058091048960522862 ) ) ;
#57665=LINE ( 'NONE', #63248, #22107 ) ;
#57666=CARTESIAN_POINT ( 'NONE',  ( 7.577019353207000485, -5.480312458445999901, 8.192326492433998908 ) ) ;
#57671=CARTESIAN_POINT ( 'NONE',  ( 7.642454705974068396, -5.316671649445813053, 6.363707368334387660 ) ) ;
#57693=CARTESIAN_POINT ( 'NONE',  ( 7.890669427268998781, -4.660296165433000404, 6.322498843348999920 ) ) ;
#57695=VECTOR ( 'NONE', #66126, 1000.000000000000114 ) ;
#57699=CARTESIAN_POINT ( 'NONE',  ( 9.966331042021000286, -2.304002513595999613, 6.575636708208000059 ) ) ;
#57708=CYLINDRICAL_SURFACE ( 'NONE', #3456, 1.350000000000000089 ) ;
#57714=CARTESIAN_POINT ( 'NONE',  ( 9.242349231304000767, -5.206700957550999931, 8.808818370147001531 ) ) ;
#57722=CARTESIAN_POINT ( 'NONE',  ( 9.786673210037999837, -2.381198102024000285, 7.612749732462000374 ) ) ;
#57727=DIRECTION ( 'NONE',  ( 0.000000000000000000, -1.000000000000000000, 0.000000000000000000 ) ) ;
#57753=CARTESIAN_POINT ( 'NONE',  ( 9.773267324721318872, -2.820167152981252645, -8.180006241673510203 ) ) ;
#57760=CARTESIAN_POINT ( 'NONE',  ( 11.13506629761000077, -2.665575611901000119, -5.176677555269999509 ) ) ;
#57761=CARTESIAN_POINT ( 'NONE',  ( 11.15264435320999858, -2.317067032475999877, -7.596564138533999255 ) ) ;
#57762=CARTESIAN_POINT ( 'NONE',  ( 9.153455117183082024, -2.649843614532905178, 7.852866721134374117 ) ) ;
#57783=B_SPLINE_CURVE_WITH_KNOTS ( 'NONE', 3,
 ( #38261, #864, #38612, #39922 ),
 .UNSPECIFIED., .F., .F.,
 ( 4, 4 ),
 ( 0.000000000000000000, 1.000000000000000000 ),
 .UNSPECIFIED. ) ;
#57785=ORIENTED_EDGE ( 'NONE', *, *, #9730, .T. ) ;
#57803=CARTESIAN_POINT ( 'NONE',  ( 9.783240866989459050, -5.333689009038027784, -6.342574321089660572 ) ) ;
#57809=CARTESIAN_POINT ( 'NONE',  ( 9.949439740260999088, -2.508493821066999807, -7.171861383782999866 ) ) ;
#57810=VERTEX_POINT ( 'NONE', #62493 ) ;
#57812=VECTOR ( 'NONE', #53045, 999.9999999999998863 ) ;
#57817=CARTESIAN_POINT ( 'NONE',  ( 10.76947109217999810, -5.100000000000000533, -6.152188490330000370 ) ) ;
#57821=CARTESIAN_POINT ( 'NONE',  ( 7.782404085375001834, -2.843788791114000958, 6.809963588862000705 ) ) ;
#57824=CARTESIAN_POINT ( 'NONE',  ( 7.782975328289005290, -3.196931270636999667, 6.293200827887002191 ) ) ;
#57829=CARTESIAN_POINT ( 'NONE',  ( 10.12549839661999940, -5.788806995403000144, 7.335561828691000485 ) ) ;
#57835=CARTESIAN_POINT ( 'NONE',  ( 8.185765847591000011, -4.942196905450001232, 6.196983455206997782 ) ) ;
#57843=EDGE_LOOP ( 'NONE', ( #4143, #63717, #32090, #1156, #21411 ) ) ;
#57849=DIRECTION ( 'NONE',  ( 1.000000000000000000, 0.000000000000000000, 0.000000000000000000 ) ) ;
#57851=FACE_OUTER_BOUND ( 'NONE', #55766, .T. ) ;
#57861=CARTESIAN_POINT ( 'NONE',  ( 9.966331042021000286, -2.304002513595999613, 6.575636708208000059 ) ) ;
#57863=CARTESIAN_POINT ( 'NONE',  ( 9.453819884702960863, -5.259191288891824634, 7.986286180968190429 ) ) ;
#57864=CARTESIAN_POINT ( 'NONE',  ( 8.636456853209999451, -3.869396851328000153, 5.695656592546999519 ) ) ;
#57869=CARTESIAN_POINT ( 'NONE',  ( 10.97843137008999825, -5.235400103863000254, 6.782920672145000829 ) ) ;
#57875=CARTESIAN_POINT ( 'NONE',  ( 9.124702828701000357, -4.778665285493000070, 8.799745834808000211 ) ) ;
#57879=LINE ( 'NONE', #14889, #42605 ) ;
#57885=PLANE ( 'NONE',  #5334 ) ;
#57889=CARTESIAN_POINT ( 'NONE',  ( 10.73930809942999964, -2.762991917822000154, 6.801028165221000066 ) ) ;
#57909=CARTESIAN_POINT ( 'NONE',  ( 8.977754440379998258, -2.019079883662000086, 7.390983468784999566 ) ) ;
#57920=DIRECTION ( 'NONE',  ( 0.000000000000000000, -1.000000000000000000, 0.000000000000000000 ) ) ;
#57923=CARTESIAN_POINT ( 'NONE',  ( 7.283516392955999841, -4.426925773067000414, 9.293310812901001583 ) ) ;
#57924=CARTESIAN_POINT ( 'NONE',  ( 8.860769353209001054, -2.935738482289000029, 6.259841087764999479 ) ) ;
#57927=CARTESIAN_POINT ( 'NONE',  ( 9.129428851719998406, -5.099284414202999827, 6.151604790022999758 ) ) ;
#57928=ORIENTED_EDGE ( 'NONE', *, *, #3488, .T. ) ;
#57937=CARTESIAN_POINT ( 'NONE',  ( 10.85738557828999973, -2.754556666341999804, 8.976367391363998749 ) ) ;
#57940=DIRECTION ( 'NONE',  ( -0.5298945028670929425, -2.005738535499974775E-09, -0.8480635682725891078 ) ) ;
#57942=CARTESIAN_POINT ( 'NONE',  ( 8.224446432042114452, -5.652657913853214033, 8.042967277513600521 ) ) ;
#57952=CARTESIAN_POINT ( 'NONE',  ( 9.844904806657000407, -2.626678530444999993, -7.387134320497999340 ) ) ;
#57962=CARTESIAN_POINT ( 'NONE',  ( 8.353308059623998361, -2.800111029801999774, 9.079936276749000612 ) ) ;
#57963=CARTESIAN_POINT ( 'NONE',  ( 11.04782425406999913, -5.235403588978999601, 5.041461677707999911 ) ) ;
#57973=CARTESIAN_POINT ( 'NONE',  ( 9.766851002543001314, -2.832432432432000269, 6.822293592207000934 ) ) ;
#57975=ORIENTED_EDGE ( 'NONE', *, *, #51859, .F. ) ;
#57982=CARTESIAN_POINT ( 'NONE',  ( 10.60519595724999853, -5.343977295764999802, -7.731524081231999190 ) ) ;
#57985=B_SPLINE_CURVE_WITH_KNOTS ( 'NONE', 3,
 ( #52526, #25961, #62666, #25269 ),
 .UNSPECIFIED., .F., .F.,
 ( 4, 4 ),
 ( 0.000000000000000000, 0.1254223444949154886 ),
 .UNSPECIFIED. ) ;
#57998=CARTESIAN_POINT ( 'NONE',  ( 8.893204545404998385, -3.399999999998999822, -6.188268997420999007 ) ) ;
#57999=B_SPLINE_CURVE_WITH_KNOTS ( 'NONE', 3,
 ( #28059, #7069, #1482, #22799, #6025, #65448, #43098, #16179, #32614, #12321, #33652, #54269, #22451, #64747, #27026 ),
 .UNSPECIFIED., .F., .F.,
 ( 4, 2, 2, 2, 1, 2, 2, 4 ),
 ( 0.000000000000000000, 0.5000000000000474065, 0.6250000000000575096, 0.6875000000000628386, 0.7187500000000658362, 0.7343750000000649480, 0.7500000000000640599, 1.000000000000000000 ),
 .UNSPECIFIED. ) ;
#58002=CARTESIAN_POINT ( 'NONE',  ( 9.192135076938702909, -2.763579744383045433, 8.048932413616332937 ) ) ;
#58003=ORIENTED_EDGE ( 'NONE', *, *, #64394, .F. ) ;
#58014=CARTESIAN_POINT ( 'NONE',  ( 10.43470728713959161, -2.143801129421504470, 7.848344630244035613 ) ) ;
#58023=CARTESIAN_POINT ( 'NONE',  ( 9.250897313459001126, -4.135077143711000325, 9.175520401071999288 ) ) ;
#58027=CARTESIAN_POINT ( 'NONE',  ( 10.22514748322304534, -2.649941783575446408, 7.500008211948054004 ) ) ;
#58028=CARTESIAN_POINT ( 'NONE',  ( 10.75915805961999894, -5.387268372866000021, -6.278119777966000292 ) ) ;
#58029=VECTOR ( 'NONE', #53293, 1000.000000000000000 ) ;
#58030=CARTESIAN_POINT ( 'NONE',  ( 7.566932968645870616, -3.846483248383185227, 5.765333662263238956 ) ) ;
#58041=CARTESIAN_POINT ( 'NONE',  ( 8.893204545404998385, -3.399999999998999822, -6.188268997420999007 ) ) ;
#58046=CARTESIAN_POINT ( 'NONE',  ( 10.36503728015203230, -2.650011783303574564, -7.500002219258004921 ) ) ;
#58053=CARTESIAN_POINT ( 'NONE',  ( 10.47253786429000044, -2.899999999999999911, -6.571291218949999902 ) ) ;
#58056=CARTESIAN_POINT ( 'NONE',  ( 10.33537187819000103, -5.153689638257000105, 8.830861236101000600 ) ) ;
#58071=B_SPLINE_CURVE_WITH_KNOTS ( 'NONE', 3,
 ( #59961, #897, #39335, #54023 ),
 .UNSPECIFIED., .F., .F.,
 ( 4, 4 ),
 ( 0.000000000000000000, 1.000000000000000000 ),
 .UNSPECIFIED. ) ;
#58072=CARTESIAN_POINT ( 'NONE',  ( 9.242197237618364980, -2.679953703640003404, 7.218470457551299901 ) ) ;
#58078=AXIS2_PLACEMENT_3D ( 'NONE', #32856, #33202, #42993 ) ;
#58079=CARTESIAN_POINT ( 'NONE',  ( 10.99433452212999818, -3.697619272994999928, 5.729306330972000261 ) ) ;
#58083=CARTESIAN_POINT ( 'NONE',  ( 7.725062132959652494, -2.650631715052233162, 7.500008390440855877 ) ) ;
#58085=CARTESIAN_POINT ( 'NONE',  ( 9.399896294736999280, -5.679455740088000582, -8.329752476417999318 ) ) ;
#58097=CARTESIAN_POINT ( 'NONE',  ( 10.87522165821000009, -4.831071966430999787, 6.312786525516999703 ) ) ;
#58109=EDGE_CURVE ( 'NONE', #1971, #36315, #44541, .T. ) ;
#58116=DIRECTION ( 'NONE',  ( -1.000000000000000000, 0.000000000000000000, -2.893429392030000019E-14 ) ) ;
#58129=EDGE_LOOP ( 'NONE', ( #29363, #22682, #22082, #1363 ) ) ;
#58158=CARTESIAN_POINT ( 'NONE',  ( 10.29094647910999782, -2.903513699412000104, -8.310923036409999298 ) ) ;
#58160=ORIENTED_EDGE ( 'NONE', *, *, #13606, .T. ) ;
#58162=CARTESIAN_POINT ( 'NONE',  ( 10.21685100254000034, -2.832432432432000269, 6.822293592207000934 ) ) ;
#58167=EDGE_CURVE ( 'NONE', #66560, #22085, #45666, .T. ) ;
#58171=CARTESIAN_POINT ( 'NONE',  ( 10.27733372368999909, -3.426503291345000424, 5.004059351583000748 ) ) ;
#58172=CARTESIAN_POINT ( 'NONE',  ( 8.228217774218997249, -3.441349337319001389, 6.127431371819001882 ) ) ;
#58177=CARTESIAN_POINT ( 'NONE',  ( 5.599999999976000176, -7.849276784099999367E-14, -1.865174681369999824E-14 ) ) ;
#58178=CARTESIAN_POINT ( 'NONE',  ( 10.62197618263000010, -5.779779175739000685, 7.256573549370999743 ) ) ;
#58191=CARTESIAN_POINT ( 'NONE',  ( 8.232750256041883929, -4.666560802762334426, 6.122829837889073978 ) ) ;
#58192=CARTESIAN_POINT ( 'NONE',  ( 9.433148997456999751, -5.167567567567999731, 6.822293592207000934 ) ) ;
#58203=CARTESIAN_POINT ( 'NONE',  ( 9.520803773887999810, -3.270557529354000348, 5.711489293131999823 ) ) ;
#58207=CARTESIAN_POINT ( 'NONE',  ( 9.047980646795000581, -2.806079842068999852, 8.615883328687999665 ) ) ;
#58214=CARTESIAN_POINT ( 'NONE',  ( 8.170084059452333847, -3.293748801396804371, 6.167716128177580970 ) ) ;
#58216=CARTESIAN_POINT ( 'NONE',  ( 11.18051369187999988, -5.340070732632000272, 8.416150632189001612 ) ) ;
#58230=EDGE_CURVE ( 'NONE', #26679, #57184, #33632, .T. ) ;
#58248=CARTESIAN_POINT ( 'NONE',  ( 7.410855646792000151, -2.302293129340000188, 6.875167727519000849 ) ) ;
#58253=EDGE_CURVE ( 'NONE', #49595, #32140, #58627, .T. ) ;
#58259=EDGE_LOOP ( 'NONE', ( #67490, #43274, #41550, #24758 ) ) ;
#58260=CARTESIAN_POINT ( 'NONE',  ( 8.251331853209000755, -5.773185758034999893, 7.141496747382000798 ) ) ;
#58274=CARTESIAN_POINT ( 'NONE',  ( 7.954963149567436886, -4.950001034494477814, 6.428732759487574278 ) ) ;
#58279=CARTESIAN_POINT ( 'NONE',  ( 8.541367865291375594, -3.305226939453190127, 5.905633504331038175 ) ) ;
#58288=CARTESIAN_POINT ( 'NONE',  ( 9.536892889968999754, -5.099406281193999746, -6.669356233738001016 ) ) ;
#58294=ORIENTED_EDGE ( 'NONE', *, *, #66043, .F. ) ;
#58299=CARTESIAN_POINT ( 'NONE',  ( 8.802620559624999785, -3.975070057433999438, 9.483761758588999058 ) ) ;
#58308=ADVANCED_FACE ( 'NONE', ( #25357 ), #56840, .T. ) ;
#58318=CARTESIAN_POINT ( 'NONE',  ( 11.09999999999999964, -2.649999999999999911, 7.500000000000000000 ) ) ;
#58338=ORIENTED_EDGE ( 'NONE', *, *, #52874, .F. ) ;
#58341=CARTESIAN_POINT ( 'NONE',  ( 11.00448450226549113, -2.648588503021471308, 6.387884280188352193 ) ) ;
#58349=EDGE_CURVE ( 'NONE', #25195, #41892, #11080, .T. ) ;
#58354=ORIENTED_EDGE ( 'NONE', *, *, #21431, .T. ) ;
#58359=CARTESIAN_POINT ( 'NONE',  ( 8.218894353209000414, -3.011617647609999615, 8.801438026873999121 ) ) ;
#58363=CARTESIAN_POINT ( 'NONE',  ( 10.72129555961999792, -4.673507771948999689, -5.778404201896999659 ) ) ;
#58364=CARTESIAN_POINT ( 'NONE',  ( 7.593455520019030125, -4.408259056465409387, 5.809061053540682806 ) ) ;
#58365=VECTOR ( 'NONE', #58116, 1000.000000000000000 ) ;
#58368=VERTEX_POINT ( 'NONE', #67998 ) ;
#58384=CARTESIAN_POINT ( 'NONE',  ( 10.32992855215000105, -4.904916250652000542, 4.624355442463000010 ) ) ;
#58390=CARTESIAN_POINT ( 'NONE',  ( 9.799258316471000541, -4.057329063942999525, 9.430691159271001212 ) ) ;
#58396=EDGE_CURVE ( 'NONE', #35557, #29557, #14434, .T. ) ;
#58408=ORIENTED_EDGE ( 'NONE', *, *, #60102, .F. ) ;
#58412=EDGE_CURVE ( 'NONE', #40911, #6003, #67784, .T. ) ;
#58413=CARTESIAN_POINT ( 'NONE',  ( 9.261668853699999815, -2.944250413017999612, 6.507387951280999339 ) ) ;
#58428=B_SPLINE_CURVE_WITH_KNOTS ( 'NONE', 3,
 ( #57130, #42431, #51880, #25316 ),
 .UNSPECIFIED., .F., .F.,
 ( 4, 4 ),
 ( 0.000000000000000000, 1.000000000000000000 ),
 .UNSPECIFIED. ) ;
#58437=EDGE_CURVE ( 'NONE', #46332, #53670, #39441, .T. ) ;
#58452=CYLINDRICAL_SURFACE ( 'NONE', #68042, 1.350000000000000089 ) ;
#58479=( BOUNDED_SURFACE ( )  B_SPLINE_SURFACE ( 3, 3, ( 
 ( #63465, #67675, #37254, #41471, #35880, #30638, #51948, #41129, #69066 ),
 ( #25043, #26078, #62778, #62441, #47756, #20830, #21172, #14562, #15922 ),
 ( #25384, #46722, #15242, #58573, #30302, #51609, #3704, #36916, #46375 ),
 ( #10335, #31671, #9642, #68366, #41811, #28146, #43883, #59952, #17305 ) ),
 .UNSPECIFIED., .F., .F., .T. ) 
 B_SPLINE_SURFACE_WITH_KNOTS ( ( 4, 4 ),
 ( 4, 1, 1, 1, 1, 1, 4 ),
 ( 0.000000000000000000, 1.000000000000000000 ),
 ( 0.8657679006235999841, 0.8794646334505999974, 0.9056938526918999477, 0.9344431701380999655, 0.9658387281735000274, 1.000000000000000000, 1.004641266558000012 ),
 .UNSPECIFIED. ) 
 GEOMETRIC_REPRESENTATION_ITEM ( )  RATIONAL_B_SPLINE_SURFACE ( (
 ( 1.157353709788000007, 1.157353709788000007, 1.157353709788000007, 1.157353709788000007, 1.157353709788000007, 1.157353709788000007, 1.157353709788000007, 1.157353709788000007, 1.157353709788000007),
 ( 0.9475487634039000406, 0.9475487634039000406, 0.9475487634039000406, 0.9475487634039000406, 0.9475487634039000406, 0.9475487634039000406, 0.9475487634039000406, 0.9475487634039000406, 0.9475487634039000406),
 ( 0.9475487634039000406, 0.9475487634039000406, 0.9475487634039000406, 0.9475487634039000406, 0.9475487634039000406, 0.9475487634039000406, 0.9475487634039000406, 0.9475487634039000406, 0.9475487634039000406),
 ( 1.157353709788000007, 1.157353709788000007, 1.157353709788000007, 1.157353709788000007, 1.157353709788000007, 1.157353709788000007, 1.157353709788000007, 1.157353709788000007, 1.157353709788000007) ) ) 
 REPRESENTATION_ITEM ( '' )  SURFACE ( )  );
#58481=ORIENTED_EDGE ( 'NONE', *, *, #39850, .T. ) ;
#58486=B_SPLINE_SURFACE_WITH_KNOTS ( 'NONE', 3, 3, ( 
 ( #15866, #21120, #69007, #27060, #37198, #42445, #52585, #32646, #31963, #53620, #63754, #52935, #10620, #5717, #37534, #27398, #11309, #42787, #53958, #59205, #26369, #47696, #43130, #41756, #6061, #5380, #53279, #5030, #48373, #48031, #58516, #63410, #21797, #48727, #26719 ),
 ( #63057, #137, #31613, #21451, #64096, #829, #482, #15534, #64435, #16557, #16210, #15184, #58865, #10971, #36508, #9937, #57829, #36858, #20773, #32310, #37885, #31274, #47349, #4678, #58178, #26020, #68655, #42105, #10280, #60594, #65129, #54657, #17250, #6407, #44182 ),
 ( #55005, #2216, #39271, #7800, #12701, #29140, #28443, #34038, #60941, #55350, #7447, #49066, #50447, #12354, #28799, #33687, #60252, #23187, #1517, #65481, #43486, #55702, #44872, #23531, #50110, #11653, #59897, #43830, #66176, #38225, #59553, #7106, #1174, #32988, #18296 ),
 ( #13057, #17954, #54304, #39618, #27754, #22487, #17605, #49757, #1867, #38573, #64783, #38930, #34385, #12005, #6752, #44533, #65827, #22146, #16896, #33342, #28092, #49405, #22836, #34727, #8831, #18640, #61288, #8489, #18979, #20010, #46585, #67203, #30172, #24570, #56037 ) ),
 .UNSPECIFIED., .F., .F., .F.,
 ( 4, 4 ),
 ( 4, 1, 1, 1, 1, 1, 1, 1, 1, 1, 1, 1, 1, 1, 1, 1, 1, 1, 1, 1, 1, 1, 1, 1, 1, 1, 1, 1, 1, 1, 1, 1, 4 ),
 ( -0.1039086239011999951, 1.103908623900999864 ),
 ( -0.01933701211302999920, 0.01208563257065999909, 0.04350827725433999843, 0.07493092193802000645, 0.1063535666217000075, 0.1377762113054000204, 0.1691988559891000055, 0.2006215006727000150, 0.2320441453564000001, 0.2634667900400999851, 0.2948894347238000258, 0.3263120794074999553, 0.3577347240911999959, 0.3891573687748000054, 0.4205800134584999905, 0.4520026581421999756, 0.4834253028259000162, 0.5148479475096000568, 0.5462705921932000663, 0.5776932368768999959, 0.6091158815606000365, 0.6405385262443000771, 0.6719611709280000067, 0.7033838156117000473, 0.7348064602953000568, 0.7662291049789999864, 0.7976517496627000270, 0.8290743943464000676, 0.8604970390300999972, 0.8919196837138000378, 0.9233423283974000473, 0.9547649730810999769, 0.9861876177648000175 ),
 .UNSPECIFIED. ) ;
#58498=CARTESIAN_POINT ( 'NONE',  ( 10.26368921839999970, -4.794141574281000295, -8.804455889106000299 ) ) ;
#58502=CARTESIAN_POINT ( 'NONE',  ( 8.616995677562000466, -4.876077402042000131, 5.996974966533000106 ) ) ;
#58504=CARTESIAN_POINT ( 'NONE',  ( 7.000000000000000000, -7.526486366024999874, -3.526486366024999874 ) ) ;
#58508=CARTESIAN_POINT ( 'NONE',  ( 10.27506785289999947, -3.374327226904999755, 5.003467443561000039 ) ) ;
#58510=ORIENTED_EDGE ( 'NONE', *, *, #68687, .T. ) ;
#58513=CARTESIAN_POINT ( 'NONE',  ( 7.684934563448005740, -2.928065616737000720, 6.508603912219004251 ) ) ;
#58514=CARTESIAN_POINT ( 'NONE',  ( 9.712899699504999873, -4.008306780893000187, -8.877926425468999128 ) ) ;
#58516=CARTESIAN_POINT ( 'NONE',  ( 11.08492081570999943, -3.668392767032000013, 5.558160538745999801 ) ) ;
#58528=CARTESIAN_POINT ( 'NONE',  ( 10.08728840308773300, -2.899999999999999911, -6.305985889617788942 ) ) ;
#58533=CARTESIAN_POINT ( 'NONE',  ( 7.652389431507828910, -3.170862826441127158, 8.579327016467345857 ) ) ;
#58541=CARTESIAN_POINT ( 'NONE',  ( 10.22399006116000031, -5.507891002176999784, 6.589804341508000540 ) ) ;
#58543=B_SPLINE_CURVE_WITH_KNOTS ( 'NONE', 3,
 ( #3992, #56116, #3651, #45973, #50877 ),
 .UNSPECIFIED., .F., .F.,
 ( 4, 1, 4 ),
 ( 0.000000000000000000, 0.1250503395655981342, 0.2125974459517032678 ),
 .UNSPECIFIED. ) ;
#58546=CARTESIAN_POINT ( 'NONE',  ( 8.957394353210000659, -2.678334737187000325, 8.735278777293000729 ) ) ;
#58554=CARTESIAN_POINT ( 'NONE',  ( 10.40727044253999978, -3.797905333157999941, 5.889909992361999969 ) ) ;
#58573=CARTESIAN_POINT ( 'NONE',  ( 7.802608290491005683, -4.876635182444005068, 6.352765399118998069 ) ) ;
#58584=CARTESIAN_POINT ( 'NONE',  ( 8.881777890044364909, -4.415113854800245541, -6.197856508860001057 ) ) ;
#58592=CARTESIAN_POINT ( 'NONE',  ( 8.373668146795001377, -2.202816532622999812, 7.706987678916999762 ) ) ;
#58594=CARTESIAN_POINT ( 'NONE',  ( 10.33253786428999987, -2.899999999999999911, 6.571291218949999902 ) ) ;
#58603=CARTESIAN_POINT ( 'NONE',  ( 8.187144353207999714, -4.968144979409999884, 5.971795951526999602 ) ) ;
#58607=ORIENTED_EDGE ( 'NONE', *, *, #18706, .T. ) ;
#58614=ADVANCED_FACE ( 'NONE', ( #60279 ), #61312, .F. ) ;
#58623=CARTESIAN_POINT ( 'NONE',  ( 8.412003453006938969, -2.446741332449001494, 8.282553572544875564 ) ) ;
#58627=B_SPLINE_CURVE_WITH_KNOTS ( 'NONE', 3,
 ( #45998, #20455, #9266, #13850, #9614, #24679, #41782, #67310, #63087, #29945, #42135, #8595 ),
 .UNSPECIFIED., .F., .F.,
 ( 4, 2, 2, 2, 2, 4 ),
 ( 0.000000000000000000, 0.2499999999999976130, 0.3749999999999962252, 0.4374999999999957256, 0.4999999999999952260, 1.000000000000000000 ),
 .UNSPECIFIED. ) ;
#58629=EDGE_LOOP ( 'NONE', ( #9137, #61830, #59853, #52982 ) ) ;
#58631=CARTESIAN_POINT ( 'NONE',  ( 4.000000000000000000, 0.000000000000000000, 0.000000000000000000 ) ) ;
#58658=ORIENTED_EDGE ( 'NONE', *, *, #18365, .T. ) ;
#58659=CARTESIAN_POINT ( 'NONE',  ( -2.147830119999999621, -1.300000000000000044, 9.662944685757000940 ) ) ;
#58666=CARTESIAN_POINT ( 'NONE',  ( 10.88016425062000003, -2.793121555136000023, -6.864957546339999439 ) ) ;
#58672=ORIENTED_EDGE ( 'NONE', *, *, #67550, .F. ) ;
#58683=ORIENTED_EDGE ( 'NONE', *, *, #34201, .T. ) ;
#58685=FACE_OUTER_BOUND ( 'NONE', #46232, .T. ) ;
#58692=CARTESIAN_POINT ( 'NONE',  ( 10.16571249083272654, -5.659096789895665225, 6.739882715535322255 ) ) ;
#58703=CARTESIAN_POINT ( 'NONE',  ( 9.625489929093001606, -3.134630999349000025, 8.626959345509000343 ) ) ;
#58704=CARTESIAN_POINT ( 'NONE',  ( 8.604019353210000887, -5.165500668528999917, 8.645534272955000432 ) ) ;
#58707=B_SPLINE_CURVE_WITH_KNOTS ( 'NONE', 3,
 ( #6269, #12223, #33550, #48938, #48240, #38441, #23047, #27963, #27610, #58730, #1046, #11864, #49272, #59077 ),
 .UNSPECIFIED., .F., .F.,
 ( 4, 2, 2, 2, 2, 2, 4 ),
 ( 0.000000000000000000, 0.1249999999999999722, 0.2499999999999999445, 0.4999999999999993339, 0.6249999999999994449, 0.7499999999999996669, 1.000000000000000000 ),
 .UNSPECIFIED. ) ;
#58709=CARTESIAN_POINT ( 'NONE',  ( 10.50898185320999900, -4.485028460808000439, -9.114431591966999591 ) ) ;
#58710=CARTESIAN_POINT ( 'NONE',  ( 7.772509392072763035, -5.050159846104850914, 8.886365745317096554 ) ) ;
#58711=CARTESIAN_POINT ( 'NONE',  ( 10.06343867337000120, -5.156226070197000411, 6.125223053176999777 ) ) ;
#58727=CARTESIAN_POINT ( 'NONE',  ( 8.992847592598998574, -5.108134449482000683, -6.664326587025001025 ) ) ;
#58730=CARTESIAN_POINT ( 'NONE',  ( 10.01008022827853772, -3.057295994144781037, -8.976432196558560506 ) ) ;
#58735=CARTESIAN_POINT ( 'NONE',  ( 10.94797187187000098, -2.864324950622999744, 8.846246404612999825 ) ) ;
#58745=VECTOR ( 'NONE', #43162, 1000.000000000000000 ) ;
#58749=CARTESIAN_POINT ( 'NONE',  ( 9.225036374688860619, -2.649952446100997339, 7.500002253091946791 ) ) ;
#58779=EDGE_CURVE ( 'NONE', #31672, #65921, #28688, .T. ) ;
#58793=CARTESIAN_POINT ( 'NONE',  ( 10.44728840309080020, -2.899999999999999911, 6.305985889617041984 ) ) ;
#58798=CARTESIAN_POINT ( 'NONE',  ( 10.56170564679000101, -5.057490041178001050, -8.595713413570999606 ) ) ;
#58801=CARTESIAN_POINT ( 'NONE',  ( 11.03776785110999903, -5.237767851104999650, 6.571291218949999902 ) ) ;
#58807=ORIENTED_EDGE ( 'NONE', *, *, #62223, .T. ) ;
#58808=AXIS2_PLACEMENT_3D ( 'NONE', #56901, #4434, #26118 ) ;
#58818=CARTESIAN_POINT ( 'NONE',  ( 10.36950884864999978, -2.719121019997000399, -7.031782724641000293 ) ) ;
#58841=CARTESIAN_POINT ( 'NONE',  ( 10.02800210979000184, -3.452027005875999865, -6.074520565702999697 ) ) ;
#58844=ORIENTED_EDGE ( 'NONE', *, *, #51525, .F. ) ;
#58847=DIRECTION ( 'NONE',  ( 0.000000000000000000, 1.000000000000000000, 0.000000000000000000 ) ) ;
#58855=CARTESIAN_POINT ( 'NONE',  ( 8.268606633798000871, -2.876811830795998670, 6.331441650266997456 ) ) ;
#58858=CARTESIAN_POINT ( 'NONE',  ( 9.905786073958001481, -2.698967003257000119, 8.979227319929000473 ) ) ;
#58865=CARTESIAN_POINT ( 'NONE',  ( 9.877259503622999759, -2.207992199716000137, 7.624813542847999059 ) ) ;
#58868=EDGE_CURVE ( 'NONE', #11696, #518, #45272, .T. ) ;
#58877=CARTESIAN_POINT ( 'NONE',  ( 9.972537864286000087, -2.899999999999999911, -6.571291218949999902 ) ) ;
#58892=VECTOR ( 'NONE', #24588, 1000.000000000000000 ) ;
#58893=CARTESIAN_POINT ( 'NONE',  ( 10.24478558459999888, -5.265199116477000452, 8.959495174640998982 ) ) ;
#58897=CARTESIAN_POINT ( 'NONE',  ( 8.032370559622998840, -3.524751762020000179, 5.573845465339999805 ) ) ;
#58907=CARTESIAN_POINT ( 'NONE',  ( 9.753140057121997941, -4.104977100659999323, 9.293279163877999238 ) ) ;
#58913=CARTESIAN_POINT ( 'NONE',  ( 10.31152944037999930, -2.716820959546999870, -7.950167805575999225 ) ) ;
#58922=AXIS2_PLACEMENT_3D ( 'NONE', #3026, #29967, #3700 ) ;
#58924=B_SPLINE_SURFACE_WITH_KNOTS ( 'NONE', 3, 3, ( 
 ( #14280, #30030, #49002, #35606, #56919, #24073, #19516, #40836, #17180, #55551, #43767, #24761, #40165, #3087, #13936, #38509, #62159, #51332, #8682 ),
 ( #60791, #66370, #50306, #61480, #45410, #12904, #45748, #2404, #27688, #46087, #34232, #29336, #67058, #66719, #50648, #35263, #7649, #67395, #28997 ),
 ( #18838, #19168, #23728, #39818, #45066, #13256, #34581, #13599, #40492, #34920, #61819, #56580, #25101, #26139, #63869, #35937, #36279, #57595, #68422 ),
 ( #42224, #31048, #9019, #30359, #41189, #14618, #41523, #53051, #51667, #57952, #41868, #46433, #36629, #9702, #31387, #52357, #58288, #10051, #52701 ) ),
 .UNSPECIFIED., .F., .F., .F.,
 ( 4, 4 ),
 ( 4, 1, 1, 1, 1, 1, 1, 1, 1, 1, 1, 1, 1, 1, 1, 1, 4 ),
 ( -0.1039086239011999951, 1.103908623900999864 ),
 ( -0.008849010032007000384, 0.01991027257200999809, 0.04866955517603999831, 0.07742883778006000306, 0.1061881203840999988, 0.1349474029881000126, 0.1637066855920999986, 0.1924659681960999846, 0.2212252508002000018, 0.2499845334042000156, 0.2787438160081999738, 0.3075030986121999876, 0.3362623812162000014, 0.3650216638202999908, 0.3937809464243000046, 0.4225402290282999629, 0.4512995116322999767 ),
 .UNSPECIFIED. ) ;
#58929=FACE_OUTER_BOUND ( 'NONE', #55459, .T. ) ;
#58940=CARTESIAN_POINT ( 'NONE',  ( 7.641206853206999661, -4.524489047957000132, 9.047757046927999980 ) ) ;
#58951=VERTEX_POINT ( 'NONE', #12814 ) ;
#58952=CARTESIAN_POINT ( 'NONE',  ( 8.315519353208999931, -5.485781663882000281, 8.532068390166999805 ) ) ;
#58965=CARTESIAN_POINT ( 'NONE',  ( 10.36409408021999923, -3.399999909169000301, -4.954046131279000065 ) ) ;
#58971=B_SPLINE_CURVE_WITH_KNOTS ( 'NONE', 3,
 ( #25522, #46850, #42632, #68154, #37384, #20273 ),
 .UNSPECIFIED., .F., .F.,
 ( 4, 2, 4 ),
 ( 0.000000000000000000, 0.3470917641979919255, 0.6941835283959838510 ),
 .UNSPECIFIED. ) ;
#58974=CARTESIAN_POINT ( 'NONE',  ( 8.319350023656893356, -4.124618607633898648, 9.242618487877578559 ) ) ;
#58981=EDGE_CURVE ( 'NONE', #48042, #47885, #28116, .T. ) ;
#58986=CARTESIAN_POINT ( 'NONE',  ( 11.07508065833999922, -8.038176207971000409, 6.929846776222000848 ) ) ;
#58987=CARTESIAN_POINT ( 'NONE',  ( 9.803754904607863807, -2.991223623039768853, -8.479528301168882010 ) ) ;
#58991=ORIENTED_EDGE ( 'NONE', *, *, #43001, .T. ) ;
#59006=DIRECTION ( 'NONE',  ( 1.000000000000000000, 0.000000000000000000, 0.000000000000000000 ) ) ;
#59015=CARTESIAN_POINT ( 'NONE',  ( 10.21685100254000034, -2.832432432432000269, 6.822293592207000934 ) ) ;
#59016=CARTESIAN_POINT ( 'NONE',  ( 8.767881343006999728, -4.605543323398999966, -6.293427432547999523 ) ) ;
#59026=AXIS2_PLACEMENT_3D ( 'NONE', #57542, #4739, #26083 ) ;
#59051=CARTESIAN_POINT ( 'NONE',  ( 10.68361719090999884, -2.603550124652000086, 7.762065570229999878 ) ) ;
#59052=CARTESIAN_POINT ( 'NONE',  ( 8.411456853209999807, -3.882020254083999866, 5.870054788755000530 ) ) ;
#59056=CARTESIAN_POINT ( 'NONE',  ( 9.991527686541001430, -4.805948463426999773, -8.932428271061001013 ) ) ;
#59057=CARTESIAN_POINT ( 'NONE',  ( 7.739691844317393432, -5.527372948754030624, 8.333565270828541927 ) ) ;
#59058=FACE_OUTER_BOUND ( 'NONE', #7440, .T. ) ;
#59060=ORIENTED_EDGE ( 'NONE', *, *, #706, .F. ) ;
#59065=ORIENTED_EDGE ( 'NONE', *, *, #10436, .F. ) ;
#59073=ORIENTED_EDGE ( 'NONE', *, *, #45108, .F. ) ;
#59074=CARTESIAN_POINT ( 'NONE',  ( 8.432504440379000599, -5.430412429559000387, 7.210798766422999329 ) ) ;
#59077=CARTESIAN_POINT ( 'NONE',  ( 9.934999999999998721, -4.640430492595999823, -9.117542781427999898 ) ) ;
#59082=CARTESIAN_POINT ( 'NONE',  ( 10.05691733561000056, -2.453480799114999833, 6.657106310117000270 ) ) ;
#59097=CARTESIAN_POINT ( 'NONE',  ( 9.070985106021000277, -8.666611253863997888, -6.095301607234000052 ) ) ;
#59102=CARTESIAN_POINT ( 'NONE',  ( 8.174990947233128580, -2.650692654197974729, 7.500004443805800669 ) ) ;
#59103=CARTESIAN_POINT ( 'NONE',  ( 9.882266086202999844, -4.932716797830999589, 6.390980246320999925 ) ) ;
#59122=CARTESIAN_POINT ( 'NONE',  ( 9.674373738639999942, -2.899999999999999911, -6.185493860157000867 ) ) ;
#59132=CARTESIAN_POINT ( 'NONE',  ( 9.575345697731034278, -5.349773134808791575, -7.676679544872200722 ) ) ;
#59139=CARTESIAN_POINT ( 'NONE',  ( 10.94033064679000233, -5.142732045902000948, -6.493502833853999512 ) ) ;
#59141=DIRECTION ( 'NONE',  ( -0.7071067811865974218, 0.7071067811864975017, 9.304588036591961259E-09 ) ) ;
#59156=CARTESIAN_POINT ( 'NONE',  ( 8.725348536223782148, -2.649439212887072959, 7.500023728975150128 ) ) ;
#59160=CARTESIAN_POINT ( 'NONE',  ( 9.898134631442999876, -2.965923230546999800, -6.610863544715000373 ) ) ;
#59165=B_SPLINE_CURVE_WITH_KNOTS ( 'NONE', 3,
 ( #68118, #37012, #67773, #68455, #20578, #62534, #31086, #10427, #36668, #4486, #41903, #47502 ),
 .UNSPECIFIED., .F., .F.,
 ( 4, 2, 2, 2, 2, 4 ),
 ( 0.000000000000000000, 0.2500000000000179301, 0.3750000000000234812, 0.4375000000000240363, 0.5000000000000245359, 1.000000000000000000 ),
 .UNSPECIFIED. ) ;
#59169=ORIENTED_EDGE ( 'NONE', *, *, #35794, .T. ) ;
#59174=EDGE_CURVE ( 'NONE', #30733, #31977, #24930, .T. ) ;
#59176=CARTESIAN_POINT ( 'NONE',  ( 10.79499900793999956, -3.503951165873000040, 6.168577387731000172 ) ) ;
#59187=CARTESIAN_POINT ( 'NONE',  ( 10.58996262057999971, -2.876743158681999812, -6.236533224899999617 ) ) ;
#59190=CARTESIAN_POINT ( 'NONE',  ( 5.700000001242999659, -1.249999998757000075, 1.883720477311000285E-09 ) ) ;
#59202=CARTESIAN_POINT ( 'NONE',  ( 10.52638330645999964, -2.451090818816000105, 6.282756943804999494 ) ) ;
#59205=CARTESIAN_POINT ( 'NONE',  ( 10.40226385995999969, -2.765692573780999641, 9.035345396600000356 ) ) ;
#59208=AXIS2_PLACEMENT_3D ( 'NONE', #53749, #9942, #63759 ) ;
#59213=DIRECTION ( 'NONE',  ( -0.000000000000000000, 1.000000000000000000, 0.000000000000000000 ) ) ;
#59217=EDGE_CURVE ( 'NONE', #1282, #49213, #4382, .T. ) ;
#59229=CARTESIAN_POINT ( 'NONE',  ( 10.57893103570000015, -4.649956431060000561, 5.681096060554999383 ) ) ;
#59232=CARTESIAN_POINT ( 'NONE',  ( 9.947288403111267385, -2.899999999999999911, 6.305985889562331970 ) ) ;
#59233=CARTESIAN_POINT ( 'NONE',  ( 9.216851002545999094, -2.832432432432000269, 6.822293592207000934 ) ) ;
#59241=CARTESIAN_POINT ( 'NONE',  ( 10.53138988903999973, -5.607755226963999640, 7.280101849877000042 ) ) ;
#59245=CARTESIAN_POINT ( 'NONE',  ( 10.52314899745999988, -5.167567567567999731, -6.822293592207000934 ) ) ;
#59246=CARTESIAN_POINT ( 'NONE',  ( 10.17270027370999941, -4.650151116117000605, -8.655526539784000661 ) ) ;
#59259=CARTESIAN_POINT ( 'NONE',  ( 9.326027934855707358, -3.975910976255049967, 9.239577797941210591 ) ) ;
#59266=FACE_OUTER_BOUND ( 'NONE', #36113, .T. ) ;
#59273=CARTESIAN_POINT ( 'NONE',  ( 7.246486640886755204, -2.683814467610606158, 7.146108783255461283 ) ) ;
#59276=CARTESIAN_POINT ( 'NONE',  ( 8.887168146795000112, -2.193670085072000120, 7.400591740205000768 ) ) ;
#59282=DIRECTION ( 'NONE',  ( 0.000000000000000000, -0.9906588508047033947, 0.1363636363636003546 ) ) ;
#59287=CARTESIAN_POINT ( 'NONE',  ( 8.919605646795000453, -5.165500668528999917, 8.645534272955000432 ) ) ;
#59290=DIRECTION ( 'NONE',  ( 0.000000000000000000, 0.000000000000000000, -1.000000000000000000 ) ) ;
#59308=B_SPLINE_CURVE_WITH_KNOTS ( 'NONE', 3,
 ( #57139, #20770, #30578, #46664, #63407, #57475, #21116 ),
 .UNSPECIFIED., .F., .F.,
 ( 4, 1, 1, 1, 4 ),
 ( 0.000000000000000000, 0.2500000143192999680, 0.5000000056314000130, 0.7499999969435999780, 1.000000000000000000 ),
 .UNSPECIFIED. ) ;
#59310=CARTESIAN_POINT ( 'NONE',  ( 8.540376343031317319, -3.285755531537955410, 5.914236678129165092 ) ) ;
#59321=ORIENTED_EDGE ( 'NONE', *, *, #28582, .F. ) ;
#59323=( LENGTH_UNIT ( ) NAMED_UNIT ( * ) SI_UNIT ( .MILLI., .METRE. ) );
#59334=ORIENTED_EDGE ( 'NONE', *, *, #8071, .T. ) ;
#59344=EDGE_CURVE ( 'NONE', #12470, #67865, #1132, .T. ) ;
#59349=CARTESIAN_POINT ( 'NONE',  ( 8.753601108637971251, -2.714205948350681297, 7.027810827039939312 ) ) ;
#59351=FACE_OUTER_BOUND ( 'NONE', #5595, .T. ) ;
#59359=CARTESIAN_POINT ( 'NONE',  ( 9.709999999999999076, -4.496968146123999865, -8.755198255949000696 ) ) ;
#59364=EDGE_CURVE ( 'NONE', #26163, #683, #1640, .T. ) ;
#59366=VECTOR ( 'NONE', #13865, 1000.000000000000114 ) ;
#59372=DIRECTION ( 'NONE',  ( -1.000000000000000000, 0.000000000000000000, 0.000000000000000000 ) ) ;
#59387=CARTESIAN_POINT ( 'NONE',  ( 11.07345355053000091, -3.998673159585000025, 8.920828114954002075 ) ) ;
#59392=CARTESIAN_POINT ( 'NONE',  ( 10.69829435321000055, -2.534030585780999711, -6.667788699001999220 ) ) ;
#59394=CARTESIAN_POINT ( 'NONE',  ( 7.806446110424286822, -4.398161847081256681, 9.193498077367777910 ) ) ;
#59395=CARTESIAN_POINT ( 'NONE',  ( 9.194602547868999665, -5.157768569202000108, 8.637845986715998237 ) ) ;
#59411=CARTESIAN_POINT ( 'NONE',  ( 9.138566940380000503, -2.933824946949000090, 8.496487880080000110 ) ) ;
#59422=CARTESIAN_POINT ( 'NONE',  ( 0.000000000000000000, -2.899999999999999911, 7.500000000000000000 ) ) ;
#59444=CARTESIAN_POINT ( 'NONE',  ( 9.634027193201999850, -3.042970193091000031, 8.588108172435999776 ) ) ;
#59479=EDGE_CURVE ( 'NONE', #50218, #24787, #13647, .T. ) ;
#59480=CARTESIAN_POINT ( 'NONE',  ( 10.17905590578999941, -2.899999999999999911, 6.571291218949999902 ) ) ;
#59481=CARTESIAN_POINT ( 'NONE',  ( 10.13035685320999946, -2.409329538444999752, -8.058042649154000259 ) ) ;
#59504=CARTESIAN_POINT ( 'NONE',  ( 9.792315001194999979, -4.284154785471999460, -9.000488933596999530 ) ) ;
#59507=EDGE_CURVE ( 'NONE', #61047, #52223, #9408, .T. ) ;
#59511=VECTOR ( 'NONE', #10917, 1000.000000000000114 ) ;
#59515=ORIENTED_EDGE ( 'NONE', *, *, #33620, .F. ) ;
#59516=CARTESIAN_POINT ( 'NONE',  ( 9.457462135716001583, -5.100000000000000533, -6.571291218949999902 ) ) ;
#59532=DIRECTION ( 'NONE',  ( 0.000000000000000000, 1.000000000000000000, 0.000000000000000000 ) ) ;
#59533=CARTESIAN_POINT ( 'NONE',  ( 10.31499432720999998, -5.458372854186999135, -8.355103994551999591 ) ) ;
#59538=CARTESIAN_POINT ( 'NONE',  ( 11.09999999999999964, -2.649999999999999911, 7.500000000000000000 ) ) ;
#59539=CARTESIAN_POINT ( 'NONE',  ( 8.567745513186627804, -3.352117027730234344, 5.929420235999764088 ) ) ;
#59550=CARTESIAN_POINT ( 'NONE',  ( 9.380781717619999682, -2.204246399534000034, 7.545378188773000261 ) ) ;
#59553=CARTESIAN_POINT ( 'NONE',  ( 10.90374822854000136, -3.726845778959999578, 5.900452123196999743 ) ) ;
#59565=CARTESIAN_POINT ( 'NONE',  ( 6.953052440528999512, -9.233022020364000326, -5.200634764108000851 ) ) ;
#59569=CARTESIAN_POINT ( 'NONE',  ( 7.621217240535393067, -3.646027591375869292, 8.814378988131492676 ) ) ;
#59582=VERTEX_POINT ( 'NONE', #53319 ) ;
#59589=CARTESIAN_POINT ( 'NONE',  ( 9.696086916451999826, -2.554404004330999900, 7.600685922079000179 ) ) ;
#59596=CARTESIAN_POINT ( 'NONE',  ( 10.50084194037999907, -4.616788958496999662, -6.288071994190999270 ) ) ;
#59607=CARTESIAN_POINT ( 'NONE',  ( 9.346662412757066107, -3.521875972694050283, 9.173020653676831060 ) ) ;
#59609=CARTESIAN_POINT ( 'NONE',  ( 8.228368194306998618, -4.806758213702000404, 6.177034600996000435 ) ) ;
#59615=CARTESIAN_POINT ( 'NONE',  ( 9.215289122285998502, -4.861979632688999686, 8.938813901364000003 ) ) ;
#59620=VERTEX_POINT ( 'NONE', #44222 ) ;
#59626=CARTESIAN_POINT ( 'NONE',  ( 9.660601868375998436, -2.901236202253999696, -6.151180522693000086 ) ) ;
#59628=CARTESIAN_POINT ( 'NONE',  ( 9.069724726289001282, -4.108965473266000146, 8.851626696081998702 ) ) ;
#59637=CARTESIAN_POINT ( 'NONE',  ( 11.10000000000000142, -5.360253205841783775, 6.560009693585453938 ) ) ;
#59640=CARTESIAN_POINT ( 'NONE',  ( 8.096558059622999792, -5.061720701958000390, 5.824087910811999613 ) ) ;
#59648=EDGE_CURVE ( 'NONE', #15625, #54866, #13526, .T. ) ;
#59660=CARTESIAN_POINT ( 'NONE',  ( 8.399899185017186909, -2.585175040501215715, 8.516097464460264277 ) ) ;
#59664=CARTESIAN_POINT ( 'NONE',  ( 11.09999999999999964, -2.700000000746000328, 5.148510364898998937 ) ) ;
#59672=SURFACE_SIDE_STYLE ('',( #21913 ) ) ;
#59694=VERTEX_POINT ( 'NONE', #3949 ) ;
#59698=CARTESIAN_POINT ( 'NONE',  ( 10.46009514222999925, -2.565650894080999667, -6.975682682930000489 ) ) ;
#59702=CARTESIAN_POINT ( 'NONE',  ( 5.699999999877000789, -1.433333330872999856, 10.65401593578999950 ) ) ;
#59703=EDGE_LOOP ( 'NONE', ( #21592, #40468, #27185, #48066 ) ) ;
#59710=CARTESIAN_POINT ( 'NONE',  ( 11.09999999999999964, -2.700000000000000178, -5.157071250680000496 ) ) ;
#59718=DIRECTION ( 'NONE',  ( -1.000000000000000000, 0.000000000000000000, 0.000000000000000000 ) ) ;
#59724=CARTESIAN_POINT ( 'NONE',  ( 10.66914689902483104, -4.353380376947088237, -8.814970433265349570 ) ) ;
#59728=CARTESIAN_POINT ( 'NONE',  ( 10.82894633243970084, -2.649868422364446197, -7.263390030261637875 ) ) ;
#59734=CARTESIAN_POINT ( 'NONE',  ( 9.736871746126999128, -2.742172332680000046, 6.839224809731999422 ) ) ;
#59738=EDGE_CURVE ( 'NONE', #518, #30733, #14390, .T. ) ;
#59741=CARTESIAN_POINT ( 'NONE',  ( 11.07691935321000010, -3.101896674955000321, -8.926549689995999515 ) ) ;
#59742=CARTESIAN_POINT ( 'NONE',  ( 7.654159297465730205, -5.473926550294729410, 6.558698546940537888 ) ) ;
#59743=CARTESIAN_POINT ( 'NONE',  ( 10.18755811987000115, -5.387486580809999204, 8.640943191857999750 ) ) ;
#59760=CARTESIAN_POINT ( 'NONE',  ( 8.817629440380001071, -3.894643656844000379, 6.044452984962999764 ) ) ;
#59763=FACE_OUTER_BOUND ( 'NONE', #65440, .T. ) ;
#59766=CARTESIAN_POINT ( 'NONE',  ( 10.60770805961999841, -2.392337812398999564, -6.587351599745000286 ) ) ;
#59769=CARTESIAN_POINT ( 'NONE',  ( 10.57893103570000015, -4.649956431060000561, 5.681096060554999383 ) ) ;
#59792=B_SPLINE_SURFACE_WITH_KNOTS ( 'NONE', 3, 3, ( 
 ( #12410, #60645, #12758, #34087 ),
 ( #28854, #2265, #44923, #20057 ),
 ( #35461, #8884, #47666, #68626 ),
 ( #25300, #14480, #52906, #41724 ),
 ( #63028, #46638, #41385, #9213 ) ),
 .UNSPECIFIED., .F., .F., .F.,
 ( 4, 1, 4 ),
 ( 4, 4 ),
 ( 0.5689291519175999623, 0.5833333333333000637, 0.5933409168203001016 ),
 ( -0.1884349902748000127, 1.188531000832999895 ),
 .UNSPECIFIED. ) ;
#59806=PLANE ( 'NONE',  #61948 ) ;
#59811=CARTESIAN_POINT ( 'NONE',  ( 5.500000000000000000, 0.4800000000000000377, -1.889999999999999902 ) ) ;
#59814=CARTESIAN_POINT ( 'NONE',  ( 11.09999999999999964, -3.512324525112999751, -8.971282648301999174 ) ) ;
#59823=CARTESIAN_POINT ( 'NONE',  ( 11.09999999999999964, -2.899999999999999911, 4.467422426380999845 ) ) ;
#59824=CARTESIAN_POINT ( 'NONE',  ( 7.100000000000000533, 0.000000000000000000, 0.000000000000000000 ) ) ;
#59831=CARTESIAN_POINT ( 'NONE',  ( 11.24323064679000161, -2.479730344050999680, -7.587230764681999418 ) ) ;
#59835=ADVANCED_FACE ( 'NONE', ( #20385 ), #32920, .F. ) ;
#59851=CARTESIAN_POINT ( 'NONE',  ( 10.31499432720999998, -5.458372854186999135, -8.355103994551999591 ) ) ;
#59853=ORIENTED_EDGE ( 'NONE', *, *, #45924, .F. ) ;
#59861=CARTESIAN_POINT ( 'NONE',  ( 10.28117360717000039, -4.719545580892999581, 4.850090003780999304 ) ) ;
#59865=CARTESIAN_POINT ( 'NONE',  ( 10.23808992278000041, -2.752437370156000540, 6.820045513931999537 ) ) ;
#59876=CARTESIAN_POINT ( 'NONE',  ( 10.79839246847000034, -5.269358106415999110, -6.148714306659999629 ) ) ;
#59879=CARTESIAN_POINT ( 'NONE',  ( 10.52314899745999988, -5.167567567567999731, -6.822293592207000934 ) ) ;
#59881=CARTESIAN_POINT ( 'NONE',  ( 8.625788328778114078, -2.987667598876605712, -6.606157699978479236 ) ) ;
#59883=CARTESIAN_POINT ( 'NONE',  ( 10.99999999997000089, -4.000000000000000000, -8.949999999965999820 ) ) ;
#59894=CARTESIAN_POINT ( 'NONE',  ( 11.14698053895999941, -5.129799765052999838, 5.886044098803999702 ) ) ;
#59897=CARTESIAN_POINT ( 'NONE',  ( 10.65550933554000146, -4.237674644795000667, 9.105223721671999115 ) ) ;
#59898=CARTESIAN_POINT ( 'NONE',  ( 9.645238140867222754, -5.359248881483462235, 6.398502314407720881 ) ) ;
#59906=CARTESIAN_POINT ( 'NONE',  ( 10.95046608577698066, -2.858708611104648245, -5.102140212562284560 ) ) ;
#59914=CARTESIAN_POINT ( 'NONE',  ( 7.704343083128708969, -2.684466035400899120, 7.853284348082095079 ) ) ;
#59921=ORIENTED_EDGE ( 'NONE', *, *, #25663, .T. ) ;
#59935=CARTESIAN_POINT ( 'NONE',  ( 10.56492304196000021, -4.212244324161999565, 8.933470634735002136 ) ) ;
#59941=CARTESIAN_POINT ( 'NONE',  ( 11.10664194037999941, -5.324199331986000594, -7.809344861333999965 ) ) ;
#59952=CARTESIAN_POINT ( 'NONE',  ( 8.222954734881996686, -4.680061443183004322, 6.135926641887999189 ) ) ;
#59961=CARTESIAN_POINT ( 'NONE',  ( 7.716851002542999716, -2.832432432432000269, 6.822293592207000934 ) ) ;
#59962=EDGE_CURVE ( 'NONE', #53841, #62127, #40700, .T. ) ;
#59965=ORIENTED_EDGE ( 'NONE', *, *, #27709, .T. ) ;
#59970=CARTESIAN_POINT ( 'NONE',  ( 7.298591271593769747, -3.170842933427397536, 6.420501794657867300 ) ) ;
#59972=CARTESIAN_POINT ( 'NONE',  ( 8.989144353209001181, -5.284133759825000887, 6.489273023403000273 ) ) ;
#59975=CARTESIAN_POINT ( 'NONE',  ( 10.96239488738000034, -6.767643977940999811, 5.462428178478999641 ) ) ;
#59976=CARTESIAN_POINT ( 'NONE',  ( 9.203545614489009097, -5.098876553266001643, -6.624379381313996618 ) ) ;
#59977=FACE_OUTER_BOUND ( 'NONE', #67264, .T. ) ;
#59983=CARTESIAN_POINT ( 'NONE',  ( 8.417495559623999313, -2.029110377978999846, 7.726994002375999315 ) ) ;
#59984=DIRECTION ( 'NONE',  ( -0.7071067811864923947, -0.6115518252005933686, -0.3549709355621961659 ) ) ;
#59999=CARTESIAN_POINT ( 'NONE',  ( 11.09999999999999964, -2.700000000000000178, -6.461133846875999787 ) ) ;
#60004=CARTESIAN_POINT ( 'NONE',  ( 8.590676109800844173, -4.354029080878516034, 5.795624387936125110 ) ) ;
#60016=ORIENTED_EDGE ( 'NONE', *, *, #46287, .T. ) ;
#60021=CARTESIAN_POINT ( 'NONE',  ( 8.745593092018999926, -5.100000000000000533, 6.404090157675000228 ) ) ;
#60028=B_SPLINE_CURVE_WITH_KNOTS ( 'NONE', 3,
 ( #41077, #46327, #68314, #62729 ),
 .UNSPECIFIED., .F., .F.,
 ( 4, 4 ),
 ( 0.000000000000000000, 0.1070776897655759813 ),
 .UNSPECIFIED. ) ;
#60034=CARTESIAN_POINT ( 'NONE',  ( 6.825988380485000562, -9.284830207118000445, 5.366267983674999797 ) ) ;
#60037=VECTOR ( 'NONE', #32096, 1000.000000000000000 ) ;
#60047=CARTESIAN_POINT ( 'NONE',  ( 10.09454055528000005, -5.362855569781999954, -7.550030734599999960 ) ) ;
#60051=EDGE_CURVE ( 'NONE', #438, #50410, #49023, .T. ) ;
#60073=CARTESIAN_POINT ( 'NONE',  ( 8.566230646795000681, -5.212258818969000451, 6.157189191035000064 ) ) ;
#60074=CARTESIAN_POINT ( 'NONE',  ( 9.705151033051999221, -4.316974633926000671, -5.653758079558000027 ) ) ;
#60079=CARTESIAN_POINT ( 'NONE',  ( 10.56498513754060653, -5.349957030113857925, -7.500000808964294663 ) ) ;
#60088=CARTESIAN_POINT ( 'NONE',  ( 9.687876499438001332, -5.912252057206999645, 7.772299417761000306 ) ) ;
#60093=CARTESIAN_POINT ( 'NONE',  ( 11.15264435320999858, -2.317067032475999877, -7.596564138533999255 ) ) ;
#60094=CARTESIAN_POINT ( 'NONE',  ( 7.685231687083611263, -5.714952426232358107, 7.177445099263493056 ) ) ;
#60095=CARTESIAN_POINT ( 'NONE',  ( 9.256662271119999730, -4.025830307267999508, 9.295859242339000517 ) ) ;
#60102=EDGE_CURVE ( 'NONE', #37807, #14642, #63518, .T. ) ;
#60113=ORIENTED_EDGE ( 'NONE', *, *, #73, .F. ) ;
#60123=CARTESIAN_POINT ( 'NONE',  ( 7.996487690580287300, -5.313957503663140791, 7.853744048643361175 ) ) ;
#60131=CARTESIAN_POINT ( 'NONE',  ( 11.09999999999999964, -2.649999999999999911, 7.500000000000000000 ) ) ;
#60140=CARTESIAN_POINT ( 'NONE',  ( 10.90000000000000036, -1.433333333332999837, -10.65401593558000037 ) ) ;
#60141=EDGE_CURVE ( 'NONE', #51331, #21554, #20219, .T. ) ;
#60158=ADVANCED_FACE ( 'NONE', ( #9372 ), #37357, .F. ) ;
#60165=ORIENTED_EDGE ( 'NONE', *, *, #43505, .F. ) ;
#60187=CARTESIAN_POINT ( 'NONE',  ( 10.77401935321000082, -3.826867196099999813, -5.823197386290999589 ) ) ;
#60207=CARTESIAN_POINT ( 'NONE',  ( 9.882901294779998125, -4.314558311729999929, -9.161035779983999205 ) ) ;
#60209=CARTESIAN_POINT ( 'NONE',  ( 10.53324933263040819, -3.041617253709827384, -5.009215415433663665 ) ) ;
#60213=EDGE_LOOP ( 'NONE', ( #28548, #8935, #42463, #38777, #28929, #30953 ) ) ;
#60215=CARTESIAN_POINT ( 'NONE',  ( 11.14212519252000000, -5.326817661814000182, 4.985844344934000638 ) ) ;
#60219=CARTESIAN_POINT ( 'NONE',  ( 10.31457635473999979, -5.362146312020000138, 6.677778992223999843 ) ) ;
#60233=CARTESIAN_POINT ( 'NONE',  ( 10.74708735964999917, -5.603138702306000418, -6.963343193308999979 ) ) ;
#60237=CARTESIAN_POINT ( 'NONE',  ( 9.172139116365000788, -4.730747404809998891, -8.668230005597001409 ) ) ;
#60249=CARTESIAN_POINT ( 'NONE',  ( 11.25041341105000114, -5.730771985297000271, 8.122672103119001008 ) ) ;
#60252=CARTESIAN_POINT ( 'NONE',  ( 10.03491210303999992, -5.615910465798999773, 7.351455544018000943 ) ) ;
#60253=CARTESIAN_POINT ( 'NONE',  ( 10.90076026837999912, -2.899999999941999640, -5.152573395210000129 ) ) ;
#60254=UNCERTAINTY_MEASURE_WITH_UNIT (LENGTH_MEASURE( 1.000000000000000082E-05 ), #45434, 'distance_accuracy_value', 'NONE');
#60279=FACE_OUTER_BOUND ( 'NONE', #7470, .T. ) ;
#60280=CARTESIAN_POINT ( 'NONE',  ( 8.160745559622998968, -5.944572422272999646, 7.106845737860000511 ) ) ;
#60284=B_SPLINE_CURVE_WITH_KNOTS ( 'NONE', 3,
 ( #37834, #88, #47648, #37489 ),
 .UNSPECIFIED., .F., .F.,
 ( 4, 4 ),
 ( 0.000000000000000000, 1.000000000000000000 ),
 .UNSPECIFIED. ) ;
#60285=CARTESIAN_POINT ( 'NONE',  ( 7.936333720142999759, -5.123034382927999175, 6.721303993095999907 ) ) ;
#60288=CARTESIAN_POINT ( 'NONE',  ( 10.13050497920000126, -3.092053006542000215, 8.629388195475000245 ) ) ;
#60293=CARTESIAN_POINT ( 'NONE',  ( 10.87946694038000039, -2.817416132545000007, -6.828662897514999663 ) ) ;
#60297=CARTESIAN_POINT ( 'NONE',  ( 9.674373738639999942, -2.899999999999999911, -6.185493860157000867 ) ) ;
#60307=B_SPLINE_CURVE_WITH_KNOTS ( 'NONE', 3,
 ( #4068, #47779, #69086, #15947 ),
 .UNSPECIFIED., .F., .F.,
 ( 4, 4 ),
 ( 0.000000000000000000, 1.000000000000000000 ),
 .UNSPECIFIED. ) ;
#60311=CARTESIAN_POINT ( 'NONE',  ( 10.83668192271000130, -4.288535286065000562, 9.448729895547000268 ) ) ;
#60314=ORIENTED_EDGE ( 'NONE', *, *, #21303, .T. ) ;
#60319=CARTESIAN_POINT ( 'NONE',  ( 10.44080359545000114, -5.435731278187999393, 7.303630150377999009 ) ) ;
#60320=CARTESIAN_POINT ( 'NONE',  ( 9.157210916635261100, -5.507291520428013953, 6.616308516811844953 ) ) ;
#60321=CARTESIAN_POINT ( 'NONE',  ( 7.486433059621999675, -5.321924421352999701, 8.118250081378000971 ) ) ;
#60325=CARTESIAN_POINT ( 'NONE',  ( 11.01655322883999943, -6.705649024436000083, 5.522682893586000397 ) ) ;
#60329=B_SPLINE_CURVE_WITH_KNOTS ( 'NONE', 3,
 ( #24791, #40193, #50333, #61509, #29716, #8374 ),
 .UNSPECIFIED., .F., .F.,
 ( 4, 2, 4 ),
 ( 0.000000000000000000, 0.4999999999999994449, 1.000000000000000000 ),
 .UNSPECIFIED. ) ;
#60339=CARTESIAN_POINT ( 'NONE',  ( 10.31498017945871126, -2.650031506806249659, -7.499998780888571304 ) ) ;
#60340=CARTESIAN_POINT ( 'NONE',  ( 7.895317210312003731, -5.140737874544996977, 6.778394131643998399 ) ) ;
#60343=VERTEX_POINT ( 'NONE', #18003 ) ;
#60355=DIRECTION ( 'NONE',  ( 0.9999999999999326095, -3.671478400246118675E-07, 1.807828440105059414E-09 ) ) ;
#60356=CARTESIAN_POINT ( 'NONE',  ( 9.625489929093001606, -3.134630999349000025, 8.626959345509000343 ) ) ;
#60357=ORIENTED_EDGE ( 'NONE', *, *, #50916, .F. ) ;
#60358=CARTESIAN_POINT ( 'NONE',  ( 9.525000000000000355, -4.417172942406000224, 8.783926296998000538 ) ) ;
#60365=CARTESIAN_POINT ( 'NONE',  ( 10.56742170454999830, -8.204434595504999095, 6.610786703431000610 ) ) ;
#60368=LINE ( 'NONE', #28211, #21954 ) ;
#60383=CARTESIAN_POINT ( 'NONE',  ( 9.041074696474980854, -2.899999999999999911, 6.201633003103719233 ) ) ;
#60384=CARTESIAN_POINT ( 'NONE',  ( 5.500000000000000000, -1.406666666667000021, 10.45580168561000001 ) ) ;
#60395=CARTESIAN_POINT ( 'NONE',  ( 11.10061802256000085, -3.093055606601000207, -6.153681532251999542 ) ) ;
#60405=CARTESIAN_POINT ( 'NONE',  ( 8.924662153698962541, -5.350575487761723537, 7.500021879703682615 ) ) ;
#60413=AXIS2_PLACEMENT_3D ( 'NONE', #26797, #63139, #15264 ) ;
#60416=CARTESIAN_POINT ( 'NONE',  ( 9.298691940377999288, -5.159251056493999954, 9.109488373271000583 ) ) ;
#60417=CARTESIAN_POINT ( 'NONE',  ( 9.617147628285000138, -2.491831134779999957, -6.388915175267000812 ) ) ;
#60431=CARTESIAN_POINT ( 'NONE',  ( 9.722771884505998941, -5.493781611190000191, 6.566828939965000167 ) ) ;
#60436=CARTESIAN_POINT ( 'NONE',  ( 11.18236694037999968, -4.516641106826999597, -8.757887038823000125 ) ) ;
#60437=CARTESIAN_POINT ( 'NONE',  ( 8.093329789650123729, -4.416228695728097620, 5.811362191399359389 ) ) ;
#60438=CARTESIAN_POINT ( 'NONE',  ( 10.49785673611999925, -3.776281940467000275, 5.717636230565000588 ) ) ;
#60446=ORIENTED_EDGE ( 'NONE', *, *, #47519, .F. ) ;
#60455=B_SPLINE_CURVE_WITH_KNOTS ( 'NONE', 3,
 ( #40244, #29772, #28729, #12637 ),
 .UNSPECIFIED., .F., .F.,
 ( 4, 4 ),
 ( 0.000000000000000000, 1.000000000000000000 ),
 .UNSPECIFIED. ) ;
#60463=CARTESIAN_POINT ( 'NONE',  ( 10.98633305961999973, -3.015090804604000141, -9.064432363387998848 ) ) ;
#60466=CARTESIAN_POINT ( 'NONE',  ( 10.46754921866999943, -2.318350880468999620, 6.549783596838000044 ) ) ;
#60499=CARTESIAN_POINT ( 'NONE',  ( 9.331129440379999807, -4.141908960411000429, 6.047561724438000219 ) ) ;
#60507=CARTESIAN_POINT ( 'NONE',  ( 9.665180073187563892, -2.900412407185302577, -6.162603501924860616 ) ) ;
#60518=CARTESIAN_POINT ( 'NONE',  ( 7.424327003564875405, -2.348384993112772712, 8.046123069814775874 ) ) ;
#60527=VECTOR ( 'NONE', #15594, 1000.000000000000114 ) ;
#60550=CARTESIAN_POINT ( 'NONE',  ( 11.08752429429999964, -2.871531501602999636, -6.302910744985999791 ) ) ;
#60557=CONICAL_SURFACE ( 'NONE', #33766, 1.349999998858999906, 0.7853981633972997312 ) ;
#60559=CARTESIAN_POINT ( 'NONE',  ( 10.32936131915000111, -4.919631126329000459, 4.567352568837999449 ) ) ;
#60563=CARTESIAN_POINT ( 'NONE',  ( 9.351499161061999743, -4.821938821912000073, 8.950150764319998231 ) ) ;
#60571=CARTESIAN_POINT ( 'NONE',  ( 11.04677151279999947, -2.764386413791999786, -5.039776830043000366 ) ) ;
#60572=VECTOR ( 'NONE', #8018, 1000.000000000000114 ) ;
#60575=FACE_OUTER_BOUND ( 'NONE', #64267, .T. ) ;
#60576=CARTESIAN_POINT ( 'NONE',  ( 10.99479839230999900, -3.850614833844999918, -9.347951988117998212 ) ) ;
#60581=CARTESIAN_POINT ( 'NONE',  ( 9.260142521132999960, -3.283392111224999965, -8.676955243274001361 ) ) ;
#60587=CARTESIAN_POINT ( 'NONE',  ( 10.26948634882999833, -3.369491526607000242, 4.845903792981999914 ) ) ;
#60588=CARTESIAN_POINT ( 'NONE',  ( 9.268025422169147376, -5.100000000000000533, 6.452077467066149374 ) ) ;
#60591=CARTESIAN_POINT ( 'NONE',  ( 9.075489683949001574, -4.020837068201999820, 8.948702918089999514 ) ) ;
#60594=CARTESIAN_POINT ( 'NONE',  ( 10.93227479887999998, -2.539880901735999785, 6.453614191797999666 ) ) ;
#60595=CARTESIAN_POINT ( 'NONE',  ( 9.979272590049129477, -2.371809606018679517, 6.860647176154606619 ) ) ;
#60607=CARTESIAN_POINT ( 'NONE',  ( 9.658740731405000446, -5.476443305113000370, -7.051545409824000465 ) ) ;
#60609=ORIENTED_EDGE ( 'NONE', *, *, #26995, .T. ) ;
#60624=CARTESIAN_POINT ( 'NONE',  ( 8.610058059625000482, -5.329429281359999493, 6.027400270608000099 ) ) ;
#60631=CARTESIAN_POINT ( 'NONE',  ( 9.199609130449999839, -2.551382302226000487, 7.536606162076999738 ) ) ;
#60638=ORIENTED_EDGE ( 'NONE', *, *, #37135, .F. ) ;
#60641=CARTESIAN_POINT ( 'NONE',  ( 10.90437356726000040, -2.900476673752999890, 5.132566153004000320 ) ) ;
#60645=CARTESIAN_POINT ( 'NONE',  ( 6.829431761257999334, -9.270817568204998693, -5.218560984457999652 ) ) ;
#60653=CARTESIAN_POINT ( 'NONE',  ( 9.843726350706999639, -4.115123626494000320, 9.466607949400000166 ) ) ;
#60663=CARTESIAN_POINT ( 'NONE',  ( 8.705995559625000269, -2.542850487891999745, 7.419808283050000064 ) ) ;
#60664=DIRECTION ( 'NONE',  ( -1.000000000000000000, -5.940303223299999030E-14, -1.603881870291000016E-12 ) ) ;
#60681=CARTESIAN_POINT ( 'NONE',  ( 8.295839940244002619, -5.118638632597003912, 6.383292232312004266 ) ) ;
#60692=ADVANCED_FACE ( 'NONE', ( #27719 ), #21762, .T. ) ;
#60701=VERTEX_POINT ( 'NONE', #68623 ) ;
#60702=CARTESIAN_POINT ( 'NONE',  ( 9.492234138830133006, -4.893440334305921624, 8.512184316248376348 ) ) ;
#60711=VERTEX_POINT ( 'NONE', #11274 ) ;
#60719=CARTESIAN_POINT ( 'NONE',  ( 10.71654240785884582, -2.829812247203900899, 6.826803421738888211 ) ) ;
#60725=CARTESIAN_POINT ( 'NONE',  ( 11.09999999999999964, -1.300000000000000044, -10.46294468575422876 ) ) ;
#60735=CARTESIAN_POINT ( 'NONE',  ( 9.819572261909000233, -2.688237737290000151, -7.873041261681999359 ) ) ;
#60743=CARTESIAN_POINT ( 'NONE',  ( 10.85460595134973794, -2.649926015912494215, -7.676664732030310745 ) ) ;
#60756=CARTESIAN_POINT ( 'NONE',  ( 7.501441940376999185, -2.138201851198999748, 6.814774777484000623 ) ) ;
#60761=AXIS2_PLACEMENT_3D ( 'NONE', #34647, #44789, #12619 ) ;
#60768=ORIENTED_EDGE ( 'NONE', *, *, #65506, .T. ) ;
#60772=CARTESIAN_POINT ( 'NONE',  ( 10.22399006116000031, -5.507891002176999784, 6.589804341508000540 ) ) ;
#60773=CARTESIAN_POINT ( 'NONE',  ( 8.577620559625000141, -3.981661727120999750, 8.959239802162999311 ) ) ;
#60778=CARTESIAN_POINT ( 'NONE',  ( 10.31152944037999930, -2.716820959546999870, -7.950167805575999225 ) ) ;
#60779=CARTESIAN_POINT ( 'NONE',  ( 7.898990479458490199, -2.593905526383240012, 8.523572096125727526 ) ) ;
#60780=CARTESIAN_POINT ( 'NONE',  ( 10.09697182628999990, -5.253379538902000156, 8.530665717066000298 ) ) ;
#60791=CARTESIAN_POINT ( 'NONE',  ( 10.01574583856000089, -4.333399685216000385, -9.088699530815999239 ) ) ;
#60800=CIRCLE ( 'NONE', #30655, 0.8000000000000002665 ) ;
#60802=CARTESIAN_POINT ( 'NONE',  ( 8.919605646795000453, -5.165500668528999917, 8.645534272955000432 ) ) ;
#60807=ADVANCED_FACE ( 'NONE', ( #44837 ), #54623, .F. ) ;
#60809=CARTESIAN_POINT ( 'NONE',  ( 10.38053305961999939, -5.283785200568999585, -8.830188095997000275 ) ) ;
#60821=B_SPLINE_CURVE_WITH_KNOTS ( 'NONE', 3,
 ( #28949, #43980, #66321, #17045 ),
 .UNSPECIFIED., .F., .F.,
 ( 4, 4 ),
 ( 0.000000000000000000, 1.000000000000000000 ),
 .UNSPECIFIED. ) ;
#60842=CARTESIAN_POINT ( 'NONE',  ( 8.766851002546001581, -2.832432432432000269, 6.822293592207000934 ) ) ;
#60846=CARTESIAN_POINT ( 'NONE',  ( 10.78447049185723650, -4.843240479914882712, 9.027236721787854634 ) ) ;
#60847=CARTESIAN_POINT ( 'NONE',  ( 8.304129440378000382, -3.650411072918999800, 6.083135626079000602 ) ) ;
#60848=DIRECTION ( 'NONE',  ( 0.000000000000000000, -0.7071067811865475727, 0.7071067811865475727 ) ) ;
#60863=CARTESIAN_POINT ( 'NONE',  ( 9.216851002545999094, -2.832432432432000269, 6.822293592207000934 ) ) ;
#60866=CARTESIAN_POINT ( 'NONE',  ( 7.424973819922880303, -2.343829071653882323, 8.032060285052104120 ) ) ;
#60869=ORIENTED_EDGE ( 'NONE', *, *, #16170, .F. ) ;
#60872=CARTESIAN_POINT ( 'NONE',  ( 10.87955921103774237, -5.549441030678586628, -8.346382036815052530 ) ) ;
#60874=AXIS2_PLACEMENT_3D ( 'NONE', #13021, #7766, #44151 ) ;
#60877=CARTESIAN_POINT ( 'NONE',  ( 10.61442944038000036, -5.287639274524000399, -7.937245019889999753 ) ) ;
#60878=CARTESIAN_POINT ( 'NONE',  ( 10.98953890776378906, -5.566676525139746978, 4.946116539698106607 ) ) ;
#60893=CARTESIAN_POINT ( 'NONE',  ( 10.98768472625999948, -6.720753154780999772, 5.471698433974999887 ) ) ;
#60896=CARTESIAN_POINT ( 'NONE',  ( 10.42081395746000005, -2.488448635474999726, -7.717895569088000229 ) ) ;
#60897=CARTESIAN_POINT ( 'NONE',  ( 10.16000000000000014, -4.496968146123999865, -8.755198255949000696 ) ) ;
#60903=CARTESIAN_POINT ( 'NONE',  ( 11.09999999999999964, -4.000000000000000000, -7.500000000000000000 ) ) ;
#60907=CARTESIAN_POINT ( 'NONE',  ( 10.92717634842000152, -5.023656093247000243, 8.718039182945998888 ) ) ;
#60913=CARTESIAN_POINT ( 'NONE',  ( 11.10000000009000054, -5.300000000088999741, -6.571291220400000022 ) ) ;
#60917=VECTOR ( 'NONE', #28023, 1000.000000000000000 ) ;
#60922=DIRECTION ( 'NONE',  ( 1.000000000000000000, 0.000000000000000000, 0.000000000000000000 ) ) ;
#60925=CARTESIAN_POINT ( 'NONE',  ( 9.570737326637999587, -4.261100936929000049, -5.979198511086000423 ) ) ;
#60938=CARTESIAN_POINT ( 'NONE',  ( 10.87021507563000000, -2.226042145532000305, 7.782753277595999997 ) ) ;
#60941=CARTESIAN_POINT ( 'NONE',  ( 9.538434317036999843, -5.620900626097999897, 7.423100105894999245 ) ) ;
#60949=CARTESIAN_POINT ( 'NONE',  ( 8.432767466320006733, -2.913363525153000566, -6.617750919463998294 ) ) ;
#60954=CARTESIAN_POINT ( 'NONE',  ( 9.172139116365000788, -4.730747404809998891, -8.668230005597001409 ) ) ;
#60978=ORIENTED_EDGE ( 'NONE', *, *, #30017, .T. ) ;
#60979=CARTESIAN_POINT ( 'NONE',  ( 9.634027193201999850, -3.042970193091000031, 8.588108172435999776 ) ) ;
#60991=CARTESIAN_POINT ( 'NONE',  ( 9.353051448577010873, -3.388693121031217448, 9.128448243495800085 ) ) ;
#60993=CARTESIAN_POINT ( 'NONE',  ( 8.320275543017386255, -5.099114840939221516, 6.576957048925175187 ) ) ;
#60998=CARTESIAN_POINT ( 'NONE',  ( 9.815199780373001559, -2.813634733202999616, 8.848854270764999086 ) ) ;
#61000=AXIS2_PLACEMENT_3D ( 'NONE', #42561, #20544, #62495 ) ;
#61002=EDGE_CURVE ( 'NONE', #22542, #46692, #56383, .T. ) ;
#61012=CARTESIAN_POINT ( 'NONE',  ( 7.165495559622000243, -2.688354259407999880, 8.140021027181001401 ) ) ;
#61026=CARTESIAN_POINT ( 'NONE',  ( 11.09999999999999964, -5.299999999999999822, -5.157071272631999825 ) ) ;
#61040=ORIENTED_EDGE ( 'NONE', *, *, #58437, .T. ) ;
#61047=VERTEX_POINT ( 'NONE', #35148 ) ;
#61049=CYLINDRICAL_SURFACE ( 'NONE', #35076, 1.350000000000000089 ) ;
#61050=VERTEX_POINT ( 'NONE', #61362 ) ;
#61052=CARTESIAN_POINT ( 'NONE',  ( 7.956793146791999227, -4.524489047957000132, 9.047757046927999980 ) ) ;
#61055=ORIENTED_EDGE ( 'NONE', *, *, #67967, .T. ) ;
#61056=CARTESIAN_POINT ( 'NONE',  ( 6.790909542087999462, -9.291477070232998514, 5.323632131722000338 ) ) ;
#61067=CARTESIAN_POINT ( 'NONE',  ( 9.739312519577287830, -2.650230560758064069, 7.263871480528514724 ) ) ;
#61070=CARTESIAN_POINT ( 'NONE',  ( 10.95460932063975790, -2.828099631735832453, -6.694244964707101175 ) ) ;
#61084=CARTESIAN_POINT ( 'NONE',  ( 9.937415816209998809, -3.510658118802999716, -6.227041669085999764 ) ) ;
#61086=CARTESIAN_POINT ( 'NONE',  ( 9.041114232695017350, -4.912826217066823986, 8.494526172176604106 ) ) ;
#61088=EDGE_CURVE ( 'NONE', #25113, #31044, #19395, .T. ) ;
#61092=DIRECTION ( 'NONE',  ( 0.000000000000000000, 0.000000000000000000, -1.000000000000000000 ) ) ;
#61094=CARTESIAN_POINT ( 'NONE',  ( 11.09999999999999964, -4.000000000000000000, 7.500000000000000000 ) ) ;
#61106=CARTESIAN_POINT ( 'NONE',  ( 8.116918146793999256, -5.773185758034999893, 7.141496747382000798 ) ) ;
#61108=ADVANCED_FACE ( 'NONE', ( #28880 ), #26536, .F. ) ;
#61124=CARTESIAN_POINT ( 'NONE',  ( 9.667080975990000269, -4.541622198376999542, 5.824041840233000755 ) ) ;
#61128=CARTESIAN_POINT ( 'NONE',  ( 10.46297944037999983, -3.993164663709000362, -6.140164943008000087 ) ) ;
#61129=CARTESIAN_POINT ( 'NONE',  ( 7.975403604543350511, -2.344124067439634640, 6.939139580511310079 ) ) ;
#61130=CARTESIAN_POINT ( 'NONE',  ( 9.972852379787999766, -5.044471434015000533, 6.258101649750000384 ) ) ;
#61139=CARTESIAN_POINT ( 'NONE',  ( 11.09999999999999964, -5.299999999999999822, -5.157071272631999825 ) ) ;
#61150=CARTESIAN_POINT ( 'NONE',  ( 7.700043146791999860, -3.346260729029000291, 6.002247316312999459 ) ) ;
#61156=CARTESIAN_POINT ( 'NONE',  ( 9.926183059621999760, -4.356410583133000003, -9.313949118577001585 ) ) ;
#61176=EDGE_CURVE ( 'NONE', #31977, #50708, #59308, .T. ) ;
#61192=CARTESIAN_POINT ( 'NONE',  ( 10.73166211313188256, -5.609524154758663173, 8.188827626220106737 ) ) ;
#61193=CARTESIAN_POINT ( 'NONE',  ( 8.085168146793000332, -2.431397064767999439, 7.958394431095000776 ) ) ;
#61200=ADVANCED_FACE ( 'NONE', ( #9582 ), #18267, .F. ) ;
#61214=CARTESIAN_POINT ( 'NONE',  ( 7.417028609100216663, -2.407073382786591775, 8.200060021492962647 ) ) ;
#61216=CARTESIAN_POINT ( 'NONE',  ( 10.51720455738115412, -5.205742106671480407, 8.206130011351941533 ) ) ;
#61224=CARTESIAN_POINT ( 'NONE',  ( 9.624831031536459136, -2.894183647071444376, 8.301356454185306433 ) ) ;
#61225=CARTESIAN_POINT ( 'NONE',  ( 10.95519194037999888, -3.860335380237000180, -6.147338954930000376 ) ) ;
#61233=ORIENTED_EDGE ( 'NONE', *, *, #46002, .T. ) ;
#61239=ADVANCED_FACE ( 'NONE', ( #49754 ), #21508, .T. ) ;
#61242=CARTESIAN_POINT ( 'NONE',  ( 10.25888544622000076, -4.512389816463000081, 5.993697694029000544 ) ) ;
#61244=CARTESIAN_POINT ( 'NONE',  ( 10.28773706650000008, -5.077599250153999932, -5.991350640809000261 ) ) ;
#61254=CARTESIAN_POINT ( 'NONE',  ( 9.945535518573000999, -2.906050966242999856, 8.880386511481999534 ) ) ;
#61255=ORIENTED_EDGE ( 'NONE', *, *, #22958, .F. ) ;
#61270=DIRECTION ( 'NONE',  ( 2.709094309399999753E-09, -3.458058237665000178E-11, 1.000000000000000000 ) ) ;
#61282=ADVANCED_FACE ( 'NONE', ( #9162 ), #30499, .F. ) ;
#61283=CARTESIAN_POINT ( 'NONE',  ( 9.785087710366283886, -4.544774531727020062, -8.875930998700511054 ) ) ;
#61284=CARTESIAN_POINT ( 'NONE',  ( 10.24961784311999935, -4.184221496660999406, 9.286877953065999947 ) ) ;
#61288=CARTESIAN_POINT ( 'NONE',  ( 10.56492304196000021, -4.212244324161999565, 8.933470634735002136 ) ) ;
#61299=CARTESIAN_POINT ( 'NONE',  ( 9.480151033051999576, -4.233164088428999605, -6.141918726850000176 ) ) ;
#61302=CARTESIAN_POINT ( 'NONE',  ( 9.883148997457000817, -5.167567567567999731, 6.822293592207000934 ) ) ;
#61309=CARTESIAN_POINT ( 'NONE',  ( 9.365000000002998704, -2.649999999999999911, -7.500000000000000000 ) ) ;
#61311=ORIENTED_EDGE ( 'NONE', *, *, #43087, .F. ) ;
#61312=CYLINDRICAL_SURFACE ( 'NONE', #46250, 1.350000000000000089 ) ;
#61337=CARTESIAN_POINT ( 'NONE',  ( 9.382636167377327752, -2.846367580966820299, 8.802155020956973885 ) ) ;
#61341=CARTESIAN_POINT ( 'NONE',  ( 10.96543126312000105, -5.152333517825000264, -5.068250443055999810 ) ) ;
#61344=CARTESIAN_POINT ( 'NONE',  ( 10.00137895011999944, -3.855365288061999962, 5.709482985498999241 ) ) ;
#61353=CARTESIAN_POINT ( 'NONE',  ( 9.285047233936884581, -4.827112843486829341, 9.039507299413969577 ) ) ;
#61357=CARTESIAN_POINT ( 'NONE',  ( 11.07071157029000119, -6.643654070931000355, 5.582937608692000175 ) ) ;
#61358=CARTESIAN_POINT ( 'NONE',  ( 8.489692067425998800, -4.486659167649003521, -6.565674902303003435 ) ) ;
#61360=CARTESIAN_POINT ( 'NONE',  ( 10.26195635248000038, -3.348682106447000262, 4.591198220724000301 ) ) ;
#61362=CARTESIAN_POINT ( 'NONE',  ( 7.000000000000000000, -6.255435840762999966, 3.000000000000000000 ) ) ;
#61378=ORIENTED_EDGE ( 'NONE', *, *, #50916, .T. ) ;
#61391=CARTESIAN_POINT ( 'NONE',  ( 9.869049086607999399, -5.575175898444999945, 7.724300702620999104 ) ) ;
#61393=CARTESIAN_POINT ( 'NONE',  ( 9.842711596872401714, -5.100000000000000533, -6.305985889525932642 ) ) ;
#61394=CARTESIAN_POINT ( 'NONE',  ( 8.689254440380000943, -2.550228841911000188, 7.666975032000999946 ) ) ;
#61413=VERTEX_POINT ( 'NONE', #22054 ) ;
#61421=ORIENTED_EDGE ( 'NONE', *, *, #38258, .T. ) ;
#61429=CARTESIAN_POINT ( 'NONE',  ( 10.27571314244999989, -5.689440078020999714, -7.562019725378000601 ) ) ;
#61436=CARTESIAN_POINT ( 'NONE',  ( 7.822379440378000481, -4.636725880537000855, 9.378965771357000492 ) ) ;
#61449=CARTESIAN_POINT ( 'NONE',  ( 8.758793146794999984, -3.977267280662000193, 9.308921106447000327 ) ) ;
#61458=CARTESIAN_POINT ( 'NONE',  ( 9.508545572907237897, -8.547664595580219071, -6.555873143209844933 ) ) ;
#61461=CARTESIAN_POINT ( 'NONE',  ( 9.457462135716001583, -5.100000000000000533, -6.571291218949999902 ) ) ;
#61463=CARTESIAN_POINT ( 'NONE',  ( 10.13340376756999994, -5.653635692335999607, 6.501829690795999817 ) ) ;
#61465=ORIENTED_EDGE ( 'NONE', *, *, #16084, .T. ) ;
#61467=CARTESIAN_POINT ( 'NONE',  ( 10.16007944038000055, -4.812966563646999596, -8.526591612524001107 ) ) ;
#61470=CARTESIAN_POINT ( 'NONE',  ( 7.906377990995630434, -2.507223990358470989, 8.393237994738566243 ) ) ;
#61471=CARTESIAN_POINT ( 'NONE',  ( 10.53138988903999973, -5.607755226963999640, 7.280101849877000042 ) ) ;
#61475=CARTESIAN_POINT ( 'NONE',  ( 9.074999999999999289, -4.417172942406000224, 8.783926296998000538 ) ) ;
#61480=CARTESIAN_POINT ( 'NONE',  ( 9.927742433789001453, -5.651611919872999934, -7.935921913274999184 ) ) ;
#61491=CARTESIAN_POINT ( 'NONE',  ( 8.122956853208000538, -3.566638198986999964, 5.743608852252999775 ) ) ;
#61496=CARTESIAN_POINT ( 'NONE',  ( 10.28180685320999999, -3.991526694881000203, -5.814304247846999729 ) ) ;
#61505=ORIENTED_EDGE ( 'NONE', *, *, #32993, .F. ) ;
#61508=( NAMED_UNIT ( * ) PLANE_ANGLE_UNIT ( ) SI_UNIT ( $, .RADIAN. ) );
#61509=CARTESIAN_POINT ( 'NONE',  ( 8.417227077245023281, -3.802951429257032334, 6.016322095508296108 ) ) ;
#61512=VECTOR ( 'NONE', #13288, 1000.000000000000114 ) ;
#61515=FACE_OUTER_BOUND ( 'NONE', #63860, .T. ) ;
#61519=ORIENTED_EDGE ( 'NONE', *, *, #10835, .F. ) ;
#61529=EDGE_CURVE ( 'NONE', #21554, #64636, #21783, .T. ) ;
#61530=ORIENTED_EDGE ( 'NONE', *, *, #25957, .F. ) ;
#61546=CARTESIAN_POINT ( 'NONE',  ( 9.417725536554337751, -5.345107907813670067, 7.385006124088557833 ) ) ;
#61547=CARTESIAN_POINT ( 'NONE',  ( 7.373066940378000034, -3.394845988290999816, 9.388942682504000103 ) ) ;
#61558=CARTESIAN_POINT ( 'NONE',  ( 10.79692742076994527, -5.515504571040683146, -6.594679436486475588 ) ) ;
#61561=VECTOR ( 'NONE', #4568, 1000.000000000000114 ) ;
#61562=CARTESIAN_POINT ( 'NONE',  ( 8.712568288355884150, -5.100000000000000533, 6.329675358928077422 ) ) ;
#61581=CARTESIAN_POINT ( 'NONE',  ( 9.534903635507999908, -3.030945724184999968, 8.761987396837000119 ) ) ;
#61583=CARTESIAN_POINT ( 'NONE',  ( 10.24845588172999911, -4.234132110154000372, -5.660862927546999934 ) ) ;
#61585=CARTESIAN_POINT ( 'NONE',  ( 10.61503919148196218, -5.349978903665073560, -7.499997722305344006 ) ) ;
#61588=CARTESIAN_POINT ( 'NONE',  ( 11.02035356290999957, -6.428762174806000651, -5.279064955367999801 ) ) ;
#61594=CARTESIAN_POINT ( 'NONE',  ( 11.20563089100999932, -3.509133048232999652, 6.118191305996999674 ) ) ;
#61598=ORIENTED_EDGE ( 'NONE', *, *, #20481, .T. ) ;
#61608=B_SPLINE_CURVE_WITH_KNOTS ( 'NONE', 3,
 ( #54229, #38147, #17880, #33614 ),
 .UNSPECIFIED., .F., .F.,
 ( 4, 4 ),
 ( 0.000000000000000000, 1.000000000000000000 ),
 .UNSPECIFIED. ) ;
#61617=VERTEX_POINT ( 'NONE', #24485 ) ;
#61620=CARTESIAN_POINT ( 'NONE',  ( 9.972852379787999766, -5.044471434015000533, 6.258101649750000384 ) ) ;
#61624=CARTESIAN_POINT ( 'NONE',  ( 10.90540321535548429, -2.790089835004903041, -6.887843015913232669 ) ) ;
#61633=CARTESIAN_POINT ( 'NONE',  ( 10.96922972661000095, -2.855437608211000011, 5.027789437851001075 ) ) ;
#61636=CARTESIAN_POINT ( 'NONE',  ( 9.751909913808001207, -4.316974633926000671, -5.653758079558000027 ) ) ;
#61653=ORIENTED_EDGE ( 'NONE', *, *, #56436, .T. ) ;
#61659=CARTESIAN_POINT ( 'NONE',  ( 27.64127793187000037, -5.599999999999999645, 6.571291218949999902 ) ) ;
#61675=CARTESIAN_POINT ( 'NONE',  ( 9.408936720234443385, -2.481771157840773512, 8.348873588805004076 ) ) ;
#61678=CARTESIAN_POINT ( 'NONE',  ( 9.907296092384241248, -5.171595203895851256, -8.821442009999598710 ) ) ;
#61679=CARTESIAN_POINT ( 'NONE',  ( 10.88207481814999866, -5.063049640536999796, -5.075897427045000576 ) ) ;
#61683=CARTESIAN_POINT ( 'NONE',  ( 9.691080333872001518, -5.335644368206000188, 8.701217921043999937 ) ) ;
#61685=CARTESIAN_POINT ( 'NONE',  ( 10.90000000000000036, -2.899999999999999911, 6.414037451299000381 ) ) ;
#61687=VERTEX_POINT ( 'NONE', #34895 ) ;
#61696=CARTESIAN_POINT ( 'NONE',  ( 8.734653236333999260, -4.846210315537001101, -6.250999225331006492 ) ) ;
#61697=ORIENTED_EDGE ( 'NONE', *, *, #46287, .F. ) ;
#61698=VECTOR ( 'NONE', #6661, 1000.000000000000000 ) ;
#61700=DIRECTION ( 'NONE',  ( 1.000000000000000000, 0.000000000000000000, 0.000000000000000000 ) ) ;
#61703=CARTESIAN_POINT ( 'NONE',  ( 9.490308298768001194, -5.536248950452999473, -7.355084988757000453 ) ) ;
#61708=CARTESIAN_POINT ( 'NONE',  ( 8.328787166962994704, -5.102611464338999703, 6.655261220345003004 ) ) ;
#61713=ORIENTED_EDGE ( 'NONE', *, *, #30419, .F. ) ;
#61715=CARTESIAN_POINT ( 'NONE',  ( 7.810193361277576685, -3.081125311113132703, 6.468046414883829698 ) ) ;
#61718=CARTESIAN_POINT ( 'NONE',  ( 10.01293113571299997, -5.100000000000000533, 6.444141223344916014 ) ) ;
#61719=EDGE_LOOP ( 'NONE', ( #5222, #49872, #15988, #15177, #39161 ) ) ;
#61727=CARTESIAN_POINT ( 'NONE',  ( 9.778462793022999477, -5.743713977826000239, 7.748300060190000060 ) ) ;
#61730=FACE_OUTER_BOUND ( 'NONE', #38179, .T. ) ;
#61734=CARTESIAN_POINT ( 'NONE',  ( 11.08380555355832620, -3.999999927290649460, -9.033895164528411570 ) ) ;
#61736=B_SPLINE_CURVE_WITH_KNOTS ( 'NONE', 3,
 ( #43813, #65108, #49740, #17233 ),
 .UNSPECIFIED., .F., .F.,
 ( 4, 4 ),
 ( 0.000000000000000000, 0.1254138569076999055 ),
 .UNSPECIFIED. ) ;
#61739=ORIENTED_EDGE ( 'NONE', *, *, #34188, .T. ) ;
#61740=CARTESIAN_POINT ( 'NONE',  ( 10.15402496696000156, -5.267980706381999667, 5.992344456606999437 ) ) ;
#61745=CARTESIAN_POINT ( 'NONE',  ( 11.03775575519999919, -8.050335494570999728, 6.914609630061999468 ) ) ;
#61749=ADVANCED_FACE ( 'NONE', ( #49329 ), #17166, .F. ) ;
#61758=VERTEX_POINT ( 'NONE', #16481 ) ;
#61764=B_SPLINE_CURVE_WITH_KNOTS ( 'NONE', 3,
 ( #50353, #40889, #18195, #60842 ),
 .UNSPECIFIED., .F., .F.,
 ( 4, 4 ),
 ( 0.000000000000000000, 1.000000000000000000 ),
 .UNSPECIFIED. ) ;
#61765=CARTESIAN_POINT ( 'NONE',  ( 10.07930721860999945, -2.718124813223000036, -6.397797539448999871 ) ) ;
#61767=CARTESIAN_POINT ( 'NONE',  ( 9.660601868375998436, -2.901236202253999696, -6.151180522693000086 ) ) ;
#61772=CARTESIAN_POINT ( 'NONE',  ( 7.437254440376999121, -2.216884807317999861, 8.370075800106999253 ) ) ;
#61785=ORIENTED_EDGE ( 'NONE', *, *, #56493, .F. ) ;
#61786=CARTESIAN_POINT ( 'NONE',  ( 8.347269353210000631, -2.741638482234999952, 6.457327039244000311 ) ) ;
#61792=CYLINDRICAL_SURFACE ( 'NONE', #43704, 0.5000000000000002220 ) ;
#61798=CARTESIAN_POINT ( 'NONE',  ( 8.131285109058133287, -8.951598720774811113, -5.991666729276850845 ) ) ;
#61801=CARTESIAN_POINT ( 'NONE',  ( 10.40685100253999984, -2.832432432432000269, -6.822293592207000934 ) ) ;
#61803=CARTESIAN_POINT ( 'NONE',  ( 10.98768538770000092, -2.700669876604000041, 4.945210823433001224 ) ) ;
#61806=CARTESIAN_POINT ( 'NONE',  ( 10.98768472639999949, -0.3876847264043000174, 4.945212061661000469 ) ) ;
#61807=CARTESIAN_POINT ( 'NONE',  ( 10.14521814679000045, -3.576528389491000048, -8.962725485696999783 ) ) ;
#61808=CARTESIAN_POINT ( 'NONE',  ( 8.064837199433295467, -3.781904628662576151, 5.773930963923838533 ) ) ;
#61812=VERTEX_POINT ( 'NONE', #64707 ) ;
#61813=CARTESIAN_POINT ( 'NONE',  ( 10.98974733714999985, -5.155859329793999635, -5.102561852530000053 ) ) ;
#61819=CARTESIAN_POINT ( 'NONE',  ( 9.710316810687000810, -2.624921803719999946, -8.200122328058998988 ) ) ;
#61828=CARTESIAN_POINT ( 'NONE',  ( 8.598668146794999245, -2.376522687267000222, 7.686981355459999499 ) ) ;
#61830=ORIENTED_EDGE ( 'NONE', *, *, #46926, .T. ) ;
#61834=CARTESIAN_POINT ( 'NONE',  ( 11.15264435320999858, -2.317067032475999877, -7.596564138533999255 ) ) ;
#61839=ADVANCED_FACE ( 'NONE', ( #54931 ), #38498, .T. ) ;
#61850=DIRECTION ( 'NONE',  ( 0.000000000000000000, 1.000000000000000000, 0.000000000000000000 ) ) ;
#61854=CARTESIAN_POINT ( 'NONE',  ( 10.22963300084641780, -4.176697648610067759, -8.850191834421890391 ) ) ;
#61867=ORIENTED_EDGE ( 'NONE', *, *, #35794, .F. ) ;
#61872=EDGE_CURVE ( 'NONE', #39743, #68200, #49682, .T. ) ;
#61875=CARTESIAN_POINT ( 'NONE',  ( 8.277730646792999636, -4.874569256861000177, 6.119503992241999590 ) ) ;
#61890=CARTESIAN_POINT ( 'NONE',  ( 8.528441940379998698, -2.472358291268000219, 6.234202627038999189 ) ) ;
#61895=CARTESIAN_POINT ( 'NONE',  ( 7.450093581731485060, -2.260954841078268274, 7.477861549239195327 ) ) ;
#61899=ORIENTED_EDGE ( 'NONE', *, *, #14220, .F. ) ;
#61912=ORIENTED_EDGE ( 'NONE', *, *, #25957, .T. ) ;
#61914=CARTESIAN_POINT ( 'NONE',  ( 10.20271159698171815, -5.100000000000000533, 6.305985889763628727 ) ) ;
#61916=ORIENTED_EDGE ( 'NONE', *, *, #68744, .F. ) ;
#61924=CARTESIAN_POINT ( 'NONE',  ( 10.29378083128999855, -3.483628580733000302, 6.176326635498999629 ) ) ;
#61926=EDGE_CURVE ( 'NONE', #53120, #32339, #18910, .T. ) ;
#61936=CARTESIAN_POINT ( 'NONE',  ( 10.73165287102650822, -3.320185038362776897, -8.679412628036383026 ) ) ;
#61940=ORIENTED_EDGE ( 'NONE', *, *, #45724, .F. ) ;
#61943=ORIENTED_EDGE ( 'NONE', *, *, #54290, .F. ) ;
#61946=CARTESIAN_POINT ( 'NONE',  ( 8.620740978634000129, -4.599999999999999645, 5.898823289756999877 ) ) ;
#61948=AXIS2_PLACEMENT_3D ( 'NONE', #44440, #65738, #60848 ) ;
#61950=FACE_OUTER_BOUND ( 'NONE', #54945, .T. ) ;
#61956=CARTESIAN_POINT ( 'NONE',  ( 5.599999999999999645, -0.4000000000000000222, -6.406472342878999804 ) ) ;
#61970=CARTESIAN_POINT ( 'NONE',  ( 9.848732933287999813, -2.769734897491000325, 6.441850735262000249 ) ) ;
#61973=CARTESIAN_POINT ( 'NONE',  ( 11.10000000009000054, -2.699999999911000259, 6.571291220400000022 ) ) ;
#61977=EDGE_CURVE ( 'NONE', #46269, #67865, #50896, .T. ) ;
#61981=ADVANCED_FACE ( 'NONE', ( #12116 ), #23981, .F. ) ;
#61983=CARTESIAN_POINT ( 'NONE',  ( 8.538555273383003907, -3.514476186897000254, -6.517616047691000780 ) ) ;
#61986=CARTESIAN_POINT ( 'NONE',  ( 9.040134009213000255, -5.099406281193999746, -6.669356233738001016 ) ) ;
#62017=AXIS2_PLACEMENT_3D ( 'NONE', #1976, #55456, #65588 ) ;
#62029=CARTESIAN_POINT ( 'NONE',  ( 10.84088306584999906, -2.636277440143000472, -7.512643837511999934 ) ) ;
#62043=ORIENTED_EDGE ( 'NONE', *, *, #15529, .F. ) ;
#62044=CYLINDRICAL_SURFACE ( 'NONE', #26934, 0.4999999999999998335 ) ;
#62047=CARTESIAN_POINT ( 'NONE',  ( 9.578311703535998589, -4.818302824158000597, -8.808202952968999355 ) ) ;
#62072=CARTESIAN_POINT ( 'NONE',  ( 10.53733998880999856, -2.992814141720000265, 8.731692578598000409 ) ) ;
#62075=CARTESIAN_POINT ( 'NONE',  ( 7.854816940377000734, -4.561648098548999997, 6.153050355516999304 ) ) ;
#62087=CARTESIAN_POINT ( 'NONE',  ( 10.53865751177000121, -3.647233463439000012, -6.014125921456000334 ) ) ;
#62101=ORIENTED_EDGE ( 'NONE', *, *, #25572, .F. ) ;
#62108=CARTESIAN_POINT ( 'NONE',  ( 11.03407957707000087, -2.992853177526999975, -9.056567163506000995 ) ) ;
#62115=EDGE_CURVE ( 'NONE', #24689, #10513, #12508, .T. ) ;
#62120=EDGE_CURVE ( 'NONE', #5301, #41119, #49737, .T. ) ;
#62127=VERTEX_POINT ( 'NONE', #48018 ) ;
#62128=CARTESIAN_POINT ( 'NONE',  ( 9.079730646793999327, -5.421531391267000011, 6.381128921159999301 ) ) ;
#62150=CARTESIAN_POINT ( 'NONE',  ( 8.254401249163198173, -5.347345989532893640, 8.600472902534793462 ) ) ;
#62154=CARTESIAN_POINT ( 'NONE',  ( 10.88897495225000078, -5.158582900058999776, -5.064471961637000419 ) ) ;
#62159=CARTESIAN_POINT ( 'NONE',  ( 9.265134009212999899, -5.494586520014999920, -6.370782351137999733 ) ) ;
#62168=CARTESIAN_POINT ( 'NONE',  ( 8.251331853209000755, -5.773185758034999893, 7.141496747382000798 ) ) ;
#62173=CARTESIAN_POINT ( 'NONE',  ( 10.84974435320999930, -5.265000209383999596, -6.385811305909999902 ) ) ;
#62179=EDGE_CURVE ( 'NONE', #66731, #42529, #36653, .T. ) ;
#62184=ORIENTED_EDGE ( 'NONE', *, *, #56493, .T. ) ;
#62186=ORIENTED_EDGE ( 'NONE', *, *, #564, .T. ) ;
#62188=VECTOR ( 'NONE', #64143, 1000.000000000000000 ) ;
#62189=FACE_OUTER_BOUND ( 'NONE', #33978, .T. ) ;
#62194=CARTESIAN_POINT ( 'NONE',  ( 8.871383953235001840, -4.600000082569999371, -6.206578679665999410 ) ) ;
#62197=CARTESIAN_POINT ( 'NONE',  ( 10.36503728015203230, -2.650011783303574564, -7.500002219258004921 ) ) ;
#62208=B_SPLINE_CURVE_WITH_KNOTS ( 'NONE', 3,
 ( #58594, #22564, #53011, #37611 ),
 .UNSPECIFIED., .F., .F.,
 ( 4, 4 ),
 ( 0.000000000000000000, 1.000000000000000000 ),
 .UNSPECIFIED. ) ;
#62216=CARTESIAN_POINT ( 'NONE',  ( 8.058769353207999586, -2.432121990576000314, 6.597519606637999523 ) ) ;
#62217=DIRECTION ( 'NONE',  ( 1.000000000000000000, 0.000000000000000000, 0.000000000000000000 ) ) ;
#62220=ORIENTED_EDGE ( 'NONE', *, *, #21380, .T. ) ;
#62223=EDGE_CURVE ( 'NONE', #22085, #61617, #5804, .T. ) ;
#62226=DIRECTION ( 'NONE',  ( 1.000000000000000000, 1.776356839362000177E-14, 5.329070518085999900E-14 ) ) ;
#62228=ADVANCED_FACE ( 'NONE', ( #38558 ), #27383, .F. ) ;
#62232=CARTESIAN_POINT ( 'NONE',  ( 8.630418146794999856, -5.808258301303999893, 7.446016267012000256 ) ) ;
#62237=CARTESIAN_POINT ( 'NONE',  ( 7.580200994261414138, -4.132977011570006631, 5.765716077822864882 ) ) ;
#62241=ORIENTED_EDGE ( 'NONE', *, *, #17839, .F. ) ;
#62249=CARTESIAN_POINT ( 'NONE',  ( 8.620740978634000129, -4.599999999999999645, 5.898823289756999877 ) ) ;
#62258=DIRECTION ( 'NONE',  ( 0.000000000000000000, 1.000000000000000000, 0.000000000000000000 ) ) ;
#62264=CARTESIAN_POINT ( 'NONE',  ( 11.07345355053000091, -3.998673159585000025, 8.920828114954002075 ) ) ;
#62265=EDGE_CURVE ( 'NONE', #18362, #65751, #48711, .T. ) ;
#62274=CARTESIAN_POINT ( 'NONE',  ( 10.96507314189000049, -5.561950019225000652, -4.905737662152000134 ) ) ;
#62293=VECTOR ( 'NONE', #51987, 1000.000000000000114 ) ;
#62294=CARTESIAN_POINT ( 'NONE',  ( 10.26685100253999927, -2.832432432432000269, 6.822293592207000934 ) ) ;
#62316=CARTESIAN_POINT ( 'NONE',  ( 9.496463691918865635, -5.100000000000000533, -6.665341197415688868 ) ) ;
#62318=B_SPLINE_CURVE_WITH_KNOTS ( 'NONE', 3,
 ( #53038, #19848, #10720, #46765, #20529, #41177, #62484, #5134, #9339, #15969, #53384, #35925, #57238, #68068, #20184, #36267 ),
 .UNSPECIFIED., .F., .F.,
 ( 4, 2, 2, 1, 1, 2, 2, 2, 4 ),
 ( 0.000000000000000000, 0.2499999999999763522, 0.3749999999999656941, 0.4374999999999591438, 0.4687499999999563127, 0.4843749999999565903, 0.4999999999999568123, 0.7499999999999784617, 1.000000000000000000 ),
 .UNSPECIFIED. ) ;
#62324=CARTESIAN_POINT ( 'NONE',  ( 11.13500760274999912, -2.665983503042999914, 5.187970728494999406 ) ) ;
#62329=CARTESIAN_POINT ( 'NONE',  ( 9.475279990687656806, -5.350441389720279162, 7.499985493516659218 ) ) ;
#62333=CARTESIAN_POINT ( 'NONE',  ( 9.115000000004000569, -5.349999999999999645, -7.500000000000000000 ) ) ;
#62336=ORIENTED_EDGE ( 'NONE', *, *, #4952, .T. ) ;
#62337=CARTESIAN_POINT ( 'NONE',  ( 8.632946129846605032, -2.796778970782837437, 8.203843119991294230 ) ) ;
#62369=ADVANCED_FACE ( 'NONE', ( #8130 ), #17059, .F. ) ;
#62372=CARTESIAN_POINT ( 'NONE',  ( 10.56591477248000110, -5.293237054095000005, -7.067083954277999958 ) ) ;
#62373=VERTEX_POINT ( 'NONE', #52141 ) ;
#62386=CARTESIAN_POINT ( 'NONE',  ( 10.38001771741999946, -3.294294314927000311, -5.012847088973000353 ) ) ;
#62387=CARTESIAN_POINT ( 'NONE',  ( 9.353137413980999071, -5.679455740088000582, -8.329752476417999318 ) ) ;
#62406=FACE_OUTER_BOUND ( 'NONE', #12372, .T. ) ;
#62412=ORIENTED_EDGE ( 'NONE', *, *, #15939, .T. ) ;
#62413=CARTESIAN_POINT ( 'NONE',  ( 11.27765354842000001, -3.273798832483999721, 6.368296067120999382 ) ) ;
#62416=CARTESIAN_POINT ( 'NONE',  ( 9.266941940380000631, -3.049610585291000042, 6.392533570808999421 ) ) ;
#62425=CARTESIAN_POINT ( 'NONE',  ( 11.27109998545999936, -5.469594811916000054, 8.504700858852999090 ) ) ;
#62431=CARTESIAN_POINT ( 'NONE',  ( 10.25166529434999951, -3.418639857622999934, -8.733652610425998830 ) ) ;
#62433=ORIENTED_EDGE ( 'NONE', *, *, #2855, .T. ) ;
#62441=CARTESIAN_POINT ( 'NONE',  ( 7.915155411429996235, -5.089315853099998677, 6.494606418034001294 ) ) ;
#62444=EDGE_CURVE ( 'NONE', #40213, #17921, #25881, .T. ) ;
#62455=CARTESIAN_POINT ( 'NONE',  ( 11.09999999999999964, -2.274006712557999688, -7.281956340829000673 ) ) ;
#62468=CARTESIAN_POINT ( 'NONE',  ( 8.064120559623999540, -4.228293421747000735, 8.941387937291999322 ) ) ;
#62475=ADVANCED_FACE ( 'NONE', ( #40974 ), #40624, .T. ) ;
#62477=ADVANCED_FACE ( 'NONE', ( #56720 ), #8815, .F. ) ;
#62484=CARTESIAN_POINT ( 'NONE',  ( 7.834511717026050093, -4.924825534011793238, 6.461662825486788719 ) ) ;
#62486=CARTESIAN_POINT ( 'NONE',  ( 8.276895518193162715, -4.975196787739221804, 8.941828154844815302 ) ) ;
#62493=CARTESIAN_POINT ( 'NONE',  ( 7.307500000000000107, -0.2999999999999999889, -3.149999999999999911 ) ) ;
#62495=DIRECTION ( 'NONE',  ( 0.000000000000000000, 1.000000000000000000, 0.000000000000000000 ) ) ;
#62496=LINE ( 'NONE', #41524, #19340 ) ;
#62502=EDGE_CURVE ( 'NONE', #3171, #28855, #19653, .T. ) ;
#62503=ADVANCED_FACE ( 'NONE', ( #30130 ), #47752, .T. ) ;
#62508=CARTESIAN_POINT ( 'NONE',  ( 8.610058059625000482, -5.329429281359999493, 6.027400270608000099 ) ) ;
#62514=CARTESIAN_POINT ( 'NONE',  ( 10.97819314679000158, -5.476828481365000556, -7.128717489481000591 ) ) ;
#62521=CARTESIAN_POINT ( 'NONE',  ( 8.517841509200911432, -5.092672768596408162, 6.425478427622871358 ) ) ;
#62534=CARTESIAN_POINT ( 'NONE',  ( 8.665068710487354053, -4.836047963814035455, -6.439919795970022065 ) ) ;
#62544=B_SPLINE_CURVE_WITH_KNOTS ( 'NONE', 3,
 ( #18737, #28544, #66958, #19065 ),
 .UNSPECIFIED., .F., .F.,
 ( 4, 4 ),
 ( 0.000000000000000000, 1.000000000000000000 ),
 .UNSPECIFIED. ) ;
#62562=LINE ( 'NONE', #57318, #25736 ) ;
#62568=CARTESIAN_POINT ( 'NONE',  ( 27.64127793187000037, -5.599999999999999645, 6.571291218949999902 ) ) ;
#62569=CARTESIAN_POINT ( 'NONE',  ( 8.052730646792999991, -4.968144979409999884, 5.971795951526999602 ) ) ;
#62573=CARTESIAN_POINT ( 'NONE',  ( 9.964045559621999004, -3.485908552077000344, -9.275738075927998594 ) ) ;
#62574=CARTESIAN_POINT ( 'NONE',  ( 7.590451290858640121, -4.346862521704085935, 5.795392881046511846 ) ) ;
#62598=CARTESIAN_POINT ( 'NONE',  ( 10.51654446536000087, -4.930670681812999945, 8.573593359022000371 ) ) ;
#62600=CARTESIAN_POINT ( 'NONE',  ( 10.60198654464000079, -2.164987663130000239, -7.764523632348000248 ) ) ;
#62606=CARTESIAN_POINT ( 'NONE',  ( 11.12373728587000166, -6.332991536706000346, -5.421362649029999758 ) ) ;
#62607=DIRECTION ( 'NONE',  ( 0.000000000000000000, -0.2461538461537955691, -0.9692307692307821076 ) ) ;
#62626=CARTESIAN_POINT ( 'NONE',  ( 9.883915020958999875, -5.811247906278000031, -7.978055797018001272 ) ) ;
#62639=CARTESIAN_POINT ( 'NONE',  ( 10.06844525594999951, -4.148609764890999863, 8.941457795715999524 ) ) ;
#62642=EDGE_CURVE ( 'NONE', #68200, #10649, #55850, .T. ) ;
#62655=CARTESIAN_POINT ( 'NONE',  ( 10.42787890655380600, -4.833579956562179980, -4.974657529990448523 ) ) ;
#62658=CARTESIAN_POINT ( 'NONE',  ( 10.86297706979999944, -2.934528160336999925, 5.173578227060000145 ) ) ;
#62661=CARTESIAN_POINT ( 'NONE',  ( 11.13224602605999891, -2.668757901739000182, -5.057295448712999963 ) ) ;
#62662=CARTESIAN_POINT ( 'NONE',  ( 9.900941392955999731, -4.883847137081999357, -9.070879136699002032 ) ) ;
#62666=CARTESIAN_POINT ( 'NONE',  ( 9.188234083221837878, -2.648243641808896598, 7.263637137173924785 ) ) ;
#62672=CARTESIAN_POINT ( 'NONE',  ( 8.434805295391802460, -5.349284795551668914, 7.676787393164613782 ) ) ;
#62693=EDGE_CURVE ( 'NONE', #41892, #46269, #35786, .T. ) ;
#62704=CARTESIAN_POINT ( 'NONE',  ( 11.06133683778999988, -2.503914237677999921, -6.712780725818999983 ) ) ;
#62716=EDGE_LOOP ( 'NONE', ( #54742, #31705, #45296, #56762 ) ) ;
#62718=CARTESIAN_POINT ( 'NONE',  ( 8.205380712518003605, -3.106081630192000009, 6.107045428706002532 ) ) ;
#62728=VECTOR ( 'NONE', #15887, 999.9999999999998863 ) ;
#62729=CARTESIAN_POINT ( 'NONE',  ( 10.86501009699205866, -2.649983380499685737, -7.500000587580680111 ) ) ;
#62737=DIRECTION ( 'NONE',  ( 0.000000000000000000, -1.000000000000000000, 0.000000000000000000 ) ) ;
#62739=ORIENTED_EDGE ( 'NONE', *, *, #50752, .T. ) ;
#62740=DIRECTION ( 'NONE',  ( -0.1522489053782972723, 0.9525130357304880668, -0.2637028395269958025 ) ) ;
#62749=CARTESIAN_POINT ( 'NONE',  ( 10.20319453770999907, -3.421758889707999796, 6.017729046583999875 ) ) ;
#62752=CARTESIAN_POINT ( 'NONE',  ( 9.368918146792999835, -5.618388245857000030, 7.727743016644000207 ) ) ;
#62753=CONICAL_SURFACE ( 'NONE', #11399, 0.8999999993279991228, 0.7853981633972997312 ) ;
#62766=CARTESIAN_POINT ( 'NONE',  ( 10.99693800072000016, -2.980603239157999962, -6.418614998350999912 ) ) ;
#62777=ORIENTED_EDGE ( 'NONE', *, *, #35203, .T. ) ;
#62778=CARTESIAN_POINT ( 'NONE',  ( 7.810726116476000236, -5.086048788582002267, 6.527219528731996512 ) ) ;
#62785=B_SPLINE_CURVE_WITH_KNOTS ( 'NONE', 3,
 ( #21950, #54115, #17408, #11460 ),
 .UNSPECIFIED., .F., .F.,
 ( 4, 4 ),
 ( 0.000000000000000000, 1.000000000000000000 ),
 .UNSPECIFIED. ) ;
#62786=CARTESIAN_POINT ( 'NONE',  ( 9.856713838269000050, -4.814118338972999567, -8.929571672388000536 ) ) ;
#62788=CARTESIAN_POINT ( 'NONE',  ( 9.316610756102749136, -5.674809202490012083, -6.995745383024254416 ) ) ;
#62796=CIRCLE ( 'NONE', #25984, 1.099999999999999867 ) ;
#62806=ORIENTED_EDGE ( 'NONE', *, *, #8279, .T. ) ;
#62807=CARTESIAN_POINT ( 'NONE',  ( 7.127706853208000126, -4.698358408974000255, 8.789434435623999065 ) ) ;
#62826=CARTESIAN_POINT ( 'NONE',  ( 8.255343399658274350, -5.333771483169611471, 8.616868296190860477 ) ) ;
#62829=CARTESIAN_POINT ( 'NONE',  ( 10.36332605023000042, -4.728604826508999714, -4.865787476787999388 ) ) ;
#62834=ORIENTED_EDGE ( 'NONE', *, *, #56040, .T. ) ;
#62835=VECTOR ( 'NONE', #23864, 1000.000000000000000 ) ;
#62845=STYLED_ITEM ( 'NONE', ( #37314 ), #29488 ) ;
#62846=CARTESIAN_POINT ( 'NONE',  ( 8.674245559624999657, -5.983034890242000081, 7.440798487724999966 ) ) ;
#62851=CARTESIAN_POINT ( 'NONE',  ( 10.71315564678999976, -2.619204038425999581, -8.142086897834001746 ) ) ;
#62888=EDGE_CURVE ( 'NONE', #57184, #5900, #21249, .T. ) ;
#62890=CARTESIAN_POINT ( 'NONE',  ( 10.95387080750653652, -2.254039244220492844, 7.421505705631724403 ) ) ;
#62900=CYLINDRICAL_SURFACE ( 'NONE', #21286, 1.350000000000000089 ) ;
#62906=CARTESIAN_POINT ( 'NONE',  ( 7.239688980126000040, -4.389298280625000714, 9.135255728583000945 ) ) ;
#62910=CARTESIAN_POINT ( 'NONE',  ( 10.41839555962000041, -4.531908721143000029, -9.270473926467998282 ) ) ;
#62911=CARTESIAN_POINT ( 'NONE',  ( 7.576990885774728568, -4.064377392965215385, 5.762023686569064829 ) ) ;
#62914=ORIENTED_EDGE ( 'NONE', *, *, #30478, .T. ) ;
#62925=AXIS2_PLACEMENT_3D ( 'NONE', #18098, #39073, #39417 ) ;
#62936=CARTESIAN_POINT ( 'NONE',  ( 10.89228096335999929, -3.998355205482000851, 9.261304730013998565 ) ) ;
#62942=FACE_OUTER_BOUND ( 'NONE', #17875, .T. ) ;
#62948=ADVANCED_FACE ( 'NONE', ( #5851 ), #22279, .F. ) ;
#62949=CARTESIAN_POINT ( 'NONE',  ( 10.41185831014999863, -2.101597930377999912, 7.856264717901999539 ) ) ;
#62956=CARTESIAN_POINT ( 'NONE',  ( 9.228135700785001561, -2.875364528161000077, 8.669943154892999715 ) ) ;
#62960=DIRECTION ( 'NONE',  ( 1.000000000000000000, 0.000000000000000000, 0.000000000000000000 ) ) ;
#62963=CARTESIAN_POINT ( 'NONE',  ( 9.971918425727000823, -4.365624317997999881, -9.242254741729000855 ) ) ;
#62986=CARTESIAN_POINT ( 'NONE',  ( 10.48676300414402185, -4.912662277004227640, -4.994045588562562088 ) ) ;
#62991=VECTOR ( 'NONE', #65935, 1000.000000000000114 ) ;
#62994=CARTESIAN_POINT ( 'NONE',  ( 11.04647087182000043, -2.754739992437999607, -5.117584562748000110 ) ) ;
#62995=CARTESIAN_POINT ( 'NONE',  ( 11.17788601987000163, -2.412142864687000010, -7.075602314719000141 ) ) ;
#63000=CARTESIAN_POINT ( 'NONE',  ( 9.101049665823000012, -5.350000000000001421, -7.263338156157798764 ) ) ;
#63004=ORIENTED_EDGE ( 'NONE', *, *, #13606, .F. ) ;
#63020=ORIENTED_EDGE ( 'NONE', *, *, #17670, .F. ) ;
#63028=CARTESIAN_POINT ( 'NONE',  ( 11.11772401304000013, -8.026951646845001065, -6.811579381709000458 ) ) ;
#63029=ORIENTED_EDGE ( 'NONE', *, *, #16777, .T. ) ;
#63038=CARTESIAN_POINT ( 'NONE',  ( 10.89218817467000200, -2.661900611977999986, -8.236035141896001832 ) ) ;
#63050=CARTESIAN_POINT ( 'NONE',  ( 8.076856445596000356, -2.879480170456998778, 6.727212843387002650 ) ) ;
#63053=CARTESIAN_POINT ( 'NONE',  ( 10.39853701727000157, -3.107293017143999858, -4.742114626611999562 ) ) ;
#63057=CARTESIAN_POINT ( 'NONE',  ( 9.194602547868999665, -5.157768569202000108, 8.637845986715998237 ) ) ;
#63077=DIRECTION ( 'NONE',  ( 0.000000000000000000, 0.8648648648648720183, -0.5020047465136825426 ) ) ;
#63081=FACE_OUTER_BOUND ( 'NONE', #35243, .T. ) ;
#63085=CARTESIAN_POINT ( 'NONE',  ( 11.11504459742000073, -3.456612073675000119, 5.970342812640000218 ) ) ;
#63087=CARTESIAN_POINT ( 'NONE',  ( 8.495897545620808344, -3.117844663886039758, 6.071417532389746796 ) ) ;
#63088=CARTESIAN_POINT ( 'NONE',  ( 7.481081853206999810, -2.374041291348000016, 8.293390875797999939 ) ) ;
#63098=CARTESIAN_POINT ( 'NONE',  ( 9.504901164121001500, -3.934733502342999678, 5.704835336325999151 ) ) ;
#63127=CARTESIAN_POINT ( 'NONE',  ( 9.274684250042126266, -5.195247215952409903, -6.222724923390055451 ) ) ;
#63134=CARTESIAN_POINT ( 'NONE',  ( 7.448644353207000357, -4.628942671846000501, 5.991663889842000046 ) ) ;
#63139=DIRECTION ( 'NONE',  ( 1.000000000000000000, 0.000000000000000000, 0.000000000000000000 ) ) ;
#63147=CARTESIAN_POINT ( 'NONE',  ( 7.448644353207000357, -4.628942671846000501, 5.991663889842000046 ) ) ;
#63158=EDGE_CURVE ( 'NONE', #16743, #46332, #52311, .T. ) ;
#63164=CARTESIAN_POINT ( 'NONE',  ( 8.236412180507333147, -5.557254354115385375, 8.275240123836031358 ) ) ;
#63169=ORIENTED_EDGE ( 'NONE', *, *, #23684, .F. ) ;
#63184=AXIS2_PLACEMENT_3D ( 'NONE', #25475, #46807, #61850 ) ;
#63198=EDGE_CURVE ( 'NONE', #31672, #3964, #53179, .T. ) ;
#63220=B_SPLINE_CURVE_WITH_KNOTS ( 'NONE', 3,
 ( #28197, #55806, #18746, #7554 ),
 .UNSPECIFIED., .F., .F.,
 ( 4, 4 ),
 ( 0.000000000000000000, 1.000000000000000000 ),
 .UNSPECIFIED. ) ;
#63228=VERTEX_POINT ( 'NONE', #45686 ) ;
#63232=DIRECTION ( 'NONE',  ( -1.000000000000000000, 0.000000000000000000, 0.000000000000000000 ) ) ;
#63248=CARTESIAN_POINT ( 'NONE',  ( 10.71685100253999856, -2.832432432432000269, 6.822293592207000934 ) ) ;
#63249=CARTESIAN_POINT ( 'NONE',  ( 7.705394353206999725, -3.245532552444000185, 8.949627348471000943 ) ) ;
#63254=CARTESIAN_POINT ( 'NONE',  ( 9.926183059621999760, -4.356410583133000003, -9.313949118577001585 ) ) ;
#63255=CARTESIAN_POINT ( 'NONE',  ( 7.484823115406580740, -2.425454210375729502, 6.760261958790284353 ) ) ;
#63281=CARTESIAN_POINT ( 'NONE',  ( 9.332935524889000689, -5.100347267927999972, 8.693464469215999912 ) ) ;
#63289=ORIENTED_EDGE ( 'NONE', *, *, #38135, .F. ) ;
#63291=CARTESIAN_POINT ( 'NONE',  ( 9.625409048293999348, -2.899999999999999911, -6.226580113766999602 ) ) ;
#63293=LINE ( 'NONE', #36746, #61561 ) ;
#63304=CARTESIAN_POINT ( 'NONE',  ( 10.90374822854000136, -3.726845778959999578, 5.900452123196999743 ) ) ;
#63319=ORIENTED_EDGE ( 'NONE', *, *, #13632, .T. ) ;
#63343=CARTESIAN_POINT ( 'NONE',  ( 9.443897997121000643, -4.993413662857000723, -9.088148847710000311 ) ) ;
#63344=CARTESIAN_POINT ( 'NONE',  ( 10.68343305961999867, -3.810133104029999718, -5.661126601970999594 ) ) ;
#63345=CARTESIAN_POINT ( 'NONE',  ( 9.174642513462206495, -2.649442673322992103, 7.499981897072125925 ) ) ;
#63346=CARTESIAN_POINT ( 'NONE',  ( 7.896812975353013186, -5.287194663100612146, 7.026484571482168207 ) ) ;
#63356=B_SPLINE_CURVE_WITH_KNOTS ( 'NONE', 3,
 ( #15706, #32142, #37035, #53456 ),
 .UNSPECIFIED., .F., .F.,
 ( 4, 4 ),
 ( 0.000000000000000000, 1.000000000000000000 ),
 .UNSPECIFIED. ) ;
#63361=CARTESIAN_POINT ( 'NONE',  ( 10.81499708368651369, -2.650004840405617124, -7.499999822193714749 ) ) ;
#63365=ORIENTED_EDGE ( 'NONE', *, *, #28985, .F. ) ;
#63392=CARTESIAN_POINT ( 'NONE',  ( 11.08752429429999964, -2.871531501602999636, -6.302910744985999791 ) ) ;
#63404=CARTESIAN_POINT ( 'NONE',  ( 7.559219638201004621, -3.224407481241000628, 6.403792276147000528 ) ) ;
#63407=CARTESIAN_POINT ( 'NONE',  ( 11.09999999999999964, -5.767038119064999968, 5.145156729235000448 ) ) ;
#63410=CARTESIAN_POINT ( 'NONE',  ( 11.14698053895999941, -5.129799765052999838, 5.886044098803999702 ) ) ;
#63426=CARTESIAN_POINT ( 'NONE',  ( 7.325000000000000178, -4.000000000000000000, 9.239711431703000244 ) ) ;
#63433=LINE ( 'NONE', #847, #56365 ) ;
#63441=CARTESIAN_POINT ( 'NONE',  ( 6.960910042590000124, -9.225299970787000703, 5.198333362044999184 ) ) ;
#63442=CARTESIAN_POINT ( 'NONE',  ( 7.711433059622000208, -5.797088532631000213, 8.340479314546998424 ) ) ;
#63449=CARTESIAN_POINT ( 'NONE',  ( 8.154573290672269437, -3.060691178947356761, 6.318599490783953776 ) ) ;
#63451=CARTESIAN_POINT ( 'NONE',  ( 9.228135700785001561, -2.875364528161000077, 8.669943154892999715 ) ) ;
#63463=DIRECTION ( 'NONE',  ( 1.000000000000000000, 0.000000000000000000, 3.552713678810000077E-14 ) ) ;
#63465=CARTESIAN_POINT ( 'NONE',  ( 7.874998340266000874, -5.143395304206999974, 6.784086671025002069 ) ) ;
#63466=VERTEX_POINT ( 'NONE', #30633 ) ;
#63471=CARTESIAN_POINT ( 'NONE',  ( 10.36409408021999923, -4.600000090830000943, -4.954046131267999087 ) ) ;
#63476=CARTESIAN_POINT ( 'NONE',  ( 9.375307864587574258, -5.578557532607083758, -8.254778991542760735 ) ) ;
#63484=CARTESIAN_POINT ( 'NONE',  ( 7.769581853207999877, -2.431397064767999439, 7.958394431095000776 ) ) ;
#63488=B_SPLINE_CURVE_WITH_KNOTS ( 'NONE', 3,
 ( #4665, #15169, #42770, #53605 ),
 .UNSPECIFIED., .F., .F.,
 ( 4, 4 ),
 ( 0.000000000000000000, 1.000000000000000000 ),
 .UNSPECIFIED. ) ;
#63489=CARTESIAN_POINT ( 'NONE',  ( 10.47253786429000044, -2.899999999999999911, -6.571291218949999902 ) ) ;
#63496=CARTESIAN_POINT ( 'NONE',  ( 9.475897313459000770, -4.122021308488999836, 9.013573548576999883 ) ) ;
#63518=B_SPLINE_CURVE_WITH_KNOTS ( 'NONE', 3,
 ( #39573, #33296, #54612, #60897 ),
 .UNSPECIFIED., .F., .F.,
 ( 4, 4 ),
 ( 0.000000000000000000, 1.000000000000000000 ),
 .UNSPECIFIED. ) ;
#63520=CARTESIAN_POINT ( 'NONE',  ( 8.127481833579825121, -5.069078398454679224, 6.127575109768734762 ) ) ;
#63522=ORIENTED_EDGE ( 'NONE', *, *, #21002, .T. ) ;
#63529=FACE_OUTER_BOUND ( 'NONE', #66293, .T. ) ;
#63531=CARTESIAN_POINT ( 'NONE',  ( 7.773264358664000007, -2.859518314699000197, 6.768377407145999669 ) ) ;
#63532=CARTESIAN_POINT ( 'NONE',  ( 9.764473719840861321, -3.575759230362629104, -8.840579835172658107 ) ) ;
#63536=CARTESIAN_POINT ( 'NONE',  ( 8.751262507007865565, -5.414309366961505887, 8.580389789711265536 ) ) ;
#63543=CARTESIAN_POINT ( 'NONE',  ( 9.316120559621998254, -3.677416446733000388, 9.250734868033999803 ) ) ;
#63567=CARTESIAN_POINT ( 'NONE',  ( 10.32322131289000033, -4.654255525074000310, -4.621083567265000802 ) ) ;
#63598=CARTESIAN_POINT ( 'NONE',  ( 7.358058059621999547, -4.561648098548999997, 6.153050355516999304 ) ) ;
#63607=CARTESIAN_POINT ( 'NONE',  ( 7.467982099739825408, -2.305963387369412754, 7.104575083399867097 ) ) ;
#63625=DIRECTION ( 'NONE',  ( -1.000000000000000000, 0.000000000000000000, 0.000000000000000000 ) ) ;
#63633=CARTESIAN_POINT ( 'NONE',  ( 9.260912867475999732, -4.901383038209000453, 9.090314591495999963 ) ) ;
#63653=CARTESIAN_POINT ( 'NONE',  ( 9.571967469951999874, -4.084684048989999816, 8.946621592834999248 ) ) ;
#63671=CARTESIAN_POINT ( 'NONE',  ( 10.75110221171000013, -2.822135527917999820, 6.655890318096999714 ) ) ;
#63684=DIRECTION ( 'NONE',  ( 0.8660254037844289376, 0.000000000000000000, -0.5000000000000169864 ) ) ;
#63685=CARTESIAN_POINT ( 'NONE',  ( 11.09999999999999964, -4.000000000000000000, 7.500000000000000000 ) ) ;
#63690=CARTESIAN_POINT ( 'NONE',  ( 10.87221764200999985, -2.934320605648999880, -5.123881828670999283 ) ) ;
#63691=CARTESIAN_POINT ( 'NONE',  ( 10.56984555961999916, -2.152868447761999704, -7.425101130468999777 ) ) ;
#63711=CARTESIAN_POINT ( 'NONE',  ( 9.383148997457999130, -5.167567567567999731, 6.822293592207000934 ) ) ;
#63715=ORIENTED_EDGE ( 'NONE', *, *, #50623, .T. ) ;
#63717=ORIENTED_EDGE ( 'NONE', *, *, #30253, .T. ) ;
#63731=VECTOR ( 'NONE', #18001, 1000.000000000000114 ) ;
#63734=CARTESIAN_POINT ( 'NONE',  ( 10.30297040315999979, -4.081263557776000361, -9.025012210052000938 ) ) ;
#63737=ORIENTED_EDGE ( 'NONE', *, *, #60051, .T. ) ;
#63751=CARTESIAN_POINT ( 'NONE',  ( 8.200208800211990834, -2.889590298673998081, 6.692105494707000446 ) ) ;
#63754=CARTESIAN_POINT ( 'NONE',  ( 9.843726350706999639, -4.115123626494000320, 9.466607949400000166 ) ) ;
#63756=CARTESIAN_POINT ( 'NONE',  ( 10.72422653164066730, -2.899999999999999911, -6.304440313833583609 ) ) ;
#63757=EDGE_CURVE ( 'NONE', #17154, #15110, #5618, .T. ) ;
#63759=DIRECTION ( 'NONE',  ( 0.000000000000000000, -0.2461538461537955413, -0.9692307692307819966 ) ) ;
#63766=VERTEX_POINT ( 'NONE', #23578 ) ;
#63772=EDGE_LOOP ( 'NONE', ( #55835, #56228, #18584, #50315, #69177, #19847, #55881, #40366, #57173, #24448 ) ) ;
#63781=CARTESIAN_POINT ( 'NONE',  ( 11.05935368890999904, -2.480241580537000168, 6.610077204591000566 ) ) ;
#63786=CARTESIAN_POINT ( 'NONE',  ( 8.829019353210000531, -5.290204991635000020, 8.768102264518001121 ) ) ;
#63791=CIRCLE ( 'NONE', #39253, 0.5000000000000000000 ) ;
#63796=CARTESIAN_POINT ( 'NONE',  ( 9.476374593785998002, -5.098398394707999159, 6.305533045879999854 ) ) ;
#63810=ORIENTED_EDGE ( 'NONE', *, *, #4070, .F. ) ;
#63815=CARTESIAN_POINT ( 'NONE',  ( 10.98768472639999949, -0.3876847264043000174, -4.945212061661000469 ) ) ;
#63827=CARTESIAN_POINT ( 'NONE',  ( 8.437855646795000553, -2.606998386752999775, 6.345764833140000505 ) ) ;
#63831=AXIS2_PLACEMENT_3D ( 'NONE', #52527, #36449, #35768 ) ;
#63839=CARTESIAN_POINT ( 'NONE',  ( 9.278331853207999913, -5.791549888895000109, 7.752110689268000954 ) ) ;
#63841=FACE_OUTER_BOUND ( 'NONE', #40959, .T. ) ;
#63849=EDGE_LOOP ( 'NONE', ( #63169, #44126, #44057, #45159 ) ) ;
#63853=FACE_OUTER_BOUND ( 'NONE', #4209, .T. ) ;
#63858=CARTESIAN_POINT ( 'NONE',  ( 8.326548857933062209, -3.968851420165860233, 9.244526958411647399 ) ) ;
#63860=EDGE_LOOP ( 'NONE', ( #67605, #35528, #41115, #54133 ) ) ;
#63867=CARTESIAN_POINT ( 'NONE',  ( 7.890669427268998781, -4.660296165433000404, 6.322498843348999920 ) ) ;
#63869=CARTESIAN_POINT ( 'NONE',  ( 9.534310001152000780, -5.383415012847999392, -8.183490493635000362 ) ) ;
#63880=CARTESIAN_POINT ( 'NONE',  ( 8.930995559624999913, -2.019079883662000086, 7.390983468784999566 ) ) ;
#63881=DIRECTION ( 'NONE',  ( 1.000000000000000000, 0.000000000000000000, 0.000000000000000000 ) ) ;
#63885=FACE_OUTER_BOUND ( 'NONE', #41781, .T. ) ;
#63886=DIRECTION ( 'NONE',  ( 1.000000000000000000, 0.000000000000000000, 0.000000000000000000 ) ) ;
#63891=ORIENTED_EDGE ( 'NONE', *, *, #58437, .F. ) ;
#63892=CARTESIAN_POINT ( 'NONE',  ( 11.12483852207999924, -5.434422895407000631, -5.164705231992000378 ) ) ;
#63894=AXIS2_PLACEMENT_3D ( 'NONE', #9703, #52358, #4451 ) ;
#63924=CARTESIAN_POINT ( 'NONE',  ( 10.91620964606000044, -2.818413279081999789, -6.814156272943999504 ) ) ;
#63928=AXIS2_PLACEMENT_3D ( 'NONE', #37621, #65223, #59290 ) ;
#63939=CARTESIAN_POINT ( 'NONE',  ( 9.532671748231999587, -4.663050389319001177, 8.669823109968998409 ) ) ;
#63940=CARTESIAN_POINT ( 'NONE',  ( 8.128308059623998716, -3.117370956513999758, 8.662188901935000018 ) ) ;
#63944=CARTESIAN_POINT ( 'NONE',  ( 10.52384314678999999, -5.441919393629000012, -7.989634081859001036 ) ) ;
#63945=CARTESIAN_POINT ( 'NONE',  ( 7.754788148867381992, -5.333023120641254167, 8.617227868399091051 ) ) ;
#63966=DIRECTION ( 'NONE',  ( 0.000000000000000000, -1.000000000000000000, 0.000000000000000000 ) ) ;
#63969=CARTESIAN_POINT ( 'NONE',  ( 10.98286725694000054, -3.998514182530999772, 9.091066422484001208 ) ) ;
#63982=EDGE_CURVE ( 'NONE', #8257, #38701, #3157, .T. ) ;
#64009=ORIENTED_EDGE ( 'NONE', *, *, #34943, .F. ) ;
#64017=ORIENTED_EDGE ( 'NONE', *, *, #32078, .T. ) ;
#64025=CARTESIAN_POINT ( 'NONE',  ( 11.09999999999999964, -5.340540540541000247, -6.721892642903999793 ) ) ;
#64027=CARTESIAN_POINT ( 'NONE',  ( 10.33453064679000200, -3.295701412239999684, -6.149875347297999895 ) ) ;
#64028=EDGE_CURVE ( 'NONE', #32816, #58368, #66401, .T. ) ;
#64032=CARTESIAN_POINT ( 'NONE',  ( -15.86200481174999943, -2.399999999999999911, 6.571291218949999902 ) ) ;
#64038=CYLINDRICAL_SURFACE ( 'NONE', #67489, 1.350000000000000089 ) ;
#64060=B_SPLINE_CURVE_WITH_KNOTS ( 'NONE', 3,
 ( #6839, #37964, #915, #33075 ),
 .UNSPECIFIED., .F., .F.,
 ( 4, 4 ),
 ( 0.000000000000000000, 1.000000000000000000 ),
 .UNSPECIFIED. ) ;
#64065=VERTEX_POINT ( 'NONE', #23760 ) ;
#64074=CARTESIAN_POINT ( 'NONE',  ( 10.57793869653000129, -4.393380534095000733, -6.024358525186999991 ) ) ;
#64082=CARTESIAN_POINT ( 'NONE',  ( 10.36503728015203230, -2.650011783303574564, -7.500002219258004921 ) ) ;
#64087=CONICAL_SURFACE ( 'NONE', #4961, 1.349999998858999906, 0.7853981633972997312 ) ;
#64093=CARTESIAN_POINT ( 'NONE',  ( 7.475100008705002352, -3.230432416208002699, 6.447622763416998914 ) ) ;
#64095=DIRECTION ( 'NONE',  ( -1.000000000000000000, 0.000000000000000000, 0.000000000000000000 ) ) ;
#64096=CARTESIAN_POINT ( 'NONE',  ( 9.380781717619999682, -2.204246399534000034, 7.545378188773000261 ) ) ;
#64113=CARTESIAN_POINT ( 'NONE',  ( 7.714733813452927969, -2.650598945404480045, 7.676825647508595196 ) ) ;
#64117=CARTESIAN_POINT ( 'NONE',  ( 10.86180282789683460, -2.874603711584073462, -6.749639981064807337 ) ) ;
#64120=ORIENTED_EDGE ( 'NONE', *, *, #67550, .T. ) ;
#64122=CARTESIAN_POINT ( 'NONE',  ( 9.576494682405000347, -4.593972507100000158, 5.662052676321000177 ) ) ;
#64123=DIRECTION ( 'NONE',  ( -0.8660254018730039194, -3.203742570879014573E-12, 0.5000000033107019348 ) ) ;
#64126=CARTESIAN_POINT ( 'NONE',  ( 8.058769353207999586, -2.432121990576000314, 6.597519606637999523 ) ) ;
#64132=CARTESIAN_POINT ( 'NONE',  ( 11.09999999999999964, -5.350000000000000533, 7.500000000000000000 ) ) ;
#64133=CARTESIAN_POINT ( 'NONE',  ( 8.180537356029997653, -3.349941516901878025, 6.152975253528285116 ) ) ;
#64135=CARTESIAN_POINT ( 'NONE',  ( 9.380781717619999682, -2.204246399534000034, 7.545378188773000261 ) ) ;
#64137=CARTESIAN_POINT ( 'NONE',  ( 5.500000000000000000, -1.300000000000000044, -10.46294468575700165 ) ) ;
#64138=ORIENTED_EDGE ( 'NONE', *, *, #10045, .F. ) ;
#64141=CARTESIAN_POINT ( 'NONE',  ( 10.34939194037999854, -2.653148377029999949, -7.312413909354000374 ) ) ;
#64143=DIRECTION ( 'NONE',  ( -3.710543846949000018E-09, 3.726597655970000124E-11, -1.000000000000000000 ) ) ;
#64165=CARTESIAN_POINT ( 'NONE',  ( 9.366922563375464250, -5.649238375891439290, -8.083220911872984971 ) ) ;
#64170=CARTESIAN_POINT ( 'NONE',  ( 9.272293146792000229, -3.705847642455000202, 9.096432253453999195 ) ) ;
#64182=CARTESIAN_POINT ( 'NONE',  ( 7.416894353206999746, -3.448181789123000218, 9.222458996124998976 ) ) ;
#64183=CARTESIAN_POINT ( 'NONE',  ( 9.216851002545999094, -2.832432432432000269, 6.822293592207000934 ) ) ;
#64184=DIRECTION ( 'NONE',  ( 1.000000000000000000, 0.000000000000000000, 0.000000000000000000 ) ) ;
#64187=CARTESIAN_POINT ( 'NONE',  ( 11.01356641589999974, -2.786433584103999994, 6.253463831328000211 ) ) ;
#64200=CARTESIAN_POINT ( 'NONE',  ( 8.551242329018723609, -3.500793602214988365, 5.833163798001932854 ) ) ;
#64211=ORIENTED_EDGE ( 'NONE', *, *, #47919, .T. ) ;
#64212=CARTESIAN_POINT ( 'NONE',  ( 10.64418092495376378, -2.624263734258304837, -6.377679599447885650 ) ) ;
#64219=VERTEX_POINT ( 'NONE', #36307 ) ;
#64223=ORIENTED_EDGE ( 'NONE', *, *, #12087, .F. ) ;
#64231=CARTESIAN_POINT ( 'NONE',  ( 7.100000000000000533, -4.000000000000000000, -7.500000000000000000 ) ) ;
#64242=CARTESIAN_POINT ( 'NONE',  ( 10.76232069631999977, -3.259150589222000072, -8.644998763029001054 ) ) ;
#64263=LINE ( 'NONE', #16715, #24642 ) ;
#64267=EDGE_LOOP ( 'NONE', ( #37604, #50009, #40815, #9358 ) ) ;
#64273=CARTESIAN_POINT ( 'NONE',  ( 10.84289849785072590, -2.713620053740499305, -7.026897974086598886 ) ) ;
#64278=CARTESIAN_POINT ( 'NONE',  ( 9.479212726990999371, -4.071727350623000063, 9.089303488377000306 ) ) ;
#64279=CARTESIAN_POINT ( 'NONE',  ( 8.860769353209001054, -2.935738482289000029, 6.259841087764999479 ) ) ;
#64283=CARTESIAN_POINT ( 'NONE',  ( 10.58470685321000104, -2.966812129551000154, -8.831977776575000050 ) ) ;
#64284=CARTESIAN_POINT ( 'NONE',  ( 7.829206492768003400, -3.883838858848270181, 9.258058093495069585 ) ) ;
#64285=CARTESIAN_POINT ( 'NONE',  ( 10.83668192271000130, -4.288535286065000562, 9.448729895547000268 ) ) ;
#64295=EDGE_CURVE ( 'NONE', #24787, #49573, #16012, .T. ) ;
#64301=CARTESIAN_POINT ( 'NONE',  ( 8.239941940377999430, -2.735207418315000361, 6.771977475428999860 ) ) ;
#64309=CARTESIAN_POINT ( 'NONE',  ( 10.66951732929000052, -4.592671928130000580, 5.841406818427000047 ) ) ;
#64326=CARTESIAN_POINT ( 'NONE',  ( 9.525000000000000355, -4.417172942406000224, 8.783926296998000538 ) ) ;
#64327=B_SPLINE_CURVE_WITH_KNOTS ( 'NONE', 3,
 ( #48492, #32080, #16322, #10389, #597, #16667 ),
 .UNSPECIFIED., .F., .F.,
 ( 4, 2, 4 ),
 ( 0.000000000000000000, 0.5000000000000000000, 1.000000000000000000 ),
 .UNSPECIFIED. ) ;
#64330=AXIS2_PLACEMENT_3D ( 'NONE', #13336, #34660, #55973 ) ;
#64344=CARTESIAN_POINT ( 'NONE',  ( 10.34365768245000083, -4.000000000000000000, -4.787564842381000219 ) ) ;
#64355=ORIENTED_EDGE ( 'NONE', *, *, #52874, .T. ) ;
#64359=CARTESIAN_POINT ( 'NONE',  ( 27.64127793187000037, -5.599999999999999645, 6.571291218949999902 ) ) ;
#64362=CARTESIAN_POINT ( 'NONE',  ( 10.33253786428999987, -2.899999999999999911, 6.571291218949999902 ) ) ;
#64366=CARTESIAN_POINT ( 'NONE',  ( 10.05463185321000097, -3.531218470783999752, -9.119231780812000920 ) ) ;
#64378=AXIS2_PLACEMENT_3D ( 'NONE', #5882, #59718, #64609 ) ;
#64389=CARTESIAN_POINT ( 'NONE',  ( 9.662447522843001124, -4.824180051339999942, -8.517611033492999084 ) ) ;
#64391=ORIENTED_EDGE ( 'NONE', *, *, #52184, .T. ) ;
#64394=EDGE_CURVE ( 'NONE', #65751, #17545, #1417, .T. ) ;
#64402=CARTESIAN_POINT ( 'NONE',  ( 9.848253563160000112, -4.436921580929999998, 6.148020168057000134 ) ) ;
#64414=CARTESIAN_POINT ( 'NONE',  ( 9.856713838269000050, -4.814118338972999567, -8.929571672388000536 ) ) ;
#64419=AXIS2_PLACEMENT_3D ( 'NONE', #57547, #48440, #20492 ) ;
#64431=CARTESIAN_POINT ( 'NONE',  ( 8.062814847549001129, -3.480055400096998319, 6.228346641557002350 ) ) ;
#64435=CARTESIAN_POINT ( 'NONE',  ( 9.629020610622001541, -5.794331084664000819, 7.414872097535999629 ) ) ;
#64446=CYLINDRICAL_SURFACE ( 'NONE', #29006, 0.5000000000000002220 ) ;
#64461=CARTESIAN_POINT ( 'NONE',  ( 10.80169466977000070, -3.998196228428999355, 9.431543037543999475 ) ) ;
#64464=CARTESIAN_POINT ( 'NONE',  ( 10.98768538770000092, -2.700669876604000041, 4.945210823433001224 ) ) ;
#64467=ORIENTED_EDGE ( 'NONE', *, *, #61926, .F. ) ;
#64473=CARTESIAN_POINT ( 'NONE',  ( 10.34521071928999980, -2.724119865955000108, 6.497322598008000050 ) ) ;
#64479=CARTESIAN_POINT ( 'NONE',  ( 11.06877944038000017, -5.318813217120000658, -7.168443364726000411 ) ) ;
#64487=CARTESIAN_POINT ( 'NONE',  ( 5.600000001140999828, 0.000000000000000000, 0.000000000000000000 ) ) ;
#64492=CARTESIAN_POINT ( 'NONE',  ( 9.323387100380815085, -4.033245596547300416, 9.239790378170226859 ) ) ;
#64496=LINE ( 'NONE', #48095, #49715 ) ;
#64506=CARTESIAN_POINT ( 'NONE',  ( 9.696086916451999826, -2.554404004330999900, 7.600685922079000179 ) ) ;
#64509=CARTESIAN_POINT ( 'NONE',  ( 8.245293146793999384, -4.282999948634999221, 9.286791354293999490 ) ) ;
#64514=AXIS2_PLACEMENT_3D ( 'NONE', #8754, #39889, #17873 ) ;
#64518=CARTESIAN_POINT ( 'NONE',  ( 8.348430368788083200, -2.904639935713019039, 6.526593578780762073 ) ) ;
#64519=VECTOR ( 'NONE', #23695, 1000.000000000000114 ) ;
#64522=CARTESIAN_POINT ( 'NONE',  ( 9.497293146791999874, -3.734278838175999482, 8.942129638874000364 ) ) ;
#64543=CARTESIAN_POINT ( 'NONE',  ( 8.499790797351490568, -2.599905373318510460, 6.452158339067893600 ) ) ;
#64550=ORIENTED_EDGE ( 'NONE', *, *, #659, .T. ) ;
#64556=FILL_AREA_STYLE_COLOUR ( '', #15944 ) ;
#64558=CARTESIAN_POINT ( 'NONE',  ( 8.902961428628096030, -2.546297866003439214, 8.472527682318533593 ) ) ;
#64563=EDGE_CURVE ( 'NONE', #56639, #8998, #50586, .T. ) ;
#64567=CARTESIAN_POINT ( 'NONE',  ( 9.112942518363999156, -5.100000000000000533, 6.192000867487999827 ) ) ;
#64568=ORIENTED_EDGE ( 'NONE', *, *, #25570, .T. ) ;
#64573=CYLINDRICAL_SURFACE ( 'NONE', #32671, 1.350000000000000089 ) ;
#64576=VECTOR ( 'NONE', #52668, 1000.000000000000000 ) ;
#64582=VERTEX_POINT ( 'NONE', #5009 ) ;
#64590=AXIS2_PLACEMENT_3D ( 'NONE', #24528, #35031, #14389 ) ;
#64609=DIRECTION ( 'NONE',  ( 0.000000000000000000, 0.000000000000000000, -1.000000000000000000 ) ) ;
#64625=CARTESIAN_POINT ( 'NONE',  ( 9.681180837610000367, -2.612237299844000216, 7.804680206899999639 ) ) ;
#64626=CARTESIAN_POINT ( 'NONE',  ( 9.272293146792000229, -3.705847642455000202, 9.096432253453999195 ) ) ;
#64632=CARTESIAN_POINT ( 'NONE',  ( 10.35753185321000025, -5.367809014988999650, -6.514738374536999999 ) ) ;
#64633=CARTESIAN_POINT ( 'NONE',  ( 7.769665546845473614, -5.098373949222779977, 8.848957063549683255 ) ) ;
#64635=DIRECTION ( 'NONE',  ( 0.000000000000000000, 1.000000000000000000, 0.000000000000000000 ) ) ;
#64636=VERTEX_POINT ( 'NONE', #60571 ) ;
#64649=CARTESIAN_POINT ( 'NONE',  ( 10.39297979612879530, -2.713506317167766468, -7.026950959993343737 ) ) ;
#64651=CARTESIAN_POINT ( 'NONE',  ( 9.074379440379999551, -3.981661727120999750, 8.959239802162999311 ) ) ;
#64657=CARTESIAN_POINT ( 'NONE',  ( 10.66052890781999984, -2.899999999999999911, -6.152188490330000370 ) ) ;
#64666=ORIENTED_EDGE ( 'NONE', *, *, #3165, .T. ) ;
#64676=CARTESIAN_POINT ( 'NONE',  ( 10.96888392554999925, -5.599999999999999645, 6.571291218949999902 ) ) ;
#64681=CARTESIAN_POINT ( 'NONE',  ( 9.509907746701999898, -5.077451867123000007, 8.469011304701000498 ) ) ;
#64684=ADVANCED_FACE ( 'NONE', ( #13033 ), #17930, .T. ) ;
#64689=CARTESIAN_POINT ( 'NONE',  ( 5.700000000000000178, 0.8000000000000000444, -3.149999999999999911 ) ) ;
#64697=ORIENTED_EDGE ( 'NONE', *, *, #47274, .F. ) ;
#64705=VERTEX_POINT ( 'NONE', #34360 ) ;
#64707=CARTESIAN_POINT ( 'NONE',  ( 11.09999999999999964, -2.700688486617000006, 5.124965750789000296 ) ) ;
#64715=CARTESIAN_POINT ( 'NONE',  ( 7.000000000000000000, -0.2897247358851999799, -3.000000000000000000 ) ) ;
#64716=CARTESIAN_POINT ( 'NONE',  ( 10.28180685320999999, -3.991526694881000203, -5.814304247846999729 ) ) ;
#64721=ORIENTED_EDGE ( 'NONE', *, *, #62693, .F. ) ;
#64732=CARTESIAN_POINT ( 'NONE',  ( 8.642358819840239903, -3.294576102360963876, 8.704493534904289120 ) ) ;
#64737=CARTESIAN_POINT ( 'NONE',  ( 10.07930721860999945, -2.718124813223000036, -6.397797539448999871 ) ) ;
#64747=CARTESIAN_POINT ( 'NONE',  ( 10.78622389186427277, -2.904384452724245058, 5.097246023308017016 ) ) ;
#64748=DIRECTION ( 'NONE',  ( -0.8231338744408063235, -0.5678473604306591982, 0.000000000000000000 ) ) ;
#64755=CARTESIAN_POINT ( 'NONE',  ( 10.60454482602940018, -3.072763806055099245, 8.633921737781435013 ) ) ;
#64760=CARTESIAN_POINT ( 'NONE',  ( 10.83767365324000131, -5.758089526411000136, -6.911472812823999945 ) ) ;
#64766=DIRECTION ( 'NONE',  ( 1.307574445097999928E-09, 5.454265898252000151E-12, -1.000000000000000000 ) ) ;
#64767=CARTESIAN_POINT ( 'NONE',  ( 8.644633100483858357, -3.089364588649414767, -6.503246041658669263 ) ) ;
#64775=CARTESIAN_POINT ( 'NONE',  ( 5.500000000000000000, 0.4800000000000000377, 1.889999999999999902 ) ) ;
#64780=CARTESIAN_POINT ( 'NONE',  ( 11.08492081570999943, -3.668392767032000013, 5.558160538745999801 ) ) ;
#64783=CARTESIAN_POINT ( 'NONE',  ( 9.571967469951999874, -4.084684048989999816, 8.946621592834999248 ) ) ;
#64799=CARTESIAN_POINT ( 'NONE',  ( 11.09999999999999964, -5.299999999999999822, 5.160242713806000303 ) ) ;
#64807=CARTESIAN_POINT ( 'NONE',  ( 11.09999999999999964, -6.593648102827000201, 5.598803487171999826 ) ) ;
#64819=CARTESIAN_POINT ( 'NONE',  ( 10.49646369190723405, -5.100000000000000533, -6.665341197409489382 ) ) ;
#64837=CARTESIAN_POINT ( 'NONE',  ( 9.327378398803991999, -3.946271215605382743, 9.238828740155991426 ) ) ;
#64844=CARTESIAN_POINT ( 'NONE',  ( 9.595487457706001422, -3.928425191288000384, 5.531324308465000783 ) ) ;
#64848=ORIENTED_EDGE ( 'NONE', *, *, #30926, .F. ) ;
#64854=CARTESIAN_POINT ( 'NONE',  ( 9.944325809452999820, -5.443013936195000291, 7.367349259341000156 ) ) ;
#64856=CARTESIAN_POINT ( 'NONE',  ( 8.577620559625000141, -3.981661727120999750, 8.959239802162999311 ) ) ;
#64865=DIRECTION ( 'NONE',  ( 0.000000000000000000, -0.7071067811865474617, -0.7071067811865474617 ) ) ;
#64882=PLANE ( 'NONE',  #2014 ) ;
#64887=CARTESIAN_POINT ( 'NONE',  ( 8.381640933329739696, -2.862614012586783385, 8.816379852580610077 ) ) ;
#64890=EDGE_LOOP ( 'NONE', ( #9498, #11621, #63365, #28036, #17899 ) ) ;
#64899=CARTESIAN_POINT ( 'NONE',  ( 10.30195995176331714, -5.579776588524842929, -6.689560773767187385 ) ) ;
#64909=CARTESIAN_POINT ( 'NONE',  ( 11.09999999999999964, -0.5000000000000000000, 9.662944685757000940 ) ) ;
#64913=DIRECTION ( 'NONE',  ( 1.000000000000000000, 0.000000000000000000, 0.000000000000000000 ) ) ;
#64926=CARTESIAN_POINT ( 'NONE',  ( 9.662447522843001124, -4.824180051339999942, -8.517611033492999084 ) ) ;
#64954=CARTESIAN_POINT ( 'NONE',  ( 11.02038275177999971, -5.599999999999999645, -6.571291218949999902 ) ) ;
#64955=EDGE_CURVE ( 'NONE', #21511, #17545, #33293, .T. ) ;
#64964=CARTESIAN_POINT ( 'NONE',  ( 10.23808992278000041, -2.752437370156000540, 6.820045513931999537 ) ) ;
#64969=CARTESIAN_POINT ( 'NONE',  ( 10.82674314678999927, -3.167157901876000103, -6.225148200207000215 ) ) ;
#64970=CARTESIAN_POINT ( 'NONE',  ( 7.662320246279550773, -5.560547198184215389, 6.711813256769637803 ) ) ;
#64971=CARTESIAN_POINT ( 'NONE',  ( 9.566960887370999700, -5.215923019114000247, 6.177729435798999802 ) ) ;
#64972=CARTESIAN_POINT ( 'NONE',  ( 9.991937366751301397, -4.976291841660785309, 8.591989380854540670 ) ) ;
#64974=AXIS2_PLACEMENT_3D ( 'NONE', #61659, #7141, #51508 ) ;
#64993=CARTESIAN_POINT ( 'NONE',  ( 10.83488305961999920, -5.800181157098999840, -7.920538492179999501 ) ) ;
#65011=CARTESIAN_POINT ( 'NONE',  ( 6.953052440528999512, -9.233022020364000326, -5.200634764108000851 ) ) ;
#65020=CARTESIAN_POINT ( 'NONE',  ( 9.385788300200999856, -4.980873770300999759, 6.433336655958999728 ) ) ;
#65045=CARTESIAN_POINT ( 'NONE',  ( 10.90000000011000125, -5.100000000110999743, 6.571291220762999430 ) ) ;
#65057=CARTESIAN_POINT ( 'NONE',  ( 10.66043185321000131, -2.315667072036000196, -7.431702410656999547 ) ) ;
#65064=CARTESIAN_POINT ( 'NONE',  ( 11.01268131116999882, -8.059163363648998768, -6.866685204375000851 ) ) ;
#65074=CARTESIAN_POINT ( 'NONE',  ( 8.579854990165863171, -4.352864158101605874, 8.850923404438391984 ) ) ;
#65079=CARTESIAN_POINT ( 'NONE',  ( 10.82564972918999935, -5.331162346451000289, -8.542142527201001201 ) ) ;
#65088=CARTESIAN_POINT ( 'NONE',  ( 10.55918725779999967, -5.125768249360000084, 4.818464946407000404 ) ) ;
#65094=CARTESIAN_POINT ( 'NONE',  ( 10.07101719722999889, -4.042170815906999337, 8.920201479886998186 ) ) ;
#65106=CARTESIAN_POINT ( 'NONE',  ( 10.39355669675000016, -4.089958462238000081, -9.188182957628999503 ) ) ;
#65108=CARTESIAN_POINT ( 'NONE',  ( 9.537027461449516963, -5.286011494985110026, -7.027146145907680719 ) ) ;
#65109=DIRECTION ( 'NONE',  ( 0.000000000000000000, 1.000000000000000000, 0.000000000000000000 ) ) ;
#65112=CARTESIAN_POINT ( 'NONE',  ( 8.627615187423813836, -2.899999999999999911, 6.423404451745915011 ) ) ;
#65119=CARTESIAN_POINT ( 'NONE',  ( 10.95824452673999971, -2.933481078303000089, 5.181932056174999524 ) ) ;
#65121=VERTEX_POINT ( 'NONE', #42344 ) ;
#65126=CARTESIAN_POINT ( 'NONE',  ( 10.09196524370999981, -3.841385669346000231, 5.536421174581999338 ) ) ;
#65129=CARTESIAN_POINT ( 'NONE',  ( 10.99433452212999818, -3.697619272994999928, 5.729306330972000261 ) ) ;
#65130=CARTESIAN_POINT ( 'NONE',  ( 10.02052890782000105, -2.899999999999999911, 6.152188490330000370 ) ) ;
#65132=VECTOR ( 'NONE', #24351, 1000.000000000000114 ) ;
#65137=VECTOR ( 'NONE', #33570, 1000.000000000000000 ) ;
#65138=DIRECTION ( 'NONE',  ( 0.000000000000000000, -0.1333333333333049375, 0.9910712498212376209 ) ) ;
#65162=EDGE_CURVE ( 'NONE', #33712, #10649, #1064, .T. ) ;
#65168=EDGE_LOOP ( 'NONE', ( #18073, #48145, #2346, #6085, #39987 ) ) ;
#65176=CARTESIAN_POINT ( 'NONE',  ( 11.37167944038000122, -2.803484087760999888, -6.967877228197000505 ) ) ;
#65177=ORIENTED_EDGE ( 'NONE', *, *, #29225, .T. ) ;
#65193=CARTESIAN_POINT ( 'NONE',  ( 10.71256247620999957, -5.951803124515000043, 7.233045248871000865 ) ) ;
#65197=VERTEX_POINT ( 'NONE', #29029 ) ;
#65204=CARTESIAN_POINT ( 'NONE',  ( 10.87522165821000009, -4.831071966430999787, 6.312786525516999703 ) ) ;
#65206=CARTESIAN_POINT ( 'NONE',  ( 10.90000000000000036, -2.778483479159999714, -6.925197956411000000 ) ) ;
#65216=CARTESIAN_POINT ( 'NONE',  ( 8.327311442791936358, -2.900678125132057694, 6.583025523232378440 ) ) ;
#65219=ORIENTED_EDGE ( 'NONE', *, *, #44598, .T. ) ;
#65220=CARTESIAN_POINT ( 'NONE',  ( 8.610058059625000482, -5.329429281359999493, 6.027400270608000099 ) ) ;
#65223=DIRECTION ( 'NONE',  ( 1.000000000000000000, 0.000000000000000000, 0.000000000000000000 ) ) ;
#65240=CARTESIAN_POINT ( 'NONE',  ( 8.448578618970964627, -2.260522387638269848, 7.526897675015515432 ) ) ;
#65242=CONICAL_SURFACE ( 'NONE', #18403, 0.8999999994071996579, 0.7853981633972997312 ) ;
#65268=CARTESIAN_POINT ( 'NONE',  ( 11.09999999999999964, -5.350000000000000533, -7.500000000000000000 ) ) ;
#65279=CONICAL_SURFACE ( 'NONE', #68617, 2.049999999589000588, 0.7853981633972997312 ) ;
#65283=CARTESIAN_POINT ( 'NONE',  ( 10.38153277269999997, -2.772136814285999673, -8.408084799892998618 ) ) ;
#65287=DIRECTION ( 'NONE',  ( -0.7071067811864999442, 0.09428090792503998618, -0.7007932008808999136 ) ) ;
#65301=ADVANCED_FACE ( 'NONE', ( #61515 ), #40198, .F. ) ;
#65303=CARTESIAN_POINT ( 'NONE',  ( 7.795980646793000624, -3.164807285701999984, 9.104732190648000767 ) ) ;
#65304=CARTESIAN_POINT ( 'NONE',  ( 9.399722005181999407, -5.700621988293000264, -7.339579610785999186 ) ) ;
#65318=CARTESIAN_POINT ( 'NONE',  ( 9.848253563160000112, -4.436921580929999998, 6.148020168057000134 ) ) ;
#65320=ORIENTED_EDGE ( 'NONE', *, *, #39476, .F. ) ;
#65324=CARTESIAN_POINT ( 'NONE',  ( 10.63743064679000128, -3.721475434679999861, -8.997096235511000017 ) ) ;
#65325=CARTESIAN_POINT ( 'NONE',  ( 7.804884823657623372, -4.430740684302771903, 9.185820566326194481 ) ) ;
#65326=CARTESIAN_POINT ( 'NONE',  ( 11.02286109245999945, -2.398753588646000079, 6.352476128646999065 ) ) ;
#65351=CARTESIAN_POINT ( 'NONE',  ( 11.17788601987000163, -2.412142864687000010, -7.075602314719000141 ) ) ;
#65353=LINE ( 'NONE', #38797, #60572 ) ;
#65392=AXIS2_PLACEMENT_3D ( 'NONE', #56737, #51143, #29141 ) ;
#65404=ORIENTED_EDGE ( 'NONE', *, *, #41655, .T. ) ;
#65416=CARTESIAN_POINT ( 'NONE',  ( 10.78888064679000003, -2.675723359162999859, -6.748225798259000818 ) ) ;
#65427=ORIENTED_EDGE ( 'NONE', *, *, #50757, .F. ) ;
#65431=VECTOR ( 'NONE', #54237, 1000.000000000000000 ) ;
#65436=CARTESIAN_POINT ( 'NONE',  ( 11.03407957707000087, -2.992853177526999975, -9.056567163506000995 ) ) ;
#65439=CARTESIAN_POINT ( 'NONE',  ( 10.57286587299508440, -3.010279057788120660, -5.022110908762327242 ) ) ;
#65440=EDGE_LOOP ( 'NONE', ( #67388, #54776, #68761, #48173 ) ) ;
#65446=CARTESIAN_POINT ( 'NONE',  ( 10.95390526108000095, -5.337639433354000040, 4.888929981400999658 ) ) ;
#65448=CARTESIAN_POINT ( 'NONE',  ( 10.53855965315437082, -2.999267221421852980, 5.023112174284990239 ) ) ;
#65451=CARTESIAN_POINT ( 'NONE',  ( 10.05691733561000056, -2.453480799114999833, 6.657106310117000270 ) ) ;
#65461=CARTESIAN_POINT ( 'NONE',  ( 10.91623602276999883, -5.459825388708999583, -8.642870457474998602 ) ) ;
#65466=CARTESIAN_POINT ( 'NONE',  ( 8.548990840217488341, -3.103435619188711136, 6.042760497454945146 ) ) ;
#65477=CARTESIAN_POINT ( 'NONE',  ( 7.411085905969002852, -3.233236485764999113, 6.481842843012996624 ) ) ;
#65481=CARTESIAN_POINT ( 'NONE',  ( 10.22109127278999807, -2.983266195621000261, 8.764707262515999631 ) ) ;
#65482=CARTESIAN_POINT ( 'NONE',  ( 10.00371413511149932, -2.641056634684001203, 6.398884489502225215 ) ) ;
#65496=ORIENTED_EDGE ( 'NONE', *, *, #29374, .T. ) ;
#65497=CYLINDRICAL_SURFACE ( 'NONE', #7609, 2.149999999999999911 ) ;
#65504=DIRECTION ( 'NONE',  ( 0.8660254037844968833, -2.665883466949989686E-12, -0.4999999999998989142 ) ) ;
#65506=EDGE_CURVE ( 'NONE', #52017, #34080, #28948, .T. ) ;
#65513=CARTESIAN_POINT ( 'NONE',  ( 11.10000000000000142, -2.495605073370282145, -8.212123196678321690 ) ) ;
#65516=CARTESIAN_POINT ( 'NONE',  ( 10.98333333333533091, -4.339018939180776080, 8.912414555067401878 ) ) ;
#65518=CARTESIAN_POINT ( 'NONE',  ( 10.96580795178999956, -4.930647899304999804, 6.170539049947000088 ) ) ;
#65524=CARTESIAN_POINT ( 'NONE',  ( 11.29595444038000096, -2.828863075736999910, -8.191124550002999882 ) ) ;
#65525=VERTEX_POINT ( 'NONE', #17044 ) ;
#65544=CARTESIAN_POINT ( 'NONE',  ( 9.533427734455999669, -2.564762519363000148, 6.150594768287000136 ) ) ;
#65554=CARTESIAN_POINT ( 'NONE',  ( 10.00638553269999953, -5.119272496996000399, 8.420388242270998802 ) ) ;
#65557=CARTESIAN_POINT ( 'NONE',  ( 5.699999999836000697, -1.433333331105999919, -10.65401593570999950 ) ) ;
#65560=CARTESIAN_POINT ( 'NONE',  ( 8.663116700034002804, -5.178392435731003829, -6.846672731545002222 ) ) ;
#65561=DIRECTION ( 'NONE',  ( 0.000000000000000000, 1.000000000000000000, 0.000000000000000000 ) ) ;
#65572=EDGE_CURVE ( 'NONE', #46074, #37636, #6559, .T. ) ;
#65574=CARTESIAN_POINT ( 'NONE',  ( 10.25036334590209464, -3.059888261081735727, -8.493457116339172330 ) ) ;
#65575=CARTESIAN_POINT ( 'NONE',  ( 7.874998340266000874, -5.143395304206999974, 6.784086671025002069 ) ) ;
#65580=ORIENTED_EDGE ( 'NONE', *, *, #68658, .T. ) ;
#65588=DIRECTION ( 'NONE',  ( 0.000000000000000000, 1.000000000000000000, 0.000000000000000000 ) ) ;
#65592=ORIENTED_EDGE ( 'NONE', *, *, #46405, .F. ) ;
#65593=CARTESIAN_POINT ( 'NONE',  ( 11.09999999999999964, -2.700230688176999738, 5.136744346970999686 ) ) ;
#65607=DIRECTION ( 'NONE',  ( 0.000000000000000000, -1.000000000000000000, 0.000000000000000000 ) ) ;
#65611=CARTESIAN_POINT ( 'NONE',  ( 10.47253786429000044, -2.899999999999999911, -6.571291218949999902 ) ) ;
#65617=CARTESIAN_POINT ( 'NONE',  ( 5.700000000000000178, 0.000000000000000000, -1.250000000000000000 ) ) ;
#65627=CARTESIAN_POINT ( 'NONE',  ( 9.898134631442999876, -2.965923230546999800, -6.610863544715000373 ) ) ;
#65636=CARTESIAN_POINT ( 'NONE',  ( 10.79212049823023278, -3.170455386494715810, -8.579526322294743323 ) ) ;
#65649=CARTESIAN_POINT ( 'NONE',  ( 8.694605646795000808, -5.290204991635000020, 8.768102264518001121 ) ) ;
#65650=CARTESIAN_POINT ( 'NONE',  ( 10.19691842572999896, -4.268950419651999617, -8.781589108989999559 ) ) ;
#65651=EDGE_CURVE ( 'NONE', #29508, #39266, #9768, .T. ) ;
#65652=EDGE_CURVE ( 'NONE', #53921, #664, #8909, .T. ) ;
#65666=CARTESIAN_POINT ( 'NONE',  ( 10.35616740164000049, -2.777283710737999733, 8.995265811011998736 ) ) ;
#65668=ORIENTED_EDGE ( 'NONE', *, *, #27877, .F. ) ;
#65672=CARTESIAN_POINT ( 'NONE',  ( 10.42511694037999881, -3.371058793856000158, -6.294333763729999198 ) ) ;
#65673=CARTESIAN_POINT ( 'NONE',  ( 7.958764476359821316, -2.272891526873158874, 7.290622470508028030 ) ) ;
#65674=CARTESIAN_POINT ( 'NONE',  ( 9.781666627457001439, -5.464740618746000145, 8.817321229216000589 ) ) ;
#65685=CIRCLE ( 'NONE', #2070, 1.000000000000000444 ) ;
#65695=ORIENTED_EDGE ( 'NONE', *, *, #659, .F. ) ;
#65698=EDGE_CURVE ( 'NONE', #57495, #23524, #15254, .T. ) ;
#65699=CARTESIAN_POINT ( 'NONE',  ( 10.87274555961999845, -5.407608219159000029, -8.698392243238998844 ) ) ;
#65702=CARTESIAN_POINT ( 'NONE',  ( 8.048510972020597620, -4.829207235971667345, 8.579008051763574727 ) ) ;
#65709=VERTEX_POINT ( 'NONE', #10687 ) ;
#65713=B_SPLINE_CURVE_WITH_KNOTS ( 'NONE', 3,
 ( #50862, #25315, #20073, #13126 ),
 .UNSPECIFIED., .F., .F.,
 ( 4, 4 ),
 ( 0.000000000000000000, 1.000000000000000000 ),
 .UNSPECIFIED. ) ;
#65724=CARTESIAN_POINT ( 'NONE',  ( 8.392489902862999784, -5.100228725471000146, 6.589622881798000265 ) ) ;
#65727=CIRCLE ( 'NONE', #35604, 1.350000000000000533 ) ;
#65731=ORIENTED_EDGE ( 'NONE', *, *, #51859, .T. ) ;
#65738=DIRECTION ( 'NONE',  ( 0.4384236320213992233, -0.6355252626312997144, -0.6355252626312997144 ) ) ;
#65749=CARTESIAN_POINT ( 'NONE',  ( 9.424850088744616272, -5.349972419855331118, 7.500009359253513530 ) ) ;
#65751=VERTEX_POINT ( 'NONE', #15934 ) ;
#65763=CARTESIAN_POINT ( 'NONE',  ( 8.745593092018999926, -5.100000000000000533, 6.404090157675000228 ) ) ;
#65764=CARTESIAN_POINT ( 'NONE',  ( 11.29595444038000096, -2.828863075736999910, -8.191124550002999882 ) ) ;
#65783=CARTESIAN_POINT ( 'NONE',  ( 10.23643195768000069, -5.517145045299000294, -6.754127937316000363 ) ) ;
#65790=CARTESIAN_POINT ( 'NONE',  ( 10.73278136149000161, -5.209917005081999619, 4.894959764772000455 ) ) ;
#65791=CARTESIAN_POINT ( 'NONE',  ( 10.74207053302677828, -3.170338597610990128, -8.579608023176293230 ) ) ;
#65795=CARTESIAN_POINT ( 'NONE',  ( 9.590594544025000445, -2.445960766574000189, 7.841185849078001091 ) ) ;
#65808=CARTESIAN_POINT ( 'NONE',  ( 9.922182479546000522, -3.489927462211000364, -9.111803974470001677 ) ) ;
#65810=PLANE ( 'NONE',  #13669 ) ;
#65812=CARTESIAN_POINT ( 'NONE',  ( 9.866664898013999263, -4.626219091573998909, -9.027249334595000008 ) ) ;
#65815=EDGE_CURVE ( 'NONE', #41592, #65121, #58071, .T. ) ;
#65820=CARTESIAN_POINT ( 'NONE',  ( 10.88463635395000040, -2.841787580345000119, 5.065370950741000300 ) ) ;
#65822=ORIENTED_EDGE ( 'NONE', *, *, #45006, .T. ) ;
#65824=CARTESIAN_POINT ( 'NONE',  ( 11.06924082387999952, -5.425685649895999774, 8.012912555523998392 ) ) ;
#65827=CARTESIAN_POINT ( 'NONE',  ( 9.944325809452999820, -5.443013936195000291, 7.367349259341000156 ) ) ;
#65836=LINE ( 'NONE', #55014, #33256 ) ;
#65866=CARTESIAN_POINT ( 'NONE',  ( 9.137549407199999862, -2.995696424181999884, 8.544763501938000161 ) ) ;
#65869=EDGE_LOOP ( 'NONE', ( #40805, #43947, #42830, #33870, #47564, #39463, #15290, #20224, #20884, #51273 ) ) ;
#65876=CARTESIAN_POINT ( 'NONE',  ( 10.38314899745999931, -5.167567567567999731, 6.822293592207000934 ) ) ;
#65880=CARTESIAN_POINT ( 'NONE',  ( 9.520528907821001141, -2.899999999999999911, 6.152188490330000370 ) ) ;
#65884=CARTESIAN_POINT ( 'NONE',  ( 10.86268281683999959, -5.065331559464999245, -5.170271095491000501 ) ) ;
#65899=CARTESIAN_POINT ( 'NONE',  ( 8.385058059625000837, -4.977917894183000236, 6.416767031887000705 ) ) ;
#65905=ADVANCED_FACE ( 'NONE', ( #50858 ), #67263, .T. ) ;
#65909=CARTESIAN_POINT ( 'NONE',  ( 10.32891357011178179, -2.649873868443101355, -7.263327745081085141 ) ) ;
#65912=CARTESIAN_POINT ( 'NONE',  ( 8.289120559623999185, -4.310353212080000773, 9.459493062793997709 ) ) ;
#65916=CARTESIAN_POINT ( 'NONE',  ( 7.915155411429996235, -5.089315853099998677, 6.494606418034001294 ) ) ;
#65918=EDGE_CURVE ( 'NONE', #53919, #63466, #42226, .T. ) ;
#65921=VERTEX_POINT ( 'NONE', #14488 ) ;
#65934=ORIENTED_EDGE ( 'NONE', *, *, #27387, .F. ) ;
#65935=DIRECTION ( 'NONE',  ( -0.9999999999996369571, -8.520359571663319094E-07, -4.194710005752155130E-09 ) ) ;
#65940=CARTESIAN_POINT ( 'NONE',  ( 7.683884986463000111, -9.053566239910001201, 5.593786582504999494 ) ) ;
#65944=CARTESIAN_POINT ( 'NONE',  ( 8.610875063856999745, -4.757997781751000410, 5.934102420827000124 ) ) ;
#65946=DIRECTION ( 'NONE',  ( 1.000000000000000000, 0.000000000000000000, 0.000000000000000000 ) ) ;
#65956=ADVANCED_FACE ( 'NONE', ( #66925 ), #27687, .F. ) ;
#65964=VERTEX_POINT ( 'NONE', #45194 ) ;
#65968=B_SPLINE_CURVE_WITH_KNOTS ( 'NONE', 3,
 ( #30746, #31780, #36681, #41918, #47168, #9752, #52752, #10101, #31436, #4847, #68471, #25151, #52406, #58002, #21279, #4499, #25497, #53098, #47862, #26191, #42275, #31100, #52055, #9069, #30407, #4159 ),
 .UNSPECIFIED., .F., .F.,
 ( 4, 2, 2, 2, 2, 2, 2, 2, 2, 1, 1, 2, 2, 4 ),
 ( 0.000000000000000000, 0.1000754736140108403, 0.2001509472280216806, 0.4003018944560433612, 0.4503396312630491560, 0.5003773680700549509, 0.6004528416840660965, 0.7005283152980773531, 0.7255471837015801118, 0.7380566179033314356, 0.7443113350042072085, 0.7474386935546450950, 0.7505660521050829814, 0.8006037889120940498 ),
 .UNSPECIFIED. ) ;
#65969=CARTESIAN_POINT ( 'NONE',  ( 10.82564972918999935, -5.331162346451000289, -8.542142527201001201 ) ) ;
#65974=CARTESIAN_POINT ( 'NONE',  ( 10.12821852033218128, -4.965567672101669494, -8.481131518971576355 ) ) ;
#65978=CARTESIAN_POINT ( 'NONE',  ( 10.84419170916408426, -2.685373094371525937, -7.853312882625532509 ) ) ;
#65979=CARTESIAN_POINT ( 'NONE',  ( 8.910378124222608776, -5.351542105685522799, 7.263808684111356939 ) ) ;
#65991=CARTESIAN_POINT ( 'NONE',  ( 8.052730646792999991, -4.968144979409999884, 5.971795951526999602 ) ) ;
#66004=ORIENTED_EDGE ( 'NONE', *, *, #21997, .T. ) ;
#66008=CARTESIAN_POINT ( 'NONE',  ( 9.611390067472999732, -3.334847606888000193, 5.869121315726000709 ) ) ;
#66013=CARTESIAN_POINT ( 'NONE',  ( 8.093556867701995117, -4.420942022140136984, 5.812522706633525438 ) ) ;
#66014=CARTESIAN_POINT ( 'NONE',  ( 10.28315099603999982, -2.387772357283999725, 7.684266429524000408 ) ) ;
#66015=CARTESIAN_POINT ( 'NONE',  ( 9.924988015501654104, -5.349815781278972615, 7.500001845592777272 ) ) ;
#66023=ORIENTED_EDGE ( 'NONE', *, *, #6857, .F. ) ;
#66035=CARTESIAN_POINT ( 'NONE',  ( 7.994581853207999522, -2.263562268490999951, 8.007440964304000985 ) ) ;
#66043=EDGE_CURVE ( 'NONE', #48366, #53120, #57640, .T. ) ;
#66048=AXIS2_PLACEMENT_3D ( 'NONE', #40954, #46203, #7762 ) ;
#66078=CARTESIAN_POINT ( 'NONE',  ( 10.71370252004577495, -5.723616352180168398, 7.813700803284126195 ) ) ;
#66079=CARTESIAN_POINT ( 'NONE',  ( 7.700043146791999860, -3.346260729029000291, 6.002247316312999459 ) ) ;
#66084=ORIENTED_EDGE ( 'NONE', *, *, #2401, .T. ) ;
#66100=CARTESIAN_POINT ( 'NONE',  ( 7.424920563404769247, -2.344203440956357909, 8.033218592177277628 ) ) ;
#66112=CARTESIAN_POINT ( 'NONE',  ( 10.98768472633000037, -5.449702618601000026, 4.945212061625999134 ) ) ;
#66126=DIRECTION ( 'NONE',  ( -0.1218403629891999795, 1.031102794712999922E-07, 0.9925497095595008368 ) ) ;
#66131=CARTESIAN_POINT ( 'NONE',  ( 9.988720925027999797, -2.842024021884000273, -6.504330542082999322 ) ) ;
#66134=ADVANCED_FACE ( 'NONE', ( #49140 ), #1251, .T. ) ;
#66135=CARTESIAN_POINT ( 'NONE',  ( 10.41272044195154223, -3.158844023651794952, -4.969917438239939145 ) ) ;
#66142=CARTESIAN_POINT ( 'NONE',  ( 10.81499708368651369, -2.650004840405617124, -7.499999822193714749 ) ) ;
#66145=CARTESIAN_POINT ( 'NONE',  ( 9.332935524889000689, -5.100347267927999972, 8.693464469215999912 ) ) ;
#66159=B_SPLINE_CURVE_WITH_KNOTS ( 'NONE', 3,
 ( #20030, #9877, #63000, #62333 ),
 .UNSPECIFIED., .F., .F.,
 ( 4, 4 ),
 ( 0.000000000000000000, 1.000000000000000000 ),
 .UNSPECIFIED. ) ;
#66160=CARTESIAN_POINT ( 'NONE',  ( 7.881386639450599141, -5.152558780658690551, 6.796436122627368626 ) ) ;
#66163=CARTESIAN_POINT ( 'NONE',  ( 9.705325322606999094, -5.130141620686999637, -6.219151643305999677 ) ) ;
#66169=CARTESIAN_POINT ( 'NONE',  ( 10.68683480410999920, -2.958852069189999767, 5.111032341795000100 ) ) ;
#66170=CARTESIAN_POINT ( 'NONE',  ( 0.000000000000000000, -2.899999999999999911, -7.500000000000000000 ) ) ;
#66173=CARTESIAN_POINT ( 'NONE',  ( 9.124702828701000357, -4.778665285493000070, 8.799745834808000211 ) ) ;
#66176=CARTESIAN_POINT ( 'NONE',  ( 10.77962878203999963, -2.397503436487000261, 7.755423856053000442 ) ) ;
#66177=ADVANCED_FACE ( 'NONE', ( #28167 ), #25398, .F. ) ;
#66178=CARTESIAN_POINT ( 'NONE',  ( 9.808181774614295634, -4.356028300593894897, 9.240976368499895344 ) ) ;
#66185=DIRECTION ( 'NONE',  ( 0.000000000000000000, -1.000000000000000000, 0.000000000000000000 ) ) ;
#66188=CARTESIAN_POINT ( 'NONE',  ( 9.529318513071000751, -2.297586052318000061, -7.360088033824999876 ) ) ;
#66191=CARTESIAN_POINT ( 'NONE',  ( 9.924988015501654104, -5.349815781278972615, 7.500001845592777272 ) ) ;
#66209=EDGE_LOOP ( 'NONE', ( #17423, #4303, #58844, #9714, #3340 ) ) ;
#66210=CARTESIAN_POINT ( 'NONE',  ( 9.571967469951999874, -4.084684048989999816, 8.946621592834999248 ) ) ;
#66227=CARTESIAN_POINT ( 'NONE',  ( 9.354551302391419298, -3.358410772673184219, 9.116760870204894118 ) ) ;
#66230=VECTOR ( 'NONE', #21321, 1000.000000000000000 ) ;
#66233=CARTESIAN_POINT ( 'NONE',  ( 11.05073074817000034, -5.235671266423000070, -5.012833499169000007 ) ) ;
#66238=CARTESIAN_POINT ( 'NONE',  ( 10.84168850528999961, -2.681008214828000114, 6.554752254946000889 ) ) ;
#66247=CARTESIAN_POINT ( 'NONE',  ( 7.962144353208000069, -4.874569256861000177, 6.119503992241999590 ) ) ;
#66250=CARTESIAN_POINT ( 'NONE',  ( 11.12439163055999991, -5.544976217683999842, 5.163701761329000384 ) ) ;
#66255=CARTESIAN_POINT ( 'NONE',  ( 11.03298400728999873, -2.754860951861000107, -5.027234841342000493 ) ) ;
#66260=CARTESIAN_POINT ( 'NONE',  ( 9.123558059623999128, -5.558929022707999046, 6.272984818914999927 ) ) ;
#66271=CARTESIAN_POINT ( 'NONE',  ( 7.806992724014596874, -3.016426643082999792, 6.525734047976322394 ) ) ;
#66272=CARTESIAN_POINT ( 'NONE',  ( 11.04230989604436530, -2.757690103955632743, 6.361542621298440281 ) ) ;
#66283=ORIENTED_EDGE ( 'NONE', *, *, #35752, .T. ) ;
#66284=CARTESIAN_POINT ( 'NONE',  ( 9.517712236484261012, -4.527663441039016412, 8.747762430587503246 ) ) ;
#66288=CARTESIAN_POINT ( 'NONE',  ( 7.643638571636000023, -9.072798860549999844, 5.701353631702000158 ) ) ;
#66293=EDGE_LOOP ( 'NONE', ( #25711, #24539, #22735 ) ) ;
#66301=ORIENTED_EDGE ( 'NONE', *, *, #39099, .F. ) ;
#66302=CARTESIAN_POINT ( 'NONE',  ( 10.51293113580700123, -5.100000000000000533, 6.444141223116233164 ) ) ;
#66304=CARTESIAN_POINT ( 'NONE',  ( 10.93870578215442713, -2.832454552556203708, -6.732216691000727060 ) ) ;
#66310=ORIENTED_EDGE ( 'NONE', *, *, #49735, .F. ) ;
#66315=B_SPLINE_CURVE_WITH_KNOTS ( 'NONE', 3,
 ( #34821, #44968, #66272, #13157 ),
 .UNSPECIFIED., .F., .F.,
 ( 4, 4 ),
 ( 0.000000000000000000, 1.000000000000000000 ),
 .UNSPECIFIED. ) ;
#66318=CARTESIAN_POINT ( 'NONE',  ( 10.02800210979000184, -3.452027005875999865, -6.074520565702999697 ) ) ;
#66320=DIRECTION ( 'NONE',  ( -0.7071067811865150432, -0.1740570546198035029, -0.6853496492573148968 ) ) ;
#66321=CARTESIAN_POINT ( 'NONE',  ( 10.34271159708237242, -5.100000000000000533, -6.305985890001590377 ) ) ;
#66325=CARTESIAN_POINT ( 'NONE',  ( 10.63590686542660890, -5.314851119339436103, -7.853271763851031650 ) ) ;
#66337=CARTESIAN_POINT ( 'NONE',  ( 7.539230646792000279, -4.696237245142999228, 5.830277424166999900 ) ) ;
#66340=DIRECTION ( 'NONE',  ( 0.000000000000000000, 0.8648648648648720183, 0.5020047465136825426 ) ) ;
#66341=VERTEX_POINT ( 'NONE', #18714 ) ;
#66349=EDGE_LOOP ( 'NONE', ( #2955, #65320, #48934, #44948 ) ) ;
#66353=CARTESIAN_POINT ( 'NONE',  ( 9.393246442089999704, -5.100000000000000533, -6.421387671005999387 ) ) ;
#66355=CARTESIAN_POINT ( 'NONE',  ( 9.465112865370999273, -2.290047720994000002, 6.601709978349000529 ) ) ;
#66357=EDGE_LOOP ( 'NONE', ( #23143, #21548, #50962, #67666 ) ) ;
#66359=CARTESIAN_POINT ( 'NONE',  ( 10.69015444038000062, -4.391267940138999570, -8.802346922965000431 ) ) ;
#66360=CARTESIAN_POINT ( 'NONE',  ( 7.915661401038873279, -2.416848911730535399, 8.220850438606255750 ) ) ;
#66361=CARTESIAN_POINT ( 'NONE',  ( 11.02786767503999954, -5.596230239120999705, 7.209501483790000442 ) ) ;
#66370=CARTESIAN_POINT ( 'NONE',  ( 10.00107860442999907, -4.626219091573998909, -9.027249334595000008 ) ) ;
#66381=ADVANCED_FACE ( 'NONE', ( #37190 ), #36500, .F. ) ;
#66383=CARTESIAN_POINT ( 'NONE',  ( 9.112168146794999757, -2.368260286481999710, 7.410200011629000549 ) ) ;
#66389=CARTESIAN_POINT ( 'NONE',  ( 10.64557055961999943, -2.988935764546999607, -5.952339209104000162 ) ) ;
#66401=LINE ( 'NONE', #60131, #32778 ) ;
#66404=ADVANCED_FACE ( 'NONE', ( #473 ), #32554, .F. ) ;
#66411=ORIENTED_EDGE ( 'NONE', *, *, #59364, .T. ) ;
#66425=CARTESIAN_POINT ( 'NONE',  ( 10.79668711518602464, -4.601537912553735232, 9.136927527625404721 ) ) ;
#66426=CARTESIAN_POINT ( 'NONE',  ( 8.020980646792999380, -3.245532552444000185, 8.949627348471000943 ) ) ;
#66430=ORIENTED_EDGE ( 'NONE', *, *, #29372, .F. ) ;
#66452=CARTESIAN_POINT ( 'NONE',  ( 10.65165493200484370, -5.052088798245987000, 5.056974862721875574 ) ) ;
#66457=CARTESIAN_POINT ( 'NONE',  ( 10.84160444037999937, -2.641264320582999758, -7.444904971031999885 ) ) ;
#66465=ORIENTED_EDGE ( 'NONE', *, *, #58412, .F. ) ;
#66483=CARTESIAN_POINT ( 'NONE',  ( 10.76290585702731661, -2.920651757519954650, -8.329491109684262540 ) ) ;
#66486=CARTESIAN_POINT ( 'NONE',  ( 10.48164908029000131, -4.022873587130999518, 9.090901241422999490 ) ) ;
#66488=EDGE_CURVE ( 'NONE', #36042, #16713, #40471, .T. ) ;
#66498=AXIS2_PLACEMENT_3D ( 'NONE', #40076, #18401, #10607 ) ;
#66499=CARTESIAN_POINT ( 'NONE',  ( 6.799999999999999822, -10.75000000000000000, 0.000000000000000000 ) ) ;
#66504=CARTESIAN_POINT ( 'NONE',  ( 9.661323620223001285, -4.289037785427000316, -5.816478295321999781 ) ) ;
#66510=CARTESIAN_POINT ( 'NONE',  ( 10.42861967375000098, -2.931274166824000105, 4.618461898129999632 ) ) ;
#66514=CARTESIAN_POINT ( 'NONE',  ( 11.08992739829000129, -5.210546653347999602, 8.327600405525998895 ) ) ;
#66532=CARTESIAN_POINT ( 'NONE',  ( 9.265308298767999773, -5.700621988293000264, -7.339579610785999186 ) ) ;
#66543=VERTEX_POINT ( 'NONE', #23177 ) ;
#66560=VERTEX_POINT ( 'NONE', #17244 ) ;
#66566=ADVANCED_FACE ( 'NONE', ( #38565 ), #19662, .T. ) ;
#66572=CARTESIAN_POINT ( 'NONE',  ( 9.382584444952824398, -2.847231605938053356, 8.802921338423775666 ) ) ;
#66576=DIRECTION ( 'NONE',  ( 1.000000000000000000, 0.000000000000000000, 0.000000000000000000 ) ) ;
#66579=B_SPLINE_CURVE_WITH_KNOTS ( 'NONE', 3,
 ( #4012, #29938, #68678, #51242 ),
 .UNSPECIFIED., .F., .F.,
 ( 4, 4 ),
 ( 0.000000000000000000, 1.000000000000000000 ),
 .UNSPECIFIED. ) ;
#66580=CARTESIAN_POINT ( 'NONE',  ( 9.939319226872999735, -2.638101016021999978, 6.328632621050000573 ) ) ;
#66589=DIRECTION ( 'NONE',  ( 0.000000000000000000, 0.000000000000000000, 1.000000000000000000 ) ) ;
#66594=CARTESIAN_POINT ( 'NONE',  ( 10.97044361512000066, -6.153378486422999671, 5.035908310043000213 ) ) ;
#66595=CARTESIAN_POINT ( 'NONE',  ( 8.888847637062996299, -5.105690627519996028, -6.405231889100001297 ) ) ;
#66598=FACE_OUTER_BOUND ( 'NONE', #29087, .T. ) ;
#66607=EDGE_CURVE ( 'NONE', #52724, #5164, #12129, .T. ) ;
#66610=CARTESIAN_POINT ( 'NONE',  ( 8.186778834302003816, -5.111320685747004156, 6.695945149192998436 ) ) ;
#66629=VECTOR ( 'NONE', #7570, 1000.000000000000000 ) ;
#66631=ORIENTED_EDGE ( 'NONE', *, *, #21052, .T. ) ;
#66634=CARTESIAN_POINT ( 'NONE',  ( 8.470293146793999028, -4.255646685191999623, 9.114089645792999406 ) ) ;
#66638=CARTESIAN_POINT ( 'NONE',  ( 9.051363484269000281, -8.680251604461998838, 6.293370873935000276 ) ) ;
#66639=FACE_OUTER_BOUND ( 'NONE', #69065, .T. ) ;
#66644=CARTESIAN_POINT ( 'NONE',  ( 9.843726350706999639, -4.115123626494000320, 9.466607949400000166 ) ) ;
#66651=CARTESIAN_POINT ( 'NONE',  ( 10.40685100253999984, -2.832432432432000269, -6.822293592207000934 ) ) ;
#66655=CARTESIAN_POINT ( 'NONE',  ( 9.020964430773000586, -2.907392932634000005, 6.146188468825999784 ) ) ;
#66665=CARTESIAN_POINT ( 'NONE',  ( 10.47211906628000122, -2.640759929160000130, -8.505246563374999624 ) ) ;
#66667=CARTESIAN_POINT ( 'NONE',  ( 9.028522009144964500, -5.063507634687575809, 8.333874286671722587 ) ) ;
#66671=CARTESIAN_POINT ( 'NONE',  ( 10.86501009699205866, -2.649983380499685737, -7.500000587580680111 ) ) ;
#66684=CARTESIAN_POINT ( 'NONE',  ( 7.603418146792000343, -5.687202994508999687, 6.847270485579000088 ) ) ;
#66699=CARTESIAN_POINT ( 'NONE',  ( 9.253736882039186540, -4.918551780227518933, -6.034027795051781773 ) ) ;
#66701=CARTESIAN_POINT ( 'NONE',  ( 9.966331042021000286, -2.304002513595999613, 6.575636708208000059 ) ) ;
#66704=DIRECTION ( 'NONE',  ( -6.273181842718999770E-11, -6.273118898148000207E-11, -1.000000000000000000 ) ) ;
#66707=CARTESIAN_POINT ( 'NONE',  ( 7.983375487919488478, -2.407341777098653157, 6.779802702655946867 ) ) ;
#66708=CARTESIAN_POINT ( 'NONE',  ( 11.05639424537999993, -5.030223832177999732, 6.028291574375000295 ) ) ;
#66712=CARTESIAN_POINT ( 'NONE',  ( 10.74001548714999998, -5.126947719599001196, -5.008168344353999935 ) ) ;
#66713=B_SPLINE_CURVE_WITH_KNOTS ( 'NONE', 3,
 ( #38756, #44007, #16044, #53795 ),
 .UNSPECIFIED., .F., .F.,
 ( 4, 4 ),
 ( 0.000000000000000000, 1.000000000000000000 ),
 .UNSPECIFIED. ) ;
#66719=CARTESIAN_POINT ( 'NONE',  ( 9.487725409950000355, -4.905858243509999106, -8.948175900338000588 ) ) ;
#66721=CARTESIAN_POINT ( 'NONE',  ( 9.472537864290000442, -2.899999999999999911, -6.571291218949999902 ) ) ;
#66729=CARTESIAN_POINT ( 'NONE',  ( 9.304730646793998972, -5.284133759825000887, 6.489273023403000273 ) ) ;
#66731=VERTEX_POINT ( 'NONE', #4595 ) ;
#66734=CARTESIAN_POINT ( 'NONE',  ( 10.13035685320999946, -2.409329538444999752, -8.058042649154000259 ) ) ;
#66775=CARTESIAN_POINT ( 'NONE',  ( 10.82122311210984478, -4.081721762518836449, 9.237771506523644760 ) ) ;
#66776=CARTESIAN_POINT ( 'NONE',  ( 7.598066940377999678, -3.554853390786000045, 8.889491623367000273 ) ) ;
#66790=CARTESIAN_POINT ( 'NONE',  ( 10.02314899745999988, -5.167567567567999731, -6.822293592207000934 ) ) ;
#66792=CARTESIAN_POINT ( 'NONE',  ( 9.362879440377000151, -3.677416446733000388, 9.250734868033999803 ) ) ;
#66793=VERTEX_POINT ( 'NONE', #14759 ) ;
#66797=AXIS2_PLACEMENT_3D ( 'NONE', #25346, #67988, #62740 ) ;
#66798=CARTESIAN_POINT ( 'NONE',  ( 10.62120626704272475, -3.646797508062162851, 8.848526273074867277 ) ) ;
#66803=CARTESIAN_POINT ( 'NONE',  ( 10.96219100130544710, -4.057262373299075797, -9.264968071217497325 ) ) ;
#66808=DIRECTION ( 'NONE',  ( -1.000000000000000000, 0.000000000000000000, 0.000000000000000000 ) ) ;
#66824=CARTESIAN_POINT ( 'NONE',  ( 10.20319453770999907, -3.421758889707999796, 6.017729046583999875 ) ) ;
#66828=CARTESIAN_POINT ( 'NONE',  ( 10.72510394928771227, -2.650147065043205519, 7.500007457243348163 ) ) ;
#66837=CARTESIAN_POINT ( 'NONE',  ( 9.757667269575000191, -4.489271889653999814, 5.986031004145000445 ) ) ;
#66851=CARTESIAN_POINT ( 'NONE',  ( 9.441315108303999892, -3.111669560323000017, -8.958991988670002016 ) ) ;
#66863=CARTESIAN_POINT ( 'NONE',  ( 10.22109127278999807, -2.983266195621000261, 8.764707262515999631 ) ) ;
#66865=CARTESIAN_POINT ( 'NONE',  ( 10.90000000000000036, -2.778483479159999714, -6.925197956411000000 ) ) ;
#66874=CARTESIAN_POINT ( 'NONE',  ( 11.13109956191000016, -2.679615677191000245, 4.997638975407999951 ) ) ;
#66878=CARTESIAN_POINT ( 'NONE',  ( 9.702742433789000032, -5.491975933468000726, -7.893788029530999673 ) ) ;
#66915=CARTESIAN_POINT ( 'NONE',  ( 9.409553643212783314, -2.475290888679036794, 8.337164624878596442 ) ) ;
#66916=ORIENTED_EDGE ( 'NONE', *, *, #38538, .F. ) ;
#66919=FACE_OUTER_BOUND ( 'NONE', #52738, .T. ) ;
#66923=CARTESIAN_POINT ( 'NONE',  ( 10.65550933554000146, -4.237674644795000667, 9.105223721671999115 ) ) ;
#66925=FACE_OUTER_BOUND ( 'NONE', #34933, .T. ) ;
#66939=CARTESIAN_POINT ( 'NONE',  ( 10.74718774421000056, -2.737610732962999727, 4.827894279797999566 ) ) ;
#66940=CARTESIAN_POINT ( 'NONE',  ( 10.77666960233000104, -2.704364821029999977, -4.799376923177000265 ) ) ;
#66941=CARTESIAN_POINT ( 'NONE',  ( 9.416972128128000108, -4.783349162191000481, -6.231236652334000148 ) ) ;
#66946=CARTESIAN_POINT ( 'NONE',  ( 11.13494815609000099, -5.334103115335000034, 5.185088833845999723 ) ) ;
#66950=CARTESIAN_POINT ( 'NONE',  ( 8.189586429382003985, -5.107684026525003418, 6.413118510302999731 ) ) ;
#66958=CARTESIAN_POINT ( 'NONE',  ( 11.05853765099000086, -8.013864593771998557, -6.925175679306001086 ) ) ;
#66970=CARTESIAN_POINT ( 'NONE',  ( 9.667080975990000269, -4.541622198376999542, 5.824041840233000755 ) ) ;
#66973=CARTESIAN_POINT ( 'NONE',  ( 9.395316940379000670, -5.146736128384000075, 6.597417125647000447 ) ) ;
#66978=CARTESIAN_POINT ( 'NONE',  ( 7.924878289113923557, -5.349357204871147076, 7.500005630225521358 ) ) ;
#66982=CARTESIAN_POINT ( 'NONE',  ( 9.781666627457001439, -5.464740618746000145, 8.817321229216000589 ) ) ;
#66993=CARTESIAN_POINT ( 'NONE',  ( 7.925196951433999715, -5.124045536972000825, 6.724518905982000305 ) ) ;
#66998=ORIENTED_EDGE ( 'NONE', *, *, #63982, .T. ) ;
#67003=AXIS2_PLACEMENT_3D ( 'NONE', #47907, #3, #62258 ) ;
#67007=CARTESIAN_POINT ( 'NONE',  ( 10.11858840337999865, -3.393395892949000014, -5.921999462319999630 ) ) ;
#67009=CARTESIAN_POINT ( 'NONE',  ( 9.593325696102663613, -2.223596456112051811, -7.416212298303232586 ) ) ;
#67013=CARTESIAN_POINT ( 'NONE',  ( 10.81294898260481041, -2.920599542025066331, -8.329474447052662711 ) ) ;
#67015=CARTESIAN_POINT ( 'NONE',  ( 7.000000000000000000, -6.255435840762999966, -3.000000000000000000 ) ) ;
#67017=DIRECTION ( 'NONE',  ( 0.000000000000000000, 1.000000000000000000, 0.000000000000000000 ) ) ;
#67027=CARTESIAN_POINT ( 'NONE',  ( 7.165495559622000243, -2.688354259407999880, 8.140021027181001401 ) ) ;
#67042=CARTESIAN_POINT ( 'NONE',  ( 10.24478558459999888, -5.265199116477000452, 8.959495174640998982 ) ) ;
#67046=CARTESIAN_POINT ( 'NONE',  ( 11.29595444038000096, -2.828863075736999910, -8.191124550002999882 ) ) ;
#67048=CARTESIAN_POINT ( 'NONE',  ( 7.938552267647699168, -2.277490889987867639, 7.743639942309443747 ) ) ;
#67049=CARTESIAN_POINT ( 'NONE',  ( 10.43579701286999928, -2.587605342384000195, 6.390039770907999461 ) ) ;
#67058=CARTESIAN_POINT ( 'NONE',  ( 9.531727112333999941, -4.010297355695000121, -9.208122400763999238 ) ) ;
#67067=CARTESIAN_POINT ( 'NONE',  ( 8.764831853209999579, -5.808258301303999893, 7.446016267012000256 ) ) ;
#67072=CARTESIAN_POINT ( 'NONE',  ( 10.77401935321000082, -3.826867196099999813, -5.823197386290999589 ) ) ;
#67084=B_SPLINE_CURVE_WITH_KNOTS ( 'NONE', 3,
 ( #8407, #55956, #40226, #35328, #51397, #24487 ),
 .UNSPECIFIED., .F., .F.,
 ( 4, 2, 4 ),
 ( 0.000000000000000000, 0.5000000000000000000, 1.000000000000000000 ),
 .UNSPECIFIED. ) ;
#67093=B_SPLINE_CURVE_WITH_KNOTS ( 'NONE', 3,
 ( #48842, #42905, #948, #43601 ),
 .UNSPECIFIED., .F., .F.,
 ( 4, 4 ),
 ( 0.000000000000000000, 1.000000000000000000 ),
 .UNSPECIFIED. ) ;
#67108=ORIENTED_EDGE ( 'NONE', *, *, #52390, .F. ) ;
#67111=CARTESIAN_POINT ( 'NONE',  ( 10.77788359937968998, -4.967860659007850899, 8.954442448909505359 ) ) ;
#67112=CARTESIAN_POINT ( 'NONE',  ( 7.983191940377000861, -5.321924421352999701, 8.118250081378000971 ) ) ;
#67113=DIRECTION ( 'NONE',  ( 0.000000000000000000, 0.000000000000000000, -1.000000000000000000 ) ) ;
#67121=DIRECTION ( 'NONE',  ( 0.000000000000000000, 1.000000000000000000, 0.000000000000000000 ) ) ;
#67126=CARTESIAN_POINT ( 'NONE',  ( 8.309480646794000336, -2.905864338704999827, 8.940687151810998046 ) ) ;
#67127=ORIENTED_EDGE ( 'NONE', *, *, #39979, .T. ) ;
#67130=CARTESIAN_POINT ( 'NONE',  ( 7.340118112958106344, -3.660443313038189928, 9.214377072997308460 ) ) ;
#67131=CARTESIAN_POINT ( 'NONE',  ( 10.70440763477068558, -2.684940916868676641, 7.852706794445921901 ) ) ;
#67136=CARTESIAN_POINT ( 'NONE',  ( 10.92087510617160540, -4.925384977304763545, -9.003857666150715033 ) ) ;
#67141=CARTESIAN_POINT ( 'NONE',  ( 10.06949314679000018, -4.910373174915999783, -8.649593977693999847 ) ) ;
#67150=ORIENTED_EDGE ( 'NONE', *, *, #11731, .F. ) ;
#67154=AXIS2_PLACEMENT_3D ( 'NONE', #47395, #31316, #67325 ) ;
#67158=CARTESIAN_POINT ( 'NONE',  ( 11.29621718459000057, -3.561654022787999807, 6.266039799355000106 ) ) ;
#67160=CARTESIAN_POINT ( 'NONE',  ( 10.56270535986999981, -2.509383044034000143, -8.602408326857998944 ) ) ;
#67163=FACE_BOUND ( 'NONE', #5061, .T. ) ;
#67165=EDGE_LOOP ( 'NONE', ( #57634, #31362, #61916, #38477, #32105 ) ) ;
#67166=CARTESIAN_POINT ( 'NONE',  ( 10.96256888877000080, -6.761399355091999297, -5.456120342596999073 ) ) ;
#67172=CARTESIAN_POINT ( 'NONE',  ( 10.30047649312000146, -4.027768368024999823, 9.431342508940000258 ) ) ;
#67173=VERTEX_POINT ( 'NONE', #57973 ) ;
#67182=B_SPLINE_CURVE_WITH_KNOTS ( 'NONE', 3,
 ( #23976, #2647, #55797, #59999 ),
 .UNSPECIFIED., .F., .F.,
 ( 4, 4 ),
 ( 0.000000000000000000, 1.000000000000000000 ),
 .UNSPECIFIED. ) ;
#67196=ORIENTED_EDGE ( 'NONE', *, *, #26833, .F. ) ;
#67197=AXIS2_PLACEMENT_3D ( 'NONE', #41998, #5273, #53171 ) ;
#67200=CARTESIAN_POINT ( 'NONE',  ( 10.18755811987000115, -5.387486580809999204, 8.640943191857999750 ) ) ;
#67203=CARTESIAN_POINT ( 'NONE',  ( 10.87522165821000009, -4.831071966430999787, 6.312786525516999703 ) ) ;
#67213=PLANE ( 'NONE',  #13872 ) ;
#67214=EDGE_CURVE ( 'NONE', #14991, #59582, #49821, .T. ) ;
#67217=CARTESIAN_POINT ( 'NONE',  ( 9.881332132140999036, -4.333399685216000385, -9.088699530815999239 ) ) ;
#67226=DIRECTION ( 'NONE',  ( 0.000000000000000000, 0.7071067811865474617, -0.7071067811865474617 ) ) ;
#67253=CARTESIAN_POINT ( 'NONE',  ( 9.370475807310532090, -3.052722418981052233, 8.962984445555635560 ) ) ;
#67257=CARTESIAN_POINT ( 'NONE',  ( 11.13092457518000167, -5.324127713801000361, -5.001427652733999807 ) ) ;
#67263=PLANE ( 'NONE',  #67618 ) ;
#67264=EDGE_LOOP ( 'NONE', ( #48171, #40918, #24422, #58003 ) ) ;
#67268=CARTESIAN_POINT ( 'NONE',  ( 8.266851002545999805, -2.832432432432000269, 6.822293592207000934 ) ) ;
#67275=CARTESIAN_POINT ( 'NONE',  ( 8.755241167949000314, -5.090758519327002851, -6.463251571066001233 ) ) ;
#67278=CARTESIAN_POINT ( 'NONE',  ( 10.27381073070999840, -3.247454413448000121, 4.596980832202000045 ) ) ;
#67280=CARTESIAN_POINT ( 'NONE',  ( 9.575728814717999526, -3.111669560323000017, -8.958991988670002016 ) ) ;
#67284=CARTESIAN_POINT ( 'NONE',  ( 10.88763167770999907, -5.057180698083000969, 5.046290572389999340 ) ) ;
#67287=CONICAL_SURFACE ( 'NONE', #3655, 10.65000803020999953, 0.7853981633972997312 ) ;
#67307=VERTEX_POINT ( 'NONE', #60384 ) ;
#67308=CARTESIAN_POINT ( 'NONE',  ( 9.980430903642000473, -4.047223565251000466, 9.090364706348999846 ) ) ;
#67309=ORIENTED_EDGE ( 'NONE', *, *, #27491, .T. ) ;
#67310=CARTESIAN_POINT ( 'NONE',  ( 8.498279931254906217, -3.130208739192112954, 6.060545171114974927 ) ) ;
#67311=CARTESIAN_POINT ( 'NONE',  ( 9.138566940380000503, -2.933824946949000090, 8.496487880080000110 ) ) ;
#67317=LINE ( 'NONE', #34507, #20815 ) ;
#67320=CARTESIAN_POINT ( 'NONE',  ( 11.02286109245999945, -2.398753588646000079, 6.352476128646999065 ) ) ;
#67323=CARTESIAN_POINT ( 'NONE',  ( 10.61721988130000049, -5.045606037229999785, -6.386907901056999570 ) ) ;
#67325=DIRECTION ( 'NONE',  ( 0.000000000000000000, -1.000000000000000000, 0.000000000000000000 ) ) ;
#67330=CARTESIAN_POINT ( 'NONE',  ( 10.08422653160753413, -2.899999999999999911, 6.304440313740826696 ) ) ;
#67334=VERTEX_POINT ( 'NONE', #65617 ) ;
#67341=CARTESIAN_POINT ( 'NONE',  ( 9.947300131853999972, -4.892806669161000599, -9.067746434455999704 ) ) ;
#67362=CARTESIAN_POINT ( 'NONE',  ( 7.769581853207999877, -2.431397064767999439, 7.958394431095000776 ) ) ;
#67367=ORIENTED_EDGE ( 'NONE', *, *, #65918, .T. ) ;
#67368=VECTOR ( 'NONE', #54558, 1000.000000000000114 ) ;
#67375=FACE_OUTER_BOUND ( 'NONE', #58129, .T. ) ;
#67378=CARTESIAN_POINT ( 'NONE',  ( 7.949305362820807019, -5.068892134240547520, 6.584878031929767950 ) ) ;
#67379=CARTESIAN_POINT ( 'NONE',  ( 11.09999999999999964, -5.299524241844999928, -5.124965750789000296 ) ) ;
#67383=EDGE_CURVE ( 'NONE', #27255, #49898, #37867, .T. ) ;
#67385=CARTESIAN_POINT ( 'NONE',  ( 8.222974175369182959, -5.661925504349325955, 8.013205229805864249 ) ) ;
#67388=ORIENTED_EDGE ( 'NONE', *, *, #8830, .T. ) ;
#67389=CARTESIAN_POINT ( 'NONE',  ( 11.07586359541999954, -5.334319426963999078, -4.951757428735000133 ) ) ;
#67391=VERTEX_POINT ( 'NONE', #56403 ) ;
#67393=VECTOR ( 'NONE', #63463, 1000.000000000000000 ) ;
#67395=CARTESIAN_POINT ( 'NONE',  ( 9.326385834542001874, -4.867164667115999599, -6.095483598963999938 ) ) ;
#67405=CARTESIAN_POINT ( 'NONE',  ( 7.673644353206999114, -4.696237245142999228, 5.830277424166999900 ) ) ;
#67410=CARTESIAN_POINT ( 'NONE',  ( 10.52384314678999999, -5.441919393629000012, -7.989634081859001036 ) ) ;
#67420=VERTEX_POINT ( 'NONE', #51493 ) ;
#67421=CARTESIAN_POINT ( 'NONE',  ( 10.26575685213000000, -4.574972855646000092, 4.689163863504999696 ) ) ;
#67450=CARTESIAN_POINT ( 'NONE',  ( 8.983793146794999629, -3.979464503892999439, 9.134080454305001595 ) ) ;
#67463=CARTESIAN_POINT ( 'NONE',  ( 11.09806944063053891, -2.697063473153181068, 6.634103937395076755 ) ) ;
#67464=CARTESIAN_POINT ( 'NONE',  ( 8.335879440378999305, -4.310353212080000773, 9.459493062793997709 ) ) ;
#67465=ORIENTED_EDGE ( 'NONE', *, *, #33931, .F. ) ;
#67473=CARTESIAN_POINT ( 'NONE',  ( 7.643806538548957974, -5.335784186437363630, 6.386268904257039303 ) ) ;
#67475=CARTESIAN_POINT ( 'NONE',  ( 7.702547272646715015, -2.712723599019214671, 7.026494385502345175 ) ) ;
#67489=AXIS2_PLACEMENT_3D ( 'NONE', #32257, #37147, #5661 ) ;
#67490=ORIENTED_EDGE ( 'NONE', *, *, #64563, .F. ) ;
#67501=B_SPLINE_CURVE_WITH_KNOTS ( 'NONE', 3,
 ( #39026, #40064, #34479, #23285 ),
 .UNSPECIFIED., .F., .F.,
 ( 4, 4 ),
 ( 0.000000000000000000, 1.000000000000000000 ),
 .UNSPECIFIED. ) ;
#67504=CARTESIAN_POINT ( 'NONE',  ( 10.62792628238999981, -3.100579357212000176, 8.599905962393000536 ) ) ;
#67506=CARTESIAN_POINT ( 'NONE',  ( 10.44486180556999955, -4.964082081645000422, -9.083599939499999110 ) ) ;
#67509=ORIENTED_EDGE ( 'NONE', *, *, #49731, .T. ) ;
#67516=CARTESIAN_POINT ( 'NONE',  ( 11.05935368890999904, -2.480241580537000168, 6.610077204591000566 ) ) ;
#67523=CYLINDRICAL_SURFACE ( 'NONE', #9523, 0.5000000000000000000 ) ;
#67542=CARTESIAN_POINT ( 'NONE',  ( 10.62698276521000196, -3.142914536759000121, 8.668455626664998803 ) ) ;
#67549=EDGE_CURVE ( 'NONE', #39743, #37501, #15338, .T. ) ;
#67550=EDGE_CURVE ( 'NONE', #20205, #8257, #48659, .T. ) ;
#67552=CARTESIAN_POINT ( 'NONE',  ( 10.64264450635444703, -5.032314077581211187, -5.044903346590539073 ) ) ;
#67558=CARTESIAN_POINT ( 'NONE',  ( 9.399896294736999280, -5.679455740088000582, -8.329752476417999318 ) ) ;
#67560=CARTESIAN_POINT ( 'NONE',  ( 9.496378438922418397, -5.350075508921414702, 7.852928877054440093 ) ) ;
#67569=CARTESIAN_POINT ( 'NONE',  ( 8.653803059789179741, -2.648172424375523804, 7.852957271307993814 ) ) ;
#67572=EDGE_CURVE ( 'NONE', #67420, #15904, #21058, .T. ) ;
#67588=ORIENTED_EDGE ( 'NONE', *, *, #870, .F. ) ;
#67602=B_SPLINE_CURVE_WITH_KNOTS ( 'NONE', 3,
 ( #22942, #59664, #65593, #56054 ),
 .UNSPECIFIED., .F., .F.,
 ( 4, 4 ),
 ( 0.000000000000000000, 1.000000000000000000 ),
 .UNSPECIFIED. ) ;
#67605=ORIENTED_EDGE ( 'NONE', *, *, #61872, .F. ) ;
#67608=CARTESIAN_POINT ( 'NONE',  ( 7.371537754583582291, -4.354055095920205787, 6.184131058409644943 ) ) ;
#67614=CARTESIAN_POINT ( 'NONE',  ( 8.908101985566998948, -4.557680047860001693, -6.178109778951999864 ) ) ;
#67618=AXIS2_PLACEMENT_3D ( 'NONE', #2953, #45619, #19379 ) ;
#67620=CARTESIAN_POINT ( 'NONE',  ( 9.622313405920001728, -4.009302068291999532, -9.043024413115999138 ) ) ;
#67623=CARTESIAN_POINT ( 'NONE',  ( 10.98768521492000083, -5.299565686336999981, -4.945211137252000455 ) ) ;
#67630=EDGE_CURVE ( 'NONE', #13225, #49271, #31552, .T. ) ;
#67641=DIRECTION ( 'NONE',  ( 1.000000000000000000, 0.000000000000000000, 0.000000000000000000 ) ) ;
#67646=ORIENTED_EDGE ( 'NONE', *, *, #67549, .T. ) ;
#67647=CARTESIAN_POINT ( 'NONE',  ( 10.98286725694000054, -3.998514182530999772, 9.091066422484001208 ) ) ;
#67650=CARTESIAN_POINT ( 'NONE',  ( 7.622413825165171630, -2.920663668686906522, 8.329223781267950599 ) ) ;
#67651=CARTESIAN_POINT ( 'NONE',  ( 8.239941940377999430, -2.735207418315000361, 6.771977475428999860 ) ) ;
#67659=ORIENTED_EDGE ( 'NONE', *, *, #46092, .T. ) ;
#67663=VERTEX_POINT ( 'NONE', #53559 ) ;
#67666=ORIENTED_EDGE ( 'NONE', *, *, #40728, .T. ) ;
#67675=CARTESIAN_POINT ( 'NONE',  ( 7.895317210312003731, -5.140737874544996977, 6.778394131643998399 ) ) ;
#67685=CARTESIAN_POINT ( 'NONE',  ( 9.004748037742926314, -5.259886971390435484, 7.984416769088259258 ) ) ;
#67693=CARTESIAN_POINT ( 'NONE',  ( 8.207504440379000954, -5.944572422272999646, 7.106845737860000511 ) ) ;
#67704=CARTESIAN_POINT ( 'NONE',  ( 7.149102686541000118, -4.351670788182000038, 8.977200644264000218 ) ) ;
#67725=CARTESIAN_POINT ( 'NONE',  ( 8.258127245199675670, -5.292721928877631044, 8.664547103137167028 ) ) ;
#67729=CARTESIAN_POINT ( 'NONE',  ( 10.60379983616000032, -5.060307628864999963, -4.956681627023000303 ) ) ;
#67731=ORIENTED_EDGE ( 'NONE', *, *, #22465, .T. ) ;
#67736=CARTESIAN_POINT ( 'NONE',  ( 10.90000000000000036, -1.300000000000000044, 9.662944685757000940 ) ) ;
#67742=VERTEX_POINT ( 'NONE', #61139 ) ;
#67744=CARTESIAN_POINT ( 'NONE',  ( 9.294724726289000927, -4.148132978932999926, 9.337467253566000380 ) ) ;
#67745=CARTESIAN_POINT ( 'NONE',  ( 11.09999999999999964, -5.299316147296000423, 5.124965750789000296 ) ) ;
#67749=CARTESIAN_POINT ( 'NONE',  ( 11.16750564679000135, -3.188702545307000147, -8.788667016604001958 ) ) ;
#67758=ORIENTED_EDGE ( 'NONE', *, *, #42574, .F. ) ;
#67771=ADVANCED_FACE ( 'NONE', ( #3426 ), #58924, .F. ) ;
#67773=CARTESIAN_POINT ( 'NONE',  ( 8.716296636326459790, -4.700163249105822949, -6.344245921207472882 ) ) ;
#67784=B_SPLINE_CURVE_WITH_KNOTS ( 'NONE', 3,
 ( #36892, #63441, #11680, #16239, #26747 ),
 .UNSPECIFIED., .F., .F.,
 ( 4, 1, 4 ),
 ( 0.000000000000000000, 0.5000000000000000000, 1.000000000000000000 ),
 .UNSPECIFIED. ) ;
#67791=VERTEX_POINT ( 'NONE', #9351 ) ;
#67801=CARTESIAN_POINT ( 'NONE',  ( 10.13804496475983186, -5.254201105732013488, 6.278396282701761422 ) ) ;
#67809=CARTESIAN_POINT ( 'NONE',  ( 8.400066940379998570, -2.800111029801999774, 9.079936276749000612 ) ) ;
#67813=CARTESIAN_POINT ( 'NONE',  ( 10.79702055961999818, -5.792859009854000263, -7.049265738992000152 ) ) ;
#67814=CARTESIAN_POINT ( 'NONE',  ( 7.577752120373228095, -4.080750291709096089, 5.762678877088324825 ) ) ;
#67821=CARTESIAN_POINT ( 'NONE',  ( 10.90710314112699564, -5.175205309304410584, -8.818007615062088078 ) ) ;
#67823=ADVANCED_FACE ( 'NONE', ( #5149 ), #30694, .F. ) ;
#67826=B_SPLINE_CURVE_WITH_KNOTS ( 'NONE', 3,
 ( #49437, #12387, #55038, #12737, #24252, #65513, #50479, #34418, #17641, #7836, #7478, #34757, #44902, #35104 ),
 .UNSPECIFIED., .F., .F.,
 ( 4, 2, 2, 2, 2, 2, 4 ),
 ( 0.000000000000000000, 0.2500000000000002220, 0.3749999999999998890, 0.4999999999999995559, 0.6249999999999992228, 0.7499999999999988898, 1.000000000000000000 ),
 .UNSPECIFIED. ) ;
#67836=ORIENTED_EDGE ( 'NONE', *, *, #46405, .T. ) ;
#67837=CARTESIAN_POINT ( 'NONE',  ( 8.616332388160998335, -5.167567399848000065, -6.822293593032000558 ) ) ;
#67845=CARTESIAN_POINT ( 'NONE',  ( 9.590594544025000445, -2.445960766574000189, 7.841185849078001091 ) ) ;
#67850=FACE_OUTER_BOUND ( 'NONE', #23217, .T. ) ;
#67852=CARTESIAN_POINT ( 'NONE',  ( 10.96873203361999849, -5.814970961921999582, -4.932337198421000046 ) ) ;
#67858=CARTESIAN_POINT ( 'NONE',  ( 11.02445830383999947, -3.404091099119999519, 5.822494319281999786 ) ) ;
#67865=VERTEX_POINT ( 'NONE', #25443 ) ;
#67877=CARTESIAN_POINT ( 'NONE',  ( 9.309310001151999359, -5.531435376468999188, -8.256621485025000595 ) ) ;
#67897=ORIENTED_EDGE ( 'NONE', *, *, #12080, .F. ) ;
#67901=CARTESIAN_POINT ( 'NONE',  ( 10.36409410702807143, -4.658690586846539361, -4.954046122677381980 ) ) ;
#67907=CARTESIAN_POINT ( 'NONE',  ( 11.09999999999999964, -4.000000000000000000, -7.500000000000000000 ) ) ;
#67908=CARTESIAN_POINT ( 'NONE',  ( 10.00190805961999807, -2.729654112791000120, -8.843024969850999284 ) ) ;
#67909=EDGE_CURVE ( 'NONE', #33561, #65121, #20411, .T. ) ;
#67914=FACE_OUTER_BOUND ( 'NONE', #27004, .T. ) ;
#67918=CARTESIAN_POINT ( 'NONE',  ( 8.466090690305595245, -5.179931350395992062, 8.180989497825457590 ) ) ;
#67923=CARTESIAN_POINT ( 'NONE',  ( 11.09999999999999964, -4.000000000000000000, 7.500000000000000000 ) ) ;
#67941=CARTESIAN_POINT ( 'NONE',  ( 27.64127793187000037, -5.599999999999999645, 6.571291218949999902 ) ) ;
#67945=VERTEX_POINT ( 'NONE', #21912 ) ;
#67948=CIRCLE ( 'NONE', #13286, 1.250000000000000000 ) ;
#67953=CARTESIAN_POINT ( 'NONE',  ( 9.753033816428001046, -4.922930220739999641, -8.639537379291999386 ) ) ;
#67954=ORIENTED_EDGE ( 'NONE', *, *, #24704, .F. ) ;
#67965=CARTESIAN_POINT ( 'NONE',  ( 9.041579158320997678, -5.131952024793004163, -6.343693428288000646 ) ) ;
#67967=EDGE_CURVE ( 'NONE', #51438, #55718, #26247, .T. ) ;
#67969=CARTESIAN_POINT ( 'NONE',  ( 10.34549887484000052, -3.253839642723999948, -4.718279307348000273 ) ) ;
#67973=FACE_OUTER_BOUND ( 'NONE', #35425, .T. ) ;
#67985=CARTESIAN_POINT ( 'NONE',  ( 11.09999999999999964, 0.000000000000000000, -2.784439345760000141E-13 ) ) ;
#67988=DIRECTION ( 'NONE',  ( -0.8660254037844296038, 7.899625398266597896E-12, 0.5000000000000157652 ) ) ;
#67996=CARTESIAN_POINT ( 'NONE',  ( 11.03855816545999957, -2.974093234901999949, 8.716125417860000724 ) ) ;
#67998=CARTESIAN_POINT ( 'NONE',  ( 9.225036374688860619, -2.649952446100997339, 7.500002253091946791 ) ) ;
#67999=CARTESIAN_POINT ( 'NONE',  ( 9.331129440379999807, -4.141908960411000429, 6.047561724438000219 ) ) ;
#68006=DIRECTION ( 'NONE',  ( -9.754664239791915610E-08, 0.7071067475397934121, -0.7071068148332932957 ) ) ;
#68007=CARTESIAN_POINT ( 'NONE',  ( 10.21613001987144465, -2.826347940569525097, 6.832757752125532491 ) ) ;
#68013=CARTESIAN_POINT ( 'NONE',  ( 9.741009892375998902, -3.588529236307000048, -8.800227248412999970 ) ) ;
#68014=CARTESIAN_POINT ( 'NONE',  ( 10.81772273141334750, -5.100000000000000533, -6.253511885790826952 ) ) ;
#68015=ORIENTED_EDGE ( 'NONE', *, *, #58981, .F. ) ;
#68024=ORIENTED_EDGE ( 'NONE', *, *, #11203, .T. ) ;
#68032=EDGE_CURVE ( 'NONE', #36772, #31317, #67093, .T. ) ;
#68034=CARTESIAN_POINT ( 'NONE',  ( 10.52342417510000061, -3.209670667763000029, -9.177087527572998837 ) ) ;
#68036=CARTESIAN_POINT ( 'NONE',  ( 8.975133088423635996, -5.349981448246158955, 7.499992563499107590 ) ) ;
#68042=AXIS2_PLACEMENT_3D ( 'NONE', #67907, #47631, #20364 ) ;
#68046=ADVANCED_FACE ( 'NONE', ( #6872 ), #22076, .F. ) ;
#68054=CARTESIAN_POINT ( 'NONE',  ( 8.732394353210001015, -2.806079842068999852, 8.615883328687999665 ) ) ;
#68056=CARTESIAN_POINT ( 'NONE',  ( 7.811250121011001468, -4.190252858842606010, 6.133645552891420216 ) ) ;
#68065=CARTESIAN_POINT ( 'NONE',  ( 10.74600376124999990, -5.242711034443999552, 8.978690688221998784 ) ) ;
#68068=CARTESIAN_POINT ( 'NONE',  ( 7.861428251418627333, -5.109570395020106126, 6.686999168342897981 ) ) ;
#68070=CARTESIAN_POINT ( 'NONE',  ( 8.214066216216412641, -5.709958105020243480, 7.828137529621371549 ) ) ;
#68081=CARTESIAN_POINT ( 'NONE',  ( 10.61171207387999971, -2.821101057508000221, -4.761811341319999613 ) ) ;
#68088=VECTOR ( 'NONE', #4117, 1000.000000000000000 ) ;
#68090=CARTESIAN_POINT ( 'NONE',  ( 8.481683059623998489, -2.472358291268000219, 6.234202627038999189 ) ) ;
#68093=B_SPLINE_SURFACE_WITH_KNOTS ( 'NONE', 3, 3, ( 
 ( #19373, #24279, #2606, #56091 ),
 ( #13115, #34444, #50167, #65884 ),
 ( #49816, #51199, #35126, #44928 ),
 ( #18012, #50506, #61341, #61679 ),
 ( #67257, #66233, #39329, #34091 ) ),
 .UNSPECIFIED., .F., .F., .F.,
 ( 4, 1, 4 ),
 ( 4, 4 ),
 ( -0.006081020443020000374, 0.000000000000000000, 0.03678947617080999960 ),
 ( -0.1730217193418999988, 1.173021718456999984 ),
 .UNSPECIFIED. ) ;
#68096=CARTESIAN_POINT ( 'NONE',  ( 11.00119435320999983, -4.640445114785999969, -9.059317673956000405 ) ) ;
#68117=ORIENTED_EDGE ( 'NONE', *, *, #18312, .T. ) ;
#68118=CARTESIAN_POINT ( 'NONE',  ( 8.767881343006999728, -4.605543323398999966, -6.293427432547999523 ) ) ;
#68139=AXIS2_PLACEMENT_3D ( 'NONE', #37457, #26975, #44099 ) ;
#68148=ORIENTED_EDGE ( 'NONE', *, *, #17808, .T. ) ;
#68152=CARTESIAN_POINT ( 'NONE',  ( 8.721004440379999778, -5.983034890242000081, 7.440798487724999966 ) ) ;
#68154=CARTESIAN_POINT ( 'NONE',  ( 9.646790723601728956, -5.267286625425933622, -8.036436072827047639 ) ) ;
#68156=CARTESIAN_POINT ( 'NONE',  ( 11.02419555961999897, -2.407899345275000158, -8.439548421502999886 ) ) ;
#68157=CARTESIAN_POINT ( 'NONE',  ( 7.479299064383798878, -2.376666221062909035, 6.873252664167585735 ) ) ;
#68160=ORIENTED_EDGE ( 'NONE', *, *, #29507, .T. ) ;
#68175=CYLINDRICAL_SURFACE ( 'NONE', #26062, 2.000000000000001332 ) ;
#68186=CARTESIAN_POINT ( 'NONE',  ( 9.576494682405000347, -4.593972507100000158, 5.662052676321000177 ) ) ;
#68197=CARTESIAN_POINT ( 'NONE',  ( 10.85738557828999973, -2.754556666341999804, 8.976367391363998749 ) ) ;
#68200=VERTEX_POINT ( 'NONE', #17282 ) ;
#68203=CARTESIAN_POINT ( 'NONE',  ( 10.55991645936999923, -5.094263939633999705, 6.075409946530999861 ) ) ;
#68208=LINE ( 'NONE', #46906, #45482 ) ;
#68210=EDGE_CURVE ( 'NONE', #66543, #2854, #32000, .T. ) ;
#68212=CARTESIAN_POINT ( 'NONE',  ( 9.353311703536000721, -4.905858243509999106, -8.948175900338000588 ) ) ;
#68239=CARTESIAN_POINT ( 'NONE',  ( 11.04420485398999929, -2.755310155137999484, 5.177028922958999857 ) ) ;
#68243=CARTESIAN_POINT ( 'NONE',  ( 9.355894592352999695, -5.864995026133001055, -7.324074232821000230 ) ) ;
#68244=CARTESIAN_POINT ( 'NONE',  ( 10.22908305962000064, -4.838492992840000007, -5.852445959518000507 ) ) ;
#68247=CARTESIAN_POINT ( 'NONE',  ( 10.95037914754042419, -5.141203310087995249, -5.102208348236233704 ) ) ;
#68248=ADVANCED_FACE ( 'NONE', ( #49096 ), #33373, .T. ) ;
#68255=ORIENTED_EDGE ( 'NONE', *, *, #21052, .F. ) ;
#68256=CARTESIAN_POINT ( 'NONE',  ( -15.86200481174999943, -2.399999999999999911, 6.571291218949999902 ) ) ;
#68263=DIRECTION ( 'NONE',  ( 0.000000000000000000, 1.000000000000000000, 0.000000000000000000 ) ) ;
#68267=( BOUNDED_CURVE ( )  B_SPLINE_CURVE ( 3, ( #5048, #52600, #48049, #57494, #9602, #30944, #52261 ),
 .UNSPECIFIED., .F., .T. ) 
 B_SPLINE_CURVE_WITH_KNOTS ( ( 4, 1, 1, 1, 4 ),
 ( 0.000000000000000000, 0.1584901274852722752, 0.4217256158758324047, 0.6948883626783448619, 1.000000000000000000 ),
 .UNSPECIFIED. ) 
 CURVE ( )  GEOMETRIC_REPRESENTATION_ITEM ( )  RATIONAL_B_SPLINE_CURVE ( ( 1.171572587279782862, 1.171572587279782862, 1.171572587279782862, 1.171572587279782862, 1.171572587279782862, 1.171572587279782862, 1.171572587279782862 ) ) 
 REPRESENTATION_ITEM ( '' )  );
#68284=CARTESIAN_POINT ( 'NONE',  ( 11.07184579812000003, -5.268087732220000596, -5.079906681876000363 ) ) ;
#68289=CARTESIAN_POINT ( 'NONE',  ( 9.701728707608999969, -4.253751259212999791, -8.839942087209999855 ) ) ;
#68290=ORIENTED_EDGE ( 'NONE', *, *, #8279, .F. ) ;
#68300=CARTESIAN_POINT ( 'NONE',  ( 7.883148997456999929, -5.167567567567999731, 6.822293592207000934 ) ) ;
#68301=CARTESIAN_POINT ( 'NONE',  ( 7.426677373658002956, -3.232655724474999381, 6.473459691208998557 ) ) ;
#68302=ORIENTED_EDGE ( 'NONE', *, *, #26833, .T. ) ;
#68309=CARTESIAN_POINT ( 'NONE',  ( 9.856463691916330205, -5.100000000000000533, 6.665341197412375962 ) ) ;
#68312=CARTESIAN_POINT ( 'NONE',  ( 7.612571400991003046, -4.588494467460999537, 6.486759529251004075 ) ) ;
#68314=CARTESIAN_POINT ( 'NONE',  ( 10.87668353155522638, -2.650012393097451291, -7.302148410131374945 ) ) ;
#68318=ORIENTED_EDGE ( 'NONE', *, *, #23600, .F. ) ;
#68334=CARTESIAN_POINT ( 'NONE',  ( 10.39106278671000005, -4.025320977579999848, 9.261121875182000807 ) ) ;
#68335=ORIENTED_EDGE ( 'NONE', *, *, #10835, .T. ) ;
#68337=CARTESIAN_POINT ( 'NONE',  ( 8.893206853209999707, -3.977267280662000193, 9.308921106447000327 ) ) ;
#68344=LINE ( 'NONE', #42824, #40931 ) ;
#68347=CARTESIAN_POINT ( 'NONE',  ( 10.31167756636999933, -2.874479384703000129, 8.900026329558999194 ) ) ;
#68353=CARTESIAN_POINT ( 'NONE',  ( 10.90000000000000036, -5.100000000000000533, -6.436740704805999691 ) ) ;
#68364=CARTESIAN_POINT ( 'NONE',  ( 10.01532628870999986, -4.946995631616999844, 8.559221361189001342 ) ) ;
#68366=CARTESIAN_POINT ( 'NONE',  ( 7.780759508074995168, -4.599947829706001912, 6.384407252255998699 ) ) ;
#68369=CARTESIAN_POINT ( 'NONE',  ( 10.99845801742999996, -5.289427263538000190, 4.962451247354000117 ) ) ;
#68375=ORIENTED_EDGE ( 'NONE', *, *, #68827, .F. ) ;
#68380=CARTESIAN_POINT ( 'NONE',  ( 7.320269353207000229, -2.466384407480000096, 6.935560677555000275 ) ) ;
#68383=VECTOR ( 'NONE', #57849, 1000.000000000000000 ) ;
#68392=CARTESIAN_POINT ( 'NONE',  ( 8.989144353209001181, -5.284133759825000887, 6.489273023403000273 ) ) ;
#68399=ORIENTED_EDGE ( 'NONE', *, *, #14023, .F. ) ;
#68403=CARTESIAN_POINT ( 'NONE',  ( 10.52324012719000024, -3.325647021086999722, 5.689999163383999026 ) ) ;
#68410=CARTESIAN_POINT ( 'NONE',  ( 8.287884602529770106, -4.765396756871579598, 9.061745085214184314 ) ) ;
#68418=CYLINDRICAL_SURFACE ( 'NONE', #12266, 1.250000000000000000 ) ;
#68422=CARTESIAN_POINT ( 'NONE',  ( 9.402304893999998470, -4.531444417037000072, -6.133284059228000018 ) ) ;
#68423=CARTESIAN_POINT ( 'NONE',  ( 10.42499241036559532, -5.349775919985432004, 7.500001834605715345 ) ) ;
#68426=CARTESIAN_POINT ( 'NONE',  ( 8.666985328329976923, -5.621196112576180681, 6.797938611047623425 ) ) ;
#68436=EDGE_CURVE ( 'NONE', #2498, #19018, #67826, .T. ) ;
#68440=CARTESIAN_POINT ( 'NONE',  ( 11.09999999999999964, -5.350000000000000533, 7.500000000000000000 ) ) ;
#68446=VERTEX_POINT ( 'NONE', #33721 ) ;
#68450=CARTESIAN_POINT ( 'NONE',  ( 10.84088306584999906, -2.636277440143000472, -7.512643837511999934 ) ) ;
#68455=CARTESIAN_POINT ( 'NONE',  ( 8.686257345956043707, -4.773936950834467119, -6.393475887002888491 ) ) ;
#68471=CARTESIAN_POINT ( 'NONE',  ( 9.169137439642966569, -2.970390391148245435, 8.373688857599031365 ) ) ;
#68475=CARTESIAN_POINT ( 'NONE',  ( 10.97892463630881110, -2.365042658448092361, 6.878289458889421226 ) ) ;
#68479=ORIENTED_EDGE ( 'NONE', *, *, #13361, .T. ) ;
#68487=DIRECTION ( 'NONE',  ( 0.000000000000000000, 0.000000000000000000, -1.000000000000000000 ) ) ;
#68488=ORIENTED_EDGE ( 'NONE', *, *, #64295, .F. ) ;
#68493=CARTESIAN_POINT ( 'NONE',  ( 7.897956853208000005, -3.608524635952000459, 5.913372239166000632 ) ) ;
#68497=CARTESIAN_POINT ( 'NONE',  ( 10.18367854428777974, -2.796579479970164872, 8.204151721975753375 ) ) ;
#68498=CARTESIAN_POINT ( 'NONE',  ( 10.19122055961999962, -3.990707710465999813, -5.651373900265999950 ) ) ;
#68499=CARTESIAN_POINT ( 'NONE',  ( 7.507604010646850234, -2.694814696844040736, 6.316660876498477073 ) ) ;
#68502=ORIENTED_EDGE ( 'NONE', *, *, #66607, .F. ) ;
#68512=VECTOR ( 'NONE', #51209, 1000.000000000000000 ) ;
#68528=CARTESIAN_POINT ( 'NONE',  ( 10.30047649312000146, -4.027768368024999823, 9.431342508940000258 ) ) ;
#68541=CARTESIAN_POINT ( 'NONE',  ( 10.96876739532000045, -2.333349849211999949, 6.524062020538999640 ) ) ;
#68549=CARTESIAN_POINT ( 'NONE',  ( 9.600494040286998043, -5.206548117663999165, 8.585114612872999373 ) ) ;
#68557=CARTESIAN_POINT ( 'NONE',  ( 9.221306596384000187, -5.362859773739999447, -6.470306978669999154 ) ) ;
#68570=CARTESIAN_POINT ( 'NONE',  ( 10.81316193496000011, -3.756072284922999938, 6.071597915422999314 ) ) ;
#68580=CARTESIAN_POINT ( 'NONE',  ( 10.98768577056000062, -2.700436730051000378, -4.945210085382000464 ) ) ;
#68584=AXIS2_PLACEMENT_3D ( 'NONE', #3675, #8938, #9967 ) ;
#68617=AXIS2_PLACEMENT_3D ( 'NONE', #56636, #62217, #67113 ) ;
#68623=CARTESIAN_POINT ( 'NONE',  ( 9.610944094206999466, -5.100000000000000533, -6.571291218949999902 ) ) ;
#68626=CARTESIAN_POINT ( 'NONE',  ( 8.969027209994999694, -8.708546445325000107, -6.388758794122999518 ) ) ;
#68630=CARTESIAN_POINT ( 'NONE',  ( 8.440795537699431250, -5.100000000000000533, 6.662590550605512973 ) ) ;
#68634=CARTESIAN_POINT ( 'NONE',  ( 10.01597818573999987, -4.792673671522000411, -6.390249203106999509 ) ) ;
#68636=ORIENTED_EDGE ( 'NONE', *, *, #68436, .T. ) ;
#68641=EDGE_CURVE ( 'NONE', #9679, #65751, #42822, .T. ) ;
#68652=CARTESIAN_POINT ( 'NONE',  ( 10.35355256951999969, -3.429327234421000181, -4.862083573089999611 ) ) ;
#68655=CARTESIAN_POINT ( 'NONE',  ( 10.74609562913000005, -4.263104965433000437, 9.276976808608999647 ) ) ;
#68657=CARTESIAN_POINT ( 'NONE',  ( 10.66052890781999984, -2.899999999999999911, -6.152188490330000370 ) ) ;
#68658=EDGE_CURVE ( 'NONE', #49429, #1971, #60284, .T. ) ;
#68678=CARTESIAN_POINT ( 'NONE',  ( 9.568197172114265570, -5.125396288426561142, -6.749639981083131346 ) ) ;
#68682=CARTESIAN_POINT ( 'NONE',  ( 9.889844610056000462, -4.052276314598000084, 9.260527932809999641 ) ) ;
#68684=CARTESIAN_POINT ( 'NONE',  ( 9.441293086742424734, -5.329066508289010962, 7.778880124525636930 ) ) ;
#68685=CARTESIAN_POINT ( 'NONE',  ( 7.647245559622000144, -5.850279024084999335, 6.784181137144999596 ) ) ;
#68687=EDGE_CURVE ( 'NONE', #37266, #2854, #51971, .T. ) ;
#68696=ORIENTED_EDGE ( 'NONE', *, *, #52985, .T. ) ;
#68697=CARTESIAN_POINT ( 'NONE',  ( 10.06343867337000120, -5.156226070197000411, 6.125223053176999777 ) ) ;
#68701=CARTESIAN_POINT ( 'NONE',  ( 10.99385884816394388, -6.143977714627776976, -5.074464171073912233 ) ) ;
#68705=CARTESIAN_POINT ( 'NONE',  ( 8.745593092018999926, -5.100000000000000533, 6.404090157675000228 ) ) ;
#68706=CARTESIAN_POINT ( 'NONE',  ( 5.000000000000000000, -0.2999999999999999889, 11.34603454956999791 ) ) ;
#68721=CARTESIAN_POINT ( 'NONE',  ( 9.543013888829964486, -2.517265190286118948, -8.482290249887922684 ) ) ;
#68729=CARTESIAN_POINT ( 'NONE',  ( 7.924355646793000751, -2.432121990576000314, 6.597519606637999523 ) ) ;
#68741=CARTESIAN_POINT ( 'NONE',  ( 8.508081853209001011, -2.202816532622999812, 7.706987678916999762 ) ) ;
#68744=EDGE_CURVE ( 'NONE', #42399, #21322, #28745, .T. ) ;
#68754=CARTESIAN_POINT ( 'NONE',  ( 10.96876739532000045, -2.333349849211999949, 6.524062020538999640 ) ) ;
#68759=CARTESIAN_POINT ( 'NONE',  ( 8.288478674082428554, -4.754023060363307351, 9.067272220935310045 ) ) ;
#68761=ORIENTED_EDGE ( 'NONE', *, *, #38171, .F. ) ;
#68773=ADVANCED_FACE ( 'NONE', ( #55303 ), #12306, .F. ) ;
#68782=B_SPLINE_CURVE_WITH_KNOTS ( 'NONE', 3,
 ( #50121, #54669, #44199, #7459 ),
 .UNSPECIFIED., .F., .F.,
 ( 4, 4 ),
 ( 0.000000000000000000, 1.000000000000000000 ),
 .UNSPECIFIED. ) ;
#68783=CARTESIAN_POINT ( 'NONE',  ( 7.647245559622000144, -5.850279024084999335, 6.784181137144999596 ) ) ;
#68784=CARTESIAN_POINT ( 'NONE',  ( 11.07232916052000071, -5.267955070953999730, 5.080680273674000880 ) ) ;
#68823=DIRECTION ( 'NONE',  ( -1.000000000000000000, 0.000000000000000000, 0.000000000000000000 ) ) ;
#68826=DIRECTION ( 'NONE',  ( 0.000000000000000000, 0.3146293386371170064, -0.9492146118074512584 ) ) ;
#68827=EDGE_CURVE ( 'NONE', #31041, #51438, #45309, .T. ) ;
#68830=VERTEX_POINT ( 'NONE', #47910 ) ;
#68843=FACE_OUTER_BOUND ( 'NONE', #59703, .T. ) ;
#68844=CARTESIAN_POINT ( 'NONE',  ( 9.160311019873999427, -4.122021308488999836, 9.013573548576999883 ) ) ;
#68845=EDGE_LOOP ( 'NONE', ( #36689, #5561, #38758, #42911, #21624, #32088, #49010, #5390, #14573, #49968 ) ) ;
#68849=CARTESIAN_POINT ( 'NONE',  ( 7.611539800697518565, -4.772443708916318528, 5.941223257842239036 ) ) ;
#68858=DIRECTION ( 'NONE',  ( 0.7660444431251208774, 4.730414054088128888E-08, 0.6427876096792169980 ) ) ;
#68861=B_SPLINE_CURVE_WITH_KNOTS ( 'NONE', 3,
 ( #62329, #67560, #20366, #14783, #20711, #46255, #36102, #14444, #30185, #51492 ),
 .UNSPECIFIED., .F., .F.,
 ( 4, 2, 2, 2, 4 ),
 ( 0.1254132184345819190, 0.3127269071678268619, 0.5000405959010718604, 0.6873542846343168033, 0.8746679733675617463 ),
 .UNSPECIFIED. ) ;
#68878=CARTESIAN_POINT ( 'NONE',  ( 9.632185590920999019, -5.638162562978999759, 6.476633609657000079 ) ) ;
#68888=CARTESIAN_POINT ( 'NONE',  ( 11.09999999999999964, -2.700000000000000178, -5.157071250680000496 ) ) ;
#68901=CARTESIAN_POINT ( 'NONE',  ( 9.075489683949001574, -4.020837068201999820, 8.948702918089999514 ) ) ;
#68918=B_SPLINE_CURVE_WITH_KNOTS ( 'NONE', 3,
 ( #54747, #35412, #6846, #28181, #24221, #65574, #17697, #8492, #39021, #60339 ),
 .UNSPECIFIED., .F., .F.,
 ( 4, 2, 2, 2, 4 ),
 ( 0.000000000000000000, 0.1968496138483742108, 0.3936992276967484217, 0.5905488415451226603, 0.7873984553934968433 ),
 .UNSPECIFIED. ) ;
#68920=EDGE_CURVE ( 'NONE', #2068, #38985, #42658, .T. ) ;
#68923=CARTESIAN_POINT ( 'NONE',  ( 10.37874387220000116, -4.882732524430000609, 6.350796477317000921 ) ) ;
#68926=VECTOR ( 'NONE', #2025, 1000.000000000000114 ) ;
#68945=CARTESIAN_POINT ( 'NONE',  ( 7.924878289113923557, -5.349357204871147076, 7.500005630225521358 ) ) ;
#68949=ORIENTED_EDGE ( 'NONE', *, *, #56776, .F. ) ;
#68961=CARTESIAN_POINT ( 'NONE',  ( 9.317462135714000837, -5.100000000000000533, 6.571291218949999902 ) ) ;
#68969=EDGE_LOOP ( 'NONE', ( #21102, #16320, #46612, #23131, #64009, #64666, #48662 ) ) ;
#68985=EDGE_CURVE ( 'NONE', #11689, #59582, #22702, .T. ) ;
#68988=CARTESIAN_POINT ( 'NONE',  ( 9.858853446676000942, -2.668079545448999834, -7.206971019603000350 ) ) ;
#68990=VERTEX_POINT ( 'NONE', #23405 ) ;
#69000=CARTESIAN_POINT ( 'NONE',  ( 8.493436541922999794, -2.902501512378997894, 6.607638123744003167 ) ) ;
#69001=ORIENTED_EDGE ( 'NONE', *, *, #68744, .T. ) ;
#69003=ADVANCED_FACE ( 'NONE', ( #23744 ), #34964, .F. ) ;
#69004=CARTESIAN_POINT ( 'NONE',  ( 8.030239402831002238, -2.905307396403002507, 6.399703979581998325 ) ) ;
#69006=DIRECTION ( 'NONE',  ( 1.000000000000000000, 0.000000000000000000, 0.000000000000000000 ) ) ;
#69007=CARTESIAN_POINT ( 'NONE',  ( 9.347248564704999652, -4.028326926800000152, 9.469437404464001062 ) ) ;
#69016=CARTESIAN_POINT ( 'NONE',  ( 7.760743125788000185, -3.157312404059000155, 6.445099350801999805 ) ) ;
#69021=CARTESIAN_POINT ( 'NONE',  ( 11.09999999999999964, -4.000000000000000000, -7.500000000000000000 ) ) ;
#69025=VERTEX_POINT ( 'NONE', #32353 ) ;
#69035=CARTESIAN_POINT ( 'NONE',  ( 9.854949224988001077, -2.800315695760000168, 9.013807298610000629 ) ) ;
#69037=ORIENTED_EDGE ( 'NONE', *, *, #64955, .F. ) ;
#69039=CARTESIAN_POINT ( 'NONE',  ( 9.112168146794999757, -2.368260286481999710, 7.410200011629000549 ) ) ;
#69043=ORIENTED_EDGE ( 'NONE', *, *, #3351, .F. ) ;
#69044=CARTESIAN_POINT ( 'NONE',  ( 27.64127793187000037, -5.599999999999999645, 6.571291218949999902 ) ) ;
#69051=CARTESIAN_POINT ( 'NONE',  ( 10.46933016578999975, -4.988498232033999891, 6.213103211926000569 ) ) ;
#69059=CARTESIAN_POINT ( 'NONE',  ( 9.842836772853271299, -2.713977296312396259, -7.027125797468761981 ) ) ;
#69065=EDGE_LOOP ( 'NONE', ( #31110, #82, #59515, #3450, #42928 ) ) ;
#69066=CARTESIAN_POINT ( 'NONE',  ( 8.500365452454994752, -5.097361224984004124, 6.605627025648004746 ) ) ;
#69067=ORIENTED_EDGE ( 'NONE', *, *, #37865, .F. ) ;
#69072=LINE ( 'NONE', #63471, #60527 ) ;
#69074=CIRCLE ( 'NONE', #34466, 1.350000000000000311 ) ;
#69076=EDGE_LOOP ( 'NONE', ( #13513, #19380, #45037, #10713, #36548, #48681, #52969, #10379, #36641, #22274 ) ) ;
#69082=CARTESIAN_POINT ( 'NONE',  ( 8.116918146793999256, -5.773185758034999893, 7.141496747382000798 ) ) ;
#69086=CARTESIAN_POINT ( 'NONE',  ( 10.65293113562639959, -5.100000000000000533, -6.444141223575878819 ) ) ;
#69095=CARTESIAN_POINT ( 'NONE',  ( 8.470293146793999028, -4.255646685191999623, 9.114089645792999406 ) ) ;
#69106=CARTESIAN_POINT ( 'NONE',  ( 9.218291396515251535, -5.004075074800184986, -6.183516294244955525 ) ) ;
#69113=CARTESIAN_POINT ( 'NONE',  ( 8.539901661839698122, -3.276467725318618296, 5.918453690889198704 ) ) ;
#69114=CARTESIAN_POINT ( 'NONE',  ( 10.96954340945999995, -8.070525344816001478, 6.995684484348000609 ) ) ;
#69121=CARTESIAN_POINT ( 'NONE',  ( 7.861016604981150735, -4.181402732447497606, 6.140015153376770840 ) ) ;
#69127=CARTESIAN_POINT ( 'NONE',  ( 8.877678275024724286, -2.921484010191843339, 8.876657601656255281 ) ) ;
#69128=EDGE_CURVE ( 'NONE', #1971, #62373, #12401, .T. ) ;
#69135=CARTESIAN_POINT ( 'NONE',  ( 7.283516392955999841, -4.426925773067000414, 9.293310812901001583 ) ) ;
#69147=FACE_OUTER_BOUND ( 'NONE', #37256, .T. ) ;
#69149=EDGE_CURVE ( 'NONE', #18837, #518, #52720, .T. ) ;
#69155=CARTESIAN_POINT ( 'NONE',  ( 8.787837227906001303, -4.603772362336000512, -6.276682186892999837 ) ) ;
#69159=CARTESIAN_POINT ( 'NONE',  ( 10.48496058254999852, -5.061587542142000018, -4.699980696949000780 ) ) ;
#69171=DIRECTION ( 'NONE',  ( 0.000000000000000000, 1.000000000000000000, 0.000000000000000000 ) ) ;
#69177=ORIENTED_EDGE ( 'NONE', *, *, #68641, .T. ) ;
#69187=CARTESIAN_POINT ( 'NONE',  ( 10.53733998880999856, -2.992814141720000265, 8.731692578598000409 ) ) ;
#69188=CARTESIAN_POINT ( 'NONE',  ( 7.807370559623000084, -3.650411072918999800, 6.083135626079000602 ) ) ;
#69189=ORIENTED_EDGE ( 'NONE', *, *, #57128, .T. ) ;
#69194=CARTESIAN_POINT ( 'NONE',  ( 7.742012705865137789, -5.501263588994199871, 8.379108557587658268 ) ) ;
#69195=CARTESIAN_POINT ( 'NONE',  ( 11.09999999999999964, -0.5000000000000000000, 5.124965750789000296 ) ) ;
ENDSEC;
END-ISO-10303-21;
